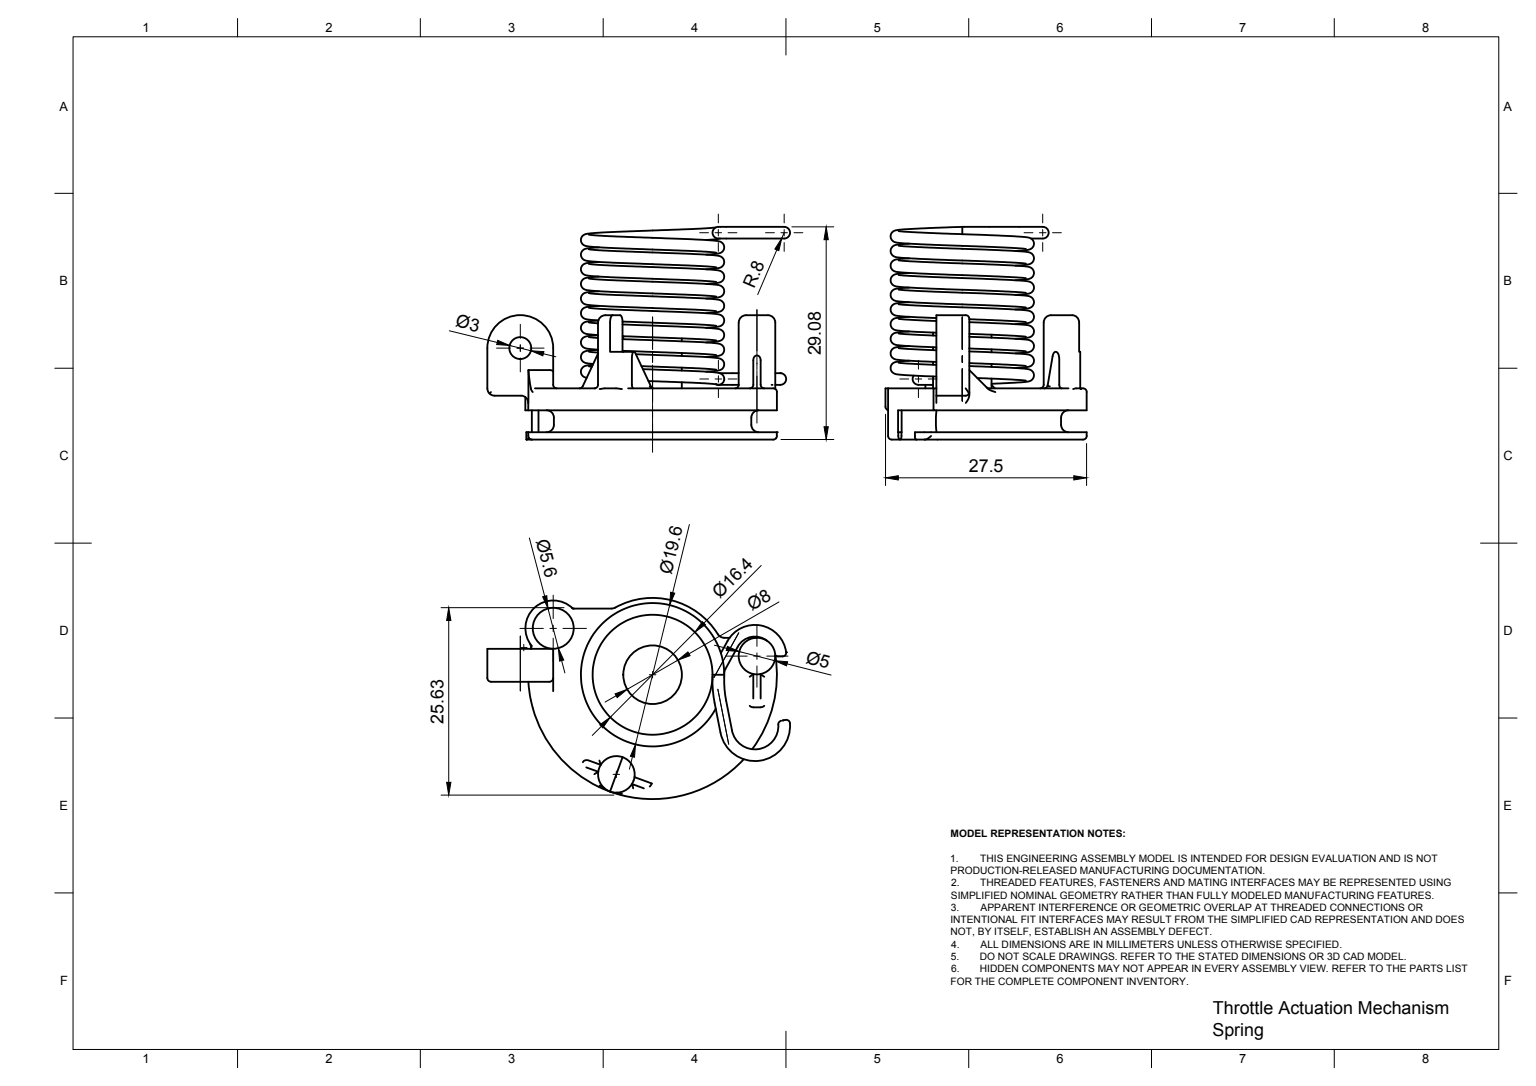
ISO-10303-21;
HEADER;
/* Generated by software containing ST-Developer
 * from STEP Tools, Inc. (www.steptools.com) 
 */

FILE_DESCRIPTION(
/* description */ ('STEP AP214'),
/* implementation_level */ '2;1');

FILE_NAME(
/* name */ 'Throttle Actuation Mechanism Spring.step',
/* time_stamp */ '2026-10-07T12:18:07-07:00',
/* author */ (''),
/* organization */ (''),
/* preprocessor_version */ 'ST-DEVELOPER v20.2',
/* originating_system */ 'Autodesk Translation Framework v15.15.0.0',
/* authorisation */ '');

FILE_SCHEMA (('AUTOMOTIVE_DESIGN { 1 0 10303 214 3 1 1 }'));
ENDSEC;

DATA;
#10=MECHANICAL_DESIGN_GEOMETRIC_PRESENTATION_REPRESENTATION('',(#126),#62974);
#71=(
BOUNDED_CURVE()
B_SPLINE_CURVE(2,(#37611,#37612,#37613,#37614,#37615,#37616,#37617,#37618,
#37619,#37620,#37621,#37622,#37623,#37624,#37625,#37626,#37627,#37628,#37629,
#37630,#37631,#37632,#37633,#37634,#37635,#37636,#37637,#37638,#37639,#37640,
#37641,#37642,#37643,#37644,#37645,#37646,#37647,#37648,#37649,#37650,#37651,
#37652,#37653,#37654,#37655,#37656,#37657,#37658,#37659,#37660,#37661,#37662,
#37663,#37664,#37665,#37666,#37667,#37668,#37669,#37670,#37671,#37672,#37673,
#37674,#37675,#37676,#37677,#37678,#37679,#37680,#37681,#37682,#37683,#37684,
#37685,#37686,#37687,#37688,#37689,#37690,#37691,#37692,#37693,#37694,#37695,
#37696,#37697,#37698,#37699,#37700,#37701,#37702,#37703,#37704,#37705,#37706,
#37707,#37708,#37709,#37710,#37711,#37712,#37713,#37714,#37715,#37716,#37717,
#37718,#37719,#37720,#37721,#37722,#37723,#37724,#37725,#37726,#37727,#37728,
#37729,#37730,#37731),.UNSPECIFIED.,.F.,.F.)
B_SPLINE_CURVE_WITH_KNOTS((3,2,2,2,2,2,2,2,2,2,2,2,2,2,2,2,2,2,2,2,2,2,
2,2,2,2,2,2,2,2,2,2,2,2,2,2,2,2,2,2,2,2,2,2,2,2,2,2,2,2,2,2,2,2,2,2,2,2,
2,2,3),(0.,0.0166666666666666,0.0333333333333333,0.05,0.0666666666666667,
0.0833333333333333,0.1,0.116666666666667,0.133333333333333,0.15,0.166666666666667,
0.183333333333334,0.2,0.216666666666667,0.233333333333334,0.25,0.266666666666667,
0.283333333333334,0.3,0.316666666666666,0.333333333333334,0.35,0.366666666666666,
0.383333333333334,0.4,0.416666666666667,0.433333333333334,0.45,0.466666666666667,
0.483333333333333,0.5,0.516666666666667,0.533333333333333,0.55,0.566666666666667,
0.583333333333333,0.6,0.616666666666667,0.633333333333333,0.65,0.666666666666667,
0.683333333333333,0.7,0.716666666666667,0.733333333333333,0.75,0.766666666666667,
0.783333333333333,0.8,0.816666666666667,0.833333333333333,0.85,0.866666666666667,
0.883333333333333,0.9,0.916666666666667,0.933333333333333,0.95,0.966666666666667,
0.983333333333333,1.),.UNSPECIFIED.)
CURVE()
GEOMETRIC_REPRESENTATION_ITEM()
RATIONAL_B_SPLINE_CURVE((1.,0.866025403784439,1.,0.866025403784439,1.,0.866025403784439,
1.,0.866025403784439,1.,0.866025403784439,1.,0.866025403784439,1.,0.866025403784439,
1.,0.866025403784439,1.,0.866025403784439,1.,0.866025403784439,1.,0.866025403784439,
1.,0.866025403784439,1.,0.866025403784439,1.,0.866025403784439,1.,0.866025403784439,
1.,0.866025403784439,1.,0.866025403784439,1.,0.866025403784439,1.,0.866025403784439,
1.,0.866025403784439,1.,0.866025403784439,1.,0.866025403784439,1.,0.866025403784439,
1.,0.866025403784439,1.,0.866025403784439,1.,0.866025403784439,1.,0.866025403784439,
1.,0.866025403784439,1.,0.866025403784439,1.,0.866025403784439,1.,0.866025403784439,
1.,0.866025403784439,1.,0.866025403784439,1.,0.866025403784439,1.,0.866025403784439,
1.,0.866025403784439,1.,0.866025403784439,1.,0.866025403784439,1.,0.866025403784439,
1.,0.866025403784439,1.,0.866025403784439,1.,0.866025403784439,1.,0.866025403784439,
1.,0.866025403784439,1.,0.866025403784439,1.,0.866025403784439,1.,0.866025403784439,
1.,0.866025403784439,1.,0.866025403784439,1.,0.866025403784439,1.,0.866025403784439,
1.,0.866025403784439,1.,0.866025403784439,1.,0.866025403784439,1.,0.866025403784439,
1.,0.866025403784439,1.,0.866025403784439,1.,0.866025403784439,1.,0.866025403784439,
1.,0.866025403784439,1.))
REPRESENTATION_ITEM('')
);
#72=(
BOUNDED_CURVE()
B_SPLINE_CURVE(2,(#37732,#37733,#37734,#37735,#37736,#37737,#37738,#37739,
#37740,#37741,#37742,#37743,#37744,#37745,#37746,#37747,#37748,#37749,#37750,
#37751,#37752,#37753,#37754,#37755,#37756,#37757,#37758,#37759,#37760,#37761,
#37762,#37763,#37764,#37765,#37766,#37767,#37768,#37769,#37770,#37771,#37772,
#37773,#37774,#37775,#37776,#37777,#37778,#37779,#37780,#37781,#37782,#37783,
#37784,#37785,#37786,#37787,#37788,#37789,#37790,#37791,#37792,#37793,#37794,
#37795,#37796,#37797,#37798,#37799,#37800,#37801,#37802,#37803,#37804,#37805,
#37806,#37807,#37808,#37809,#37810,#37811,#37812,#37813,#37814,#37815,#37816,
#37817,#37818,#37819,#37820,#37821,#37822,#37823,#37824,#37825,#37826,#37827,
#37828,#37829,#37830,#37831,#37832,#37833,#37834,#37835,#37836,#37837,#37838,
#37839,#37840,#37841,#37842,#37843,#37844,#37845,#37846,#37847,#37848,#37849,
#37850,#37851,#37852),.UNSPECIFIED.,.F.,.F.)
B_SPLINE_CURVE_WITH_KNOTS((3,2,2,2,2,2,2,2,2,2,2,2,2,2,2,2,2,2,2,2,2,2,
2,2,2,2,2,2,2,2,2,2,2,2,2,2,2,2,2,2,2,2,2,2,2,2,2,2,2,2,2,2,2,2,2,2,2,2,
2,2,3),(0.,0.0166666666666666,0.0333333333333333,0.05,0.0666666666666667,
0.0833333333333333,0.1,0.116666666666667,0.133333333333333,0.15,0.166666666666667,
0.183333333333334,0.2,0.216666666666667,0.233333333333334,0.25,0.266666666666667,
0.283333333333334,0.3,0.316666666666666,0.333333333333334,0.35,0.366666666666666,
0.383333333333334,0.4,0.416666666666667,0.433333333333334,0.45,0.466666666666667,
0.483333333333333,0.5,0.516666666666667,0.533333333333333,0.55,0.566666666666667,
0.583333333333333,0.6,0.616666666666667,0.633333333333333,0.65,0.666666666666667,
0.683333333333333,0.7,0.716666666666667,0.733333333333333,0.75,0.766666666666667,
0.783333333333333,0.8,0.816666666666667,0.833333333333333,0.85,0.866666666666667,
0.883333333333333,0.9,0.916666666666667,0.933333333333333,0.95,0.966666666666667,
0.983333333333333,1.),.UNSPECIFIED.)
CURVE()
GEOMETRIC_REPRESENTATION_ITEM()
RATIONAL_B_SPLINE_CURVE((1.,0.866025403784439,1.,0.866025403784439,1.,0.866025403784439,
1.,0.866025403784439,1.,0.866025403784439,1.,0.866025403784439,1.,0.866025403784439,
1.,0.866025403784439,1.,0.866025403784439,1.,0.866025403784439,1.,0.866025403784439,
1.,0.866025403784439,1.,0.866025403784439,1.,0.866025403784439,1.,0.866025403784439,
1.,0.866025403784439,1.,0.866025403784439,1.,0.866025403784439,1.,0.866025403784439,
1.,0.866025403784439,1.,0.866025403784439,1.,0.866025403784439,1.,0.866025403784439,
1.,0.866025403784439,1.,0.866025403784439,1.,0.866025403784439,1.,0.866025403784439,
1.,0.866025403784439,1.,0.866025403784439,1.,0.866025403784439,1.,0.866025403784439,
1.,0.866025403784439,1.,0.866025403784439,1.,0.866025403784439,1.,0.866025403784439,
1.,0.866025403784439,1.,0.866025403784439,1.,0.866025403784439,1.,0.866025403784439,
1.,0.866025403784439,1.,0.866025403784439,1.,0.866025403784439,1.,0.866025403784439,
1.,0.866025403784439,1.,0.866025403784439,1.,0.866025403784439,1.,0.866025403784439,
1.,0.866025403784439,1.,0.866025403784439,1.,0.866025403784439,1.,0.866025403784439,
1.,0.866025403784439,1.,0.866025403784439,1.,0.866025403784439,1.,0.866025403784439,
1.,0.866025403784439,1.,0.866025403784439,1.,0.866025403784439,1.,0.866025403784439,
1.,0.866025403784439,1.))
REPRESENTATION_ITEM('')
);
#102=SHAPE_REPRESENTATION_RELATIONSHIP('SRR','None',#63025,#114);
#114=ADVANCED_BREP_SHAPE_REPRESENTATION('',(#138),#62966);
#126=STYLED_ITEM('',(#63090),#138);
#138=MANIFOLD_SOLID_BREP('Body1',#15196);
#149=(
BOUNDED_SURFACE()
B_SPLINE_SURFACE(3,2,((#36764,#36765,#36766,#36767,#36768,#36769,#36770,
#36771,#36772,#36773,#36774,#36775,#36776,#36777,#36778,#36779,#36780,#36781,
#36782,#36783,#36784,#36785,#36786,#36787,#36788,#36789,#36790,#36791,#36792,
#36793,#36794,#36795,#36796,#36797,#36798,#36799,#36800,#36801,#36802,#36803,
#36804,#36805,#36806,#36807,#36808,#36809,#36810,#36811,#36812,#36813,#36814,
#36815,#36816,#36817,#36818,#36819,#36820,#36821,#36822,#36823,#36824,#36825,
#36826,#36827,#36828,#36829,#36830,#36831,#36832,#36833,#36834,#36835,#36836,
#36837,#36838,#36839,#36840,#36841,#36842,#36843,#36844,#36845,#36846,#36847,
#36848,#36849,#36850,#36851,#36852,#36853,#36854,#36855,#36856,#36857,#36858,
#36859,#36860,#36861,#36862,#36863,#36864,#36865,#36866,#36867,#36868,#36869,
#36870,#36871,#36872,#36873,#36874,#36875,#36876,#36877,#36878,#36879,#36880,
#36881,#36882,#36883,#36884),(#36885,#36886,#36887,#36888,#36889,#36890,
#36891,#36892,#36893,#36894,#36895,#36896,#36897,#36898,#36899,#36900,#36901,
#36902,#36903,#36904,#36905,#36906,#36907,#36908,#36909,#36910,#36911,#36912,
#36913,#36914,#36915,#36916,#36917,#36918,#36919,#36920,#36921,#36922,#36923,
#36924,#36925,#36926,#36927,#36928,#36929,#36930,#36931,#36932,#36933,#36934,
#36935,#36936,#36937,#36938,#36939,#36940,#36941,#36942,#36943,#36944,#36945,
#36946,#36947,#36948,#36949,#36950,#36951,#36952,#36953,#36954,#36955,#36956,
#36957,#36958,#36959,#36960,#36961,#36962,#36963,#36964,#36965,#36966,#36967,
#36968,#36969,#36970,#36971,#36972,#36973,#36974,#36975,#36976,#36977,#36978,
#36979,#36980,#36981,#36982,#36983,#36984,#36985,#36986,#36987,#36988,#36989,
#36990,#36991,#36992,#36993,#36994,#36995,#36996,#36997,#36998,#36999,#37000,
#37001,#37002,#37003,#37004,#37005),(#37006,#37007,#37008,#37009,#37010,
#37011,#37012,#37013,#37014,#37015,#37016,#37017,#37018,#37019,#37020,#37021,
#37022,#37023,#37024,#37025,#37026,#37027,#37028,#37029,#37030,#37031,#37032,
#37033,#37034,#37035,#37036,#37037,#37038,#37039,#37040,#37041,#37042,#37043,
#37044,#37045,#37046,#37047,#37048,#37049,#37050,#37051,#37052,#37053,#37054,
#37055,#37056,#37057,#37058,#37059,#37060,#37061,#37062,#37063,#37064,#37065,
#37066,#37067,#37068,#37069,#37070,#37071,#37072,#37073,#37074,#37075,#37076,
#37077,#37078,#37079,#37080,#37081,#37082,#37083,#37084,#37085,#37086,#37087,
#37088,#37089,#37090,#37091,#37092,#37093,#37094,#37095,#37096,#37097,#37098,
#37099,#37100,#37101,#37102,#37103,#37104,#37105,#37106,#37107,#37108,#37109,
#37110,#37111,#37112,#37113,#37114,#37115,#37116,#37117,#37118,#37119,#37120,
#37121,#37122,#37123,#37124,#37125,#37126),(#37127,#37128,#37129,#37130,
#37131,#37132,#37133,#37134,#37135,#37136,#37137,#37138,#37139,#37140,#37141,
#37142,#37143,#37144,#37145,#37146,#37147,#37148,#37149,#37150,#37151,#37152,
#37153,#37154,#37155,#37156,#37157,#37158,#37159,#37160,#37161,#37162,#37163,
#37164,#37165,#37166,#37167,#37168,#37169,#37170,#37171,#37172,#37173,#37174,
#37175,#37176,#37177,#37178,#37179,#37180,#37181,#37182,#37183,#37184,#37185,
#37186,#37187,#37188,#37189,#37190,#37191,#37192,#37193,#37194,#37195,#37196,
#37197,#37198,#37199,#37200,#37201,#37202,#37203,#37204,#37205,#37206,#37207,
#37208,#37209,#37210,#37211,#37212,#37213,#37214,#37215,#37216,#37217,#37218,
#37219,#37220,#37221,#37222,#37223,#37224,#37225,#37226,#37227,#37228,#37229,
#37230,#37231,#37232,#37233,#37234,#37235,#37236,#37237,#37238,#37239,#37240,
#37241,#37242,#37243,#37244,#37245,#37246,#37247),(#37248,#37249,#37250,
#37251,#37252,#37253,#37254,#37255,#37256,#37257,#37258,#37259,#37260,#37261,
#37262,#37263,#37264,#37265,#37266,#37267,#37268,#37269,#37270,#37271,#37272,
#37273,#37274,#37275,#37276,#37277,#37278,#37279,#37280,#37281,#37282,#37283,
#37284,#37285,#37286,#37287,#37288,#37289,#37290,#37291,#37292,#37293,#37294,
#37295,#37296,#37297,#37298,#37299,#37300,#37301,#37302,#37303,#37304,#37305,
#37306,#37307,#37308,#37309,#37310,#37311,#37312,#37313,#37314,#37315,#37316,
#37317,#37318,#37319,#37320,#37321,#37322,#37323,#37324,#37325,#37326,#37327,
#37328,#37329,#37330,#37331,#37332,#37333,#37334,#37335,#37336,#37337,#37338,
#37339,#37340,#37341,#37342,#37343,#37344,#37345,#37346,#37347,#37348,#37349,
#37350,#37351,#37352,#37353,#37354,#37355,#37356,#37357,#37358,#37359,#37360,
#37361,#37362,#37363,#37364,#37365,#37366,#37367,#37368),(#37369,#37370,
#37371,#37372,#37373,#37374,#37375,#37376,#37377,#37378,#37379,#37380,#37381,
#37382,#37383,#37384,#37385,#37386,#37387,#37388,#37389,#37390,#37391,#37392,
#37393,#37394,#37395,#37396,#37397,#37398,#37399,#37400,#37401,#37402,#37403,
#37404,#37405,#37406,#37407,#37408,#37409,#37410,#37411,#37412,#37413,#37414,
#37415,#37416,#37417,#37418,#37419,#37420,#37421,#37422,#37423,#37424,#37425,
#37426,#37427,#37428,#37429,#37430,#37431,#37432,#37433,#37434,#37435,#37436,
#37437,#37438,#37439,#37440,#37441,#37442,#37443,#37444,#37445,#37446,#37447,
#37448,#37449,#37450,#37451,#37452,#37453,#37454,#37455,#37456,#37457,#37458,
#37459,#37460,#37461,#37462,#37463,#37464,#37465,#37466,#37467,#37468,#37469,
#37470,#37471,#37472,#37473,#37474,#37475,#37476,#37477,#37478,#37479,#37480,
#37481,#37482,#37483,#37484,#37485,#37486,#37487,#37488,#37489),(#37490,
#37491,#37492,#37493,#37494,#37495,#37496,#37497,#37498,#37499,#37500,#37501,
#37502,#37503,#37504,#37505,#37506,#37507,#37508,#37509,#37510,#37511,#37512,
#37513,#37514,#37515,#37516,#37517,#37518,#37519,#37520,#37521,#37522,#37523,
#37524,#37525,#37526,#37527,#37528,#37529,#37530,#37531,#37532,#37533,#37534,
#37535,#37536,#37537,#37538,#37539,#37540,#37541,#37542,#37543,#37544,#37545,
#37546,#37547,#37548,#37549,#37550,#37551,#37552,#37553,#37554,#37555,#37556,
#37557,#37558,#37559,#37560,#37561,#37562,#37563,#37564,#37565,#37566,#37567,
#37568,#37569,#37570,#37571,#37572,#37573,#37574,#37575,#37576,#37577,#37578,
#37579,#37580,#37581,#37582,#37583,#37584,#37585,#37586,#37587,#37588,#37589,
#37590,#37591,#37592,#37593,#37594,#37595,#37596,#37597,#37598,#37599,#37600,
#37601,#37602,#37603,#37604,#37605,#37606,#37607,#37608,#37609,#37610)),
 .UNSPECIFIED.,.T.,.F.,.F.)
B_SPLINE_SURFACE_WITH_KNOTS((4,3,4),(3,2,2,2,2,2,2,2,2,2,2,2,2,2,2,2,2,
2,2,2,2,2,2,2,2,2,2,2,2,2,2,2,2,2,2,2,2,2,2,2,2,2,2,2,2,2,2,2,2,2,2,2,2,
2,2,2,2,2,2,2,3),(0.,0.5,1.),(0.,0.0166666666666666,0.0333333333333333,
0.05,0.0666666666666667,0.0833333333333333,0.1,0.116666666666667,0.133333333333333,
0.15,0.166666666666667,0.183333333333334,0.2,0.216666666666667,0.233333333333334,
0.25,0.266666666666667,0.283333333333334,0.3,0.316666666666666,0.333333333333334,
0.35,0.366666666666666,0.383333333333334,0.4,0.416666666666667,0.433333333333334,
0.45,0.466666666666667,0.483333333333333,0.5,0.516666666666667,0.533333333333333,
0.55,0.566666666666667,0.583333333333333,0.6,0.616666666666667,0.633333333333333,
0.65,0.666666666666667,0.683333333333333,0.7,0.716666666666667,0.733333333333333,
0.75,0.766666666666667,0.783333333333333,0.8,0.816666666666667,0.833333333333333,
0.85,0.866666666666667,0.883333333333333,0.9,0.916666666666667,0.933333333333333,
0.95,0.966666666666667,0.983333333333333,1.),.UNSPECIFIED.)
GEOMETRIC_REPRESENTATION_ITEM()
RATIONAL_B_SPLINE_SURFACE(((1.,0.866025403784439,1.,0.866025403784439,1.,
0.866025403784439,1.,0.866025403784439,1.,0.866025403784439,1.,0.866025403784439,
1.,0.866025403784439,1.,0.866025403784439,1.,0.866025403784439,1.,0.866025403784439,
1.,0.866025403784439,1.,0.866025403784439,1.,0.866025403784439,1.,0.866025403784439,
1.,0.866025403784439,1.,0.866025403784439,1.,0.866025403784439,1.,0.866025403784439,
1.,0.866025403784439,1.,0.866025403784439,1.,0.866025403784439,1.,0.866025403784439,
1.,0.866025403784439,1.,0.866025403784439,1.,0.866025403784439,1.,0.866025403784439,
1.,0.866025403784439,1.,0.866025403784439,1.,0.866025403784439,1.,0.866025403784439,
1.,0.866025403784439,1.,0.866025403784439,1.,0.866025403784439,1.,0.866025403784439,
1.,0.866025403784439,1.,0.866025403784439,1.,0.866025403784439,1.,0.866025403784439,
1.,0.866025403784439,1.,0.866025403784439,1.,0.866025403784439,1.,0.866025403784439,
1.,0.866025403784439,1.,0.866025403784439,1.,0.866025403784439,1.,0.866025403784439,
1.,0.866025403784439,1.,0.866025403784439,1.,0.866025403784439,1.,0.866025403784439,
1.,0.866025403784439,1.,0.866025403784439,1.,0.866025403784439,1.,0.866025403784439,
1.,0.866025403784439,1.,0.866025403784439,1.,0.866025403784439,1.,0.866025403784439,
1.,0.866025403784439,1.,0.866025403784439,1.),(0.333333333333334,0.288675134594813,
0.333333333333334,0.288675134594813,0.333333333333334,0.288675134594813,
0.333333333333334,0.288675134594813,0.333333333333334,0.288675134594813,
0.333333333333334,0.288675134594813,0.333333333333334,0.288675134594813,
0.333333333333334,0.288675134594813,0.333333333333334,0.288675134594813,
0.333333333333334,0.288675134594813,0.333333333333334,0.288675134594813,
0.333333333333334,0.288675134594813,0.333333333333334,0.288675134594813,
0.333333333333334,0.288675134594813,0.333333333333334,0.288675134594813,
0.333333333333334,0.288675134594813,0.333333333333334,0.288675134594813,
0.333333333333334,0.288675134594813,0.333333333333334,0.288675134594813,
0.333333333333334,0.288675134594813,0.333333333333334,0.288675134594813,
0.333333333333334,0.288675134594813,0.333333333333334,0.288675134594813,
0.333333333333334,0.288675134594813,0.333333333333334,0.288675134594813,
0.333333333333334,0.288675134594813,0.333333333333334,0.288675134594813,
0.333333333333334,0.288675134594813,0.333333333333334,0.288675134594813,
0.333333333333334,0.288675134594813,0.333333333333334,0.288675134594813,
0.333333333333334,0.288675134594813,0.333333333333334,0.288675134594813,
0.333333333333334,0.288675134594813,0.333333333333334,0.288675134594813,
0.333333333333334,0.288675134594813,0.333333333333334,0.288675134594813,
0.333333333333334,0.288675134594813,0.333333333333334,0.288675134594813,
0.333333333333334,0.288675134594813,0.333333333333334,0.288675134594813,
0.333333333333334,0.288675134594813,0.333333333333334,0.288675134594813,
0.333333333333334,0.288675134594813,0.333333333333334,0.288675134594813,
0.333333333333334,0.288675134594813,0.333333333333334,0.288675134594813,
0.333333333333334,0.288675134594813,0.333333333333334,0.288675134594813,
0.333333333333334,0.288675134594813,0.333333333333334,0.288675134594813,
0.333333333333334,0.288675134594813,0.333333333333334,0.288675134594813,
0.333333333333334,0.288675134594813,0.333333333333334,0.288675134594813,
0.333333333333334,0.288675134594813,0.333333333333334,0.288675134594813,
0.333333333333334,0.288675134594813,0.333333333333334,0.288675134594813,
0.333333333333334,0.288675134594813,0.333333333333334),(0.333333333333334,
0.288675134594813,0.333333333333334,0.288675134594813,0.333333333333334,
0.288675134594813,0.333333333333334,0.288675134594813,0.333333333333334,
0.288675134594813,0.333333333333334,0.288675134594813,0.333333333333334,
0.288675134594813,0.333333333333334,0.288675134594813,0.333333333333334,
0.288675134594813,0.333333333333334,0.288675134594813,0.333333333333334,
0.288675134594813,0.333333333333334,0.288675134594813,0.333333333333334,
0.288675134594813,0.333333333333334,0.288675134594813,0.333333333333334,
0.288675134594813,0.333333333333334,0.288675134594813,0.333333333333334,
0.288675134594813,0.333333333333334,0.288675134594813,0.333333333333334,
0.288675134594813,0.333333333333334,0.288675134594813,0.333333333333334,
0.288675134594813,0.333333333333334,0.288675134594813,0.333333333333334,
0.288675134594813,0.333333333333334,0.288675134594813,0.333333333333334,
0.288675134594813,0.333333333333334,0.288675134594813,0.333333333333334,
0.288675134594813,0.333333333333334,0.288675134594813,0.333333333333334,
0.288675134594813,0.333333333333334,0.288675134594813,0.333333333333334,
0.288675134594813,0.333333333333334,0.288675134594813,0.333333333333334,
0.288675134594813,0.333333333333334,0.288675134594813,0.333333333333334,
0.288675134594813,0.333333333333334,0.288675134594813,0.333333333333334,
0.288675134594813,0.333333333333334,0.288675134594813,0.333333333333334,
0.288675134594813,0.333333333333334,0.288675134594813,0.333333333333334,
0.288675134594813,0.333333333333334,0.288675134594813,0.333333333333334,
0.288675134594813,0.333333333333334,0.288675134594813,0.333333333333334,
0.288675134594813,0.333333333333334,0.288675134594813,0.333333333333334,
0.288675134594813,0.333333333333334,0.288675134594813,0.333333333333334,
0.288675134594813,0.333333333333334,0.288675134594813,0.333333333333334,
0.288675134594813,0.333333333333334,0.288675134594813,0.333333333333334,
0.288675134594813,0.333333333333334,0.288675134594813,0.333333333333334,
0.288675134594813,0.333333333333334,0.288675134594813,0.333333333333334,
0.288675134594813,0.333333333333334,0.288675134594813,0.333333333333334,
0.288675134594813,0.333333333333334,0.288675134594813,0.333333333333334),
(1.,0.866025403784439,1.,0.866025403784439,1.,0.866025403784439,1.,0.866025403784439,
1.,0.866025403784439,1.,0.866025403784439,1.,0.866025403784439,1.,0.866025403784439,
1.,0.866025403784439,1.,0.866025403784439,1.,0.866025403784439,1.,0.866025403784439,
1.,0.866025403784439,1.,0.866025403784439,1.,0.866025403784439,1.,0.866025403784439,
1.,0.866025403784439,1.,0.866025403784439,1.,0.866025403784439,1.,0.866025403784439,
1.,0.866025403784439,1.,0.866025403784439,1.,0.866025403784439,1.,0.866025403784439,
1.,0.866025403784439,1.,0.866025403784439,1.,0.866025403784439,1.,0.866025403784439,
1.,0.866025403784439,1.,0.866025403784439,1.,0.866025403784439,1.,0.866025403784439,
1.,0.866025403784439,1.,0.866025403784439,1.,0.866025403784439,1.,0.866025403784439,
1.,0.866025403784439,1.,0.866025403784439,1.,0.866025403784439,1.,0.866025403784439,
1.,0.866025403784439,1.,0.866025403784439,1.,0.866025403784439,1.,0.866025403784439,
1.,0.866025403784439,1.,0.866025403784439,1.,0.866025403784439,1.,0.866025403784439,
1.,0.866025403784439,1.,0.866025403784439,1.,0.866025403784439,1.,0.866025403784439,
1.,0.866025403784439,1.,0.866025403784439,1.,0.866025403784439,1.,0.866025403784439,
1.,0.866025403784439,1.,0.866025403784439,1.,0.866025403784439,1.,0.866025403784439,
1.),(0.333333333333334,0.288675134594813,0.333333333333334,0.288675134594813,
0.333333333333334,0.288675134594813,0.333333333333334,0.288675134594813,
0.333333333333334,0.288675134594813,0.333333333333334,0.288675134594813,
0.333333333333334,0.288675134594813,0.333333333333334,0.288675134594813,
0.333333333333334,0.288675134594813,0.333333333333334,0.288675134594813,
0.333333333333334,0.288675134594813,0.333333333333334,0.288675134594813,
0.333333333333334,0.288675134594813,0.333333333333334,0.288675134594813,
0.333333333333334,0.288675134594813,0.333333333333334,0.288675134594813,
0.333333333333334,0.288675134594813,0.333333333333334,0.288675134594813,
0.333333333333334,0.288675134594813,0.333333333333334,0.288675134594813,
0.333333333333334,0.288675134594813,0.333333333333334,0.288675134594813,
0.333333333333334,0.288675134594813,0.333333333333334,0.288675134594813,
0.333333333333334,0.288675134594813,0.333333333333334,0.288675134594813,
0.333333333333334,0.288675134594813,0.333333333333334,0.288675134594813,
0.333333333333334,0.288675134594813,0.333333333333334,0.288675134594813,
0.333333333333334,0.288675134594813,0.333333333333334,0.288675134594813,
0.333333333333334,0.288675134594813,0.333333333333334,0.288675134594813,
0.333333333333334,0.288675134594813,0.333333333333334,0.288675134594813,
0.333333333333334,0.288675134594813,0.333333333333334,0.288675134594813,
0.333333333333334,0.288675134594813,0.333333333333334,0.288675134594813,
0.333333333333334,0.288675134594813,0.333333333333334,0.288675134594813,
0.333333333333334,0.288675134594813,0.333333333333334,0.288675134594813,
0.333333333333334,0.288675134594813,0.333333333333334,0.288675134594813,
0.333333333333334,0.288675134594813,0.333333333333334,0.288675134594813,
0.333333333333334,0.288675134594813,0.333333333333334,0.288675134594813,
0.333333333333334,0.288675134594813,0.333333333333334,0.288675134594813,
0.333333333333334,0.288675134594813,0.333333333333334,0.288675134594813,
0.333333333333334,0.288675134594813,0.333333333333334,0.288675134594813,
0.333333333333334,0.288675134594813,0.333333333333334,0.288675134594813,
0.333333333333334,0.288675134594813,0.333333333333334,0.288675134594813,
0.333333333333334),(0.333333333333334,0.288675134594813,0.333333333333334,
0.288675134594813,0.333333333333334,0.288675134594813,0.333333333333334,
0.288675134594813,0.333333333333334,0.288675134594813,0.333333333333334,
0.288675134594813,0.333333333333334,0.288675134594813,0.333333333333334,
0.288675134594813,0.333333333333334,0.288675134594813,0.333333333333334,
0.288675134594813,0.333333333333334,0.288675134594813,0.333333333333334,
0.288675134594813,0.333333333333334,0.288675134594813,0.333333333333334,
0.288675134594813,0.333333333333334,0.288675134594813,0.333333333333334,
0.288675134594813,0.333333333333334,0.288675134594813,0.333333333333334,
0.288675134594813,0.333333333333334,0.288675134594813,0.333333333333334,
0.288675134594813,0.333333333333334,0.288675134594813,0.333333333333334,
0.288675134594813,0.333333333333334,0.288675134594813,0.333333333333334,
0.288675134594813,0.333333333333334,0.288675134594813,0.333333333333334,
0.288675134594813,0.333333333333334,0.288675134594813,0.333333333333334,
0.288675134594813,0.333333333333334,0.288675134594813,0.333333333333334,
0.288675134594813,0.333333333333334,0.288675134594813,0.333333333333334,
0.288675134594813,0.333333333333334,0.288675134594813,0.333333333333334,
0.288675134594813,0.333333333333334,0.288675134594813,0.333333333333334,
0.288675134594813,0.333333333333334,0.288675134594813,0.333333333333334,
0.288675134594813,0.333333333333334,0.288675134594813,0.333333333333334,
0.288675134594813,0.333333333333334,0.288675134594813,0.333333333333334,
0.288675134594813,0.333333333333334,0.288675134594813,0.333333333333334,
0.288675134594813,0.333333333333334,0.288675134594813,0.333333333333334,
0.288675134594813,0.333333333333334,0.288675134594813,0.333333333333334,
0.288675134594813,0.333333333333334,0.288675134594813,0.333333333333334,
0.288675134594813,0.333333333333334,0.288675134594813,0.333333333333334,
0.288675134594813,0.333333333333334,0.288675134594813,0.333333333333334,
0.288675134594813,0.333333333333334,0.288675134594813,0.333333333333334,
0.288675134594813,0.333333333333334,0.288675134594813,0.333333333333334,
0.288675134594813,0.333333333333334,0.288675134594813,0.333333333333334,
0.288675134594813,0.333333333333334),(1.,0.866025403784439,1.,0.866025403784439,
1.,0.866025403784439,1.,0.866025403784439,1.,0.866025403784439,1.,0.866025403784439,
1.,0.866025403784439,1.,0.866025403784439,1.,0.866025403784439,1.,0.866025403784439,
1.,0.866025403784439,1.,0.866025403784439,1.,0.866025403784439,1.,0.866025403784439,
1.,0.866025403784439,1.,0.866025403784439,1.,0.866025403784439,1.,0.866025403784439,
1.,0.866025403784439,1.,0.866025403784439,1.,0.866025403784439,1.,0.866025403784439,
1.,0.866025403784439,1.,0.866025403784439,1.,0.866025403784439,1.,0.866025403784439,
1.,0.866025403784439,1.,0.866025403784439,1.,0.866025403784439,1.,0.866025403784439,
1.,0.866025403784439,1.,0.866025403784439,1.,0.866025403784439,1.,0.866025403784439,
1.,0.866025403784439,1.,0.866025403784439,1.,0.866025403784439,1.,0.866025403784439,
1.,0.866025403784439,1.,0.866025403784439,1.,0.866025403784439,1.,0.866025403784439,
1.,0.866025403784439,1.,0.866025403784439,1.,0.866025403784439,1.,0.866025403784439,
1.,0.866025403784439,1.,0.866025403784439,1.,0.866025403784439,1.,0.866025403784439,
1.,0.866025403784439,1.,0.866025403784439,1.,0.866025403784439,1.,0.866025403784439,
1.,0.866025403784439,1.,0.866025403784439,1.,0.866025403784439,1.,0.866025403784439,
1.,0.866025403784439,1.,0.866025403784439,1.)))
REPRESENTATION_ITEM('')
SURFACE()
);
#150=(
BOUNDED_SURFACE()
B_SPLINE_SURFACE(3,2,((#37853,#37854,#37855),(#37856,#37857,#37858),(#37859,
#37860,#37861),(#37862,#37863,#37864),(#37865,#37866,#37867),(#37868,#37869,
#37870),(#37871,#37872,#37873),(#37874,#37875,#37876),(#37877,#37878,#37879),
(#37880,#37881,#37882),(#37883,#37884,#37885),(#37886,#37887,#37888),(#37889,
#37890,#37891),(#37892,#37893,#37894),(#37895,#37896,#37897),(#37898,#37899,
#37900),(#37901,#37902,#37903),(#37904,#37905,#37906),(#37907,#37908,#37909),
(#37910,#37911,#37912),(#37913,#37914,#37915),(#37916,#37917,#37918),(#37919,
#37920,#37921),(#37922,#37923,#37924),(#37925,#37926,#37927),(#37928,#37929,
#37930),(#37931,#37932,#37933),(#37934,#37935,#37936),(#37937,#37938,#37939),
(#37940,#37941,#37942),(#37943,#37944,#37945),(#37946,#37947,#37948),(#37949,
#37950,#37951),(#37952,#37953,#37954),(#37955,#37956,#37957),(#37958,#37959,
#37960),(#37961,#37962,#37963),(#37964,#37965,#37966),(#37967,#37968,#37969),
(#37970,#37971,#37972),(#37973,#37974,#37975),(#37976,#37977,#37978),(#37979,
#37980,#37981),(#37982,#37983,#37984),(#37985,#37986,#37987),(#37988,#37989,
#37990),(#37991,#37992,#37993),(#37994,#37995,#37996),(#37997,#37998,#37999),
(#38000,#38001,#38002),(#38003,#38004,#38005),(#38006,#38007,#38008),(#38009,
#38010,#38011),(#38012,#38013,#38014),(#38015,#38016,#38017),(#38018,#38019,
#38020),(#38021,#38022,#38023),(#38024,#38025,#38026),(#38027,#38028,#38029),
(#38030,#38031,#38032),(#38033,#38034,#38035),(#38036,#38037,#38038),(#38039,
#38040,#38041),(#38042,#38043,#38044),(#38045,#38046,#38047),(#38048,#38049,
#38050),(#38051,#38052,#38053),(#38054,#38055,#38056),(#38057,#38058,#38059),
(#38060,#38061,#38062),(#38063,#38064,#38065),(#38066,#38067,#38068),(#38069,
#38070,#38071),(#38072,#38073,#38074),(#38075,#38076,#38077),(#38078,#38079,
#38080),(#38081,#38082,#38083),(#38084,#38085,#38086),(#38087,#38088,#38089),
(#38090,#38091,#38092),(#38093,#38094,#38095),(#38096,#38097,#38098),(#38099,
#38100,#38101),(#38102,#38103,#38104),(#38105,#38106,#38107),(#38108,#38109,
#38110),(#38111,#38112,#38113),(#38114,#38115,#38116),(#38117,#38118,#38119),
(#38120,#38121,#38122),(#38123,#38124,#38125),(#38126,#38127,#38128),(#38129,
#38130,#38131),(#38132,#38133,#38134),(#38135,#38136,#38137),(#38138,#38139,
#38140),(#38141,#38142,#38143),(#38144,#38145,#38146),(#38147,#38148,#38149),
(#38150,#38151,#38152),(#38153,#38154,#38155),(#38156,#38157,#38158),(#38159,
#38160,#38161),(#38162,#38163,#38164),(#38165,#38166,#38167),(#38168,#38169,
#38170),(#38171,#38172,#38173),(#38174,#38175,#38176),(#38177,#38178,#38179),
(#38180,#38181,#38182),(#38183,#38184,#38185),(#38186,#38187,#38188),(#38189,
#38190,#38191),(#38192,#38193,#38194),(#38195,#38196,#38197),(#38198,#38199,
#38200),(#38201,#38202,#38203),(#38204,#38205,#38206),(#38207,#38208,#38209),
(#38210,#38211,#38212),(#38213,#38214,#38215),(#38216,#38217,#38218),(#38219,
#38220,#38221),(#38222,#38223,#38224),(#38225,#38226,#38227),(#38228,#38229,
#38230),(#38231,#38232,#38233),(#38234,#38235,#38236),(#38237,#38238,#38239),
(#38240,#38241,#38242),(#38243,#38244,#38245),(#38246,#38247,#38248),(#38249,
#38250,#38251),(#38252,#38253,#38254),(#38255,#38256,#38257),(#38258,#38259,
#38260),(#38261,#38262,#38263),(#38264,#38265,#38266),(#38267,#38268,#38269),
(#38270,#38271,#38272),(#38273,#38274,#38275),(#38276,#38277,#38278),(#38279,
#38280,#38281),(#38282,#38283,#38284),(#38285,#38286,#38287),(#38288,#38289,
#38290),(#38291,#38292,#38293),(#38294,#38295,#38296)),.UNSPECIFIED.,.T.,
 .F.,.F.)
B_SPLINE_SURFACE_WITH_KNOTS((4,2,2,2,2,2,2,2,2,2,2,2,2,2,2,2,2,2,2,2,2,
2,2,2,2,2,2,2,2,2,2,2,2,2,2,2,2,2,2,2,2,2,2,2,2,2,2,2,2,2,2,2,2,2,2,2,2,
2,2,2,2,2,2,2,2,2,2,2,2,2,2,2,2,4),(3,3),(0.,5.88439546912971E-5,8.82659320369456E-5,
0.00010297692070977,0.000117687909382594,0.000176531864073891,0.000191242852746715,
0.00020595384141954,0.000235375818765188,0.000294219773456485,0.000301575267792897,
0.00030893076212931,0.000323641750802134,0.000353063728147782,0.000382485705493431,
0.000397196694166255,0.000404552188502667,0.000411907682839079,0.000470751637530376,
0.000500173614876025,0.000514884603548849,0.000529595592221674,0.00058843954691297,
0.000603150535585795,0.000617861524258619,0.000647283501604268,0.000706127456295565,
0.000713482950631977,0.000720838444968389,0.000735549433641213,0.000764971410986862,
0.00079439338833251,0.000809104377005334,0.000823815365678159,0.000882659320369456,
0.00089737030904228,0.000912081297715104,0.000941503275060753,0.000970925252406401,
0.000985636241079226,0.00100034722975205,0.00105919118444335,0.00107390217311617,
0.001088613161789,0.00111803513913464,0.00117687909382594,0.00120630107117159,
0.00123572304851724,0.00126514502586289,0.00127985601453571,0.00129456700320854,
0.00135341095789983,0.00136812194657266,0.00138283293524548,0.00141225491259113,
0.00147109886728243,0.00147845436161884,0.00148580985595525,0.00150052084462807,
0.00152994282197372,0.00155936479931937,0.0015740757879922,0.00158878677666502,
0.00164763073135632,0.00167705270870197,0.00168440820303838,0.00169176369737479,
0.00170647468604761,0.00176531864073891,0.00178002962941174,0.00179474061808456,
0.00182416259543021,0.00185358457277586,0.00188300655012151),(0.,1.),
 .UNSPECIFIED.)
GEOMETRIC_REPRESENTATION_ITEM()
RATIONAL_B_SPLINE_SURFACE(((1.,0.715726527571974,1.),(1.,0.712824837312312,
1.),(1.,0.709939183288703,1.),(1.,0.70563780485041,1.),(1.,0.704208324053071,
1.),(1.,0.702070408823295,1.),(1.,0.701358182508267,1.),(1.,0.699938470033913,
1.),(1.,0.699235558344621,1.),(1.,0.695754807328025,1.),(1.,0.693077556893273,
1.),(1.,0.689858407232006,1.),(1.,0.689220997236269,1.),(1.,0.687959045727463,
1.),(1.,0.687333603220981,1.),(1.,0.685482641655898,1.),(1.,0.684295233247551,
1.),(1.,0.680865948622576,1.),(1.,0.678755828779441,1.),(1.,0.676577048170574,
1.),(1.,0.676337696500587,1.),(1.,0.675864499150325,1.),(1.,0.675630328898002,
1.),(1.,0.674939074618547,1.),(1.,0.674493188941281,1.),(1.,0.673199210425328,
1.),(1.,0.672394697221168,1.),(1.,0.670898516819421,1.),(1.,0.67020685543305,
1.),(1.,0.669254011840167,1.),(1.,0.668950530912342,1.),(1.,0.668516758864078,
1.),(1.,0.668375744076451,1.),(1.,0.668100931680429,1.),(1.,0.66796703830326,
1.),(1.,0.666801110120948,1.),(1.,0.666028636022973,1.),(1.,0.665248431462833,
1.),(1.,0.665051947055941,1.),(1.,0.664854970332435,1.),(1.,0.664805603591522,
1.),(1.,0.664740760515236,1.),(1.,0.664725098690157,1.),(1.,0.664729031892036,
1.),(1.,0.664992831063146,1.),(1.,0.665649916349412,1.),(1.,0.665797857858843,
1.),(1.,0.666127492088933,1.),(1.,0.666309421952839,1.),(1.,0.666899952411735,
1.),(1.,0.667354870043226,1.),(1.,0.668899800350139,1.),(1.,0.670168108270442,
1.),(1.,0.671877972859038,1.),(1.,0.672071972172369,1.),(1.,0.672465766634245,
1.),(1.,0.672665825106501,1.),(1.,0.673275414881356,1.),(1.,0.673694356676243,
1.),(1.,0.674988511758639,1.),(1.,0.675900966431535,1.),(1.,0.677825804601594,
1.),(1.,0.678838181026788,1.),(1.,0.680434320387322,1.),(1.,0.680979480786494,
1.),(1.,0.682095794766937,1.),(1.,0.682662909252039,1.),(1.,0.68554058312361,
1.),(1.,0.687978699058213,1.),(1.,0.69120098153353,1.),(1.,0.691854240148126,
1.),(1.,0.693178775224038,1.),(1.,0.693851046877455,1.),(1.,0.695888940711959,
1.),(1.,0.697266250733029,1.),(1.,0.700058726696578,1.),(1.,0.701473890706926,
1.),(1.,0.703625959383263,1.),(1.,0.704345718616287,1.),(1.,0.705783355102051,
1.),(1.,0.706502269097388,1.),(1.,0.71009740810345,1.),(1.,0.712975541569779,
1.),(1.,0.716575141001572,1.),(1.,0.717295144791949,1.),(1.,0.718735249984781,
1.),(1.,0.719451276741359,1.),(1.,0.721578968626909,1.),(1.,0.722973916817993,
1.),(1.,0.727088200171688,1.),(1.,0.729737986565996,1.),(1.,0.733557197223877,
1.),(1.,0.734784504108155,1.),(1.,0.737143649706032,1.),(1.,0.738276364056428,
1.),(1.,0.740446615586834,1.),(1.,0.741484163457107,1.),(1.,0.742965865508942,
1.),(1.,0.743447540320556,1.),(1.,0.744384190268116,1.),(1.,0.744835768417984,
1.),(1.,0.747010115951137,1.),(1.,0.748485471872314,1.),(1.,0.749993321046985,
1.),(1.,0.750277933331016,1.),(1.,0.750812495848506,1.),(1.,0.751062871482513,
1.),(1.,0.751757652067472,1.),(1.,0.752142025968554,1.),(1.,0.753064753379183,
1.),(1.,0.753374703098945,1.),(1.,0.753370274811438,1.),(1.,0.753364836618584,
1.),(1.,0.753343954153974,1.),(1.,0.753328486568168,1.),(1.,0.753267330936153,
1.),(1.,0.753206862795746,1.),(1.,0.752967583346212,1.),(1.,0.752731013298035,
1.),(1.,0.752107006678872,1.),(1.,0.751719566002465,1.),(1.,0.751024658994972,
1.),(1.,0.75077403600156,1.),(1.,0.750234324747068,1.),(1.,0.749944553237197,
1.),(1.,0.748414981448763,1.),(1.,0.746926622748835,1.),(1.,0.744319366838701,
1.),(1.,0.743387383255421,1.),(1.,0.742142765249864,1.),(1.,0.741889533171004,
1.),(1.,0.74137762258562,1.),(1.,0.74111874517533,1.),(1.,0.740333498527515,
1.),(1.,0.739798515633772,1.),(1.,0.737067782822572,1.),(1.,0.73470619863159,
1.),(1.,0.731541347327889,1.),(1.,0.73089763158831,1.),(1.,0.729588498808487,
1.),(1.,0.728926359265131,1.),(1.,0.726927210402846,1.),(1.,0.725573615722195,
1.),(1.,0.722827030199711,1.),(1.,0.721434033464342,1.),(1.,0.718609414473237,
1.),(1.,0.717177372701805,1.),(1.,0.715726527571974,1.)))
REPRESENTATION_ITEM('')
SURFACE()
);
#151=(
BOUNDED_SURFACE()
B_SPLINE_SURFACE(3,2,((#38515,#38516,#38517),(#38518,#38519,#38520),(#38521,
#38522,#38523),(#38524,#38525,#38526),(#38527,#38528,#38529),(#38530,#38531,
#38532),(#38533,#38534,#38535),(#38536,#38537,#38538),(#38539,#38540,#38541),
(#38542,#38543,#38544),(#38545,#38546,#38547),(#38548,#38549,#38550),(#38551,
#38552,#38553),(#38554,#38555,#38556),(#38557,#38558,#38559),(#38560,#38561,
#38562),(#38563,#38564,#38565),(#38566,#38567,#38568),(#38569,#38570,#38571),
(#38572,#38573,#38574),(#38575,#38576,#38577),(#38578,#38579,#38580),(#38581,
#38582,#38583),(#38584,#38585,#38586),(#38587,#38588,#38589),(#38590,#38591,
#38592),(#38593,#38594,#38595),(#38596,#38597,#38598),(#38599,#38600,#38601),
(#38602,#38603,#38604),(#38605,#38606,#38607),(#38608,#38609,#38610),(#38611,
#38612,#38613),(#38614,#38615,#38616),(#38617,#38618,#38619),(#38620,#38621,
#38622),(#38623,#38624,#38625),(#38626,#38627,#38628),(#38629,#38630,#38631),
(#38632,#38633,#38634),(#38635,#38636,#38637),(#38638,#38639,#38640),(#38641,
#38642,#38643),(#38644,#38645,#38646),(#38647,#38648,#38649),(#38650,#38651,
#38652),(#38653,#38654,#38655),(#38656,#38657,#38658),(#38659,#38660,#38661),
(#38662,#38663,#38664),(#38665,#38666,#38667),(#38668,#38669,#38670),(#38671,
#38672,#38673),(#38674,#38675,#38676),(#38677,#38678,#38679),(#38680,#38681,
#38682),(#38683,#38684,#38685),(#38686,#38687,#38688),(#38689,#38690,#38691),
(#38692,#38693,#38694),(#38695,#38696,#38697),(#38698,#38699,#38700),(#38701,
#38702,#38703),(#38704,#38705,#38706),(#38707,#38708,#38709),(#38710,#38711,
#38712),(#38713,#38714,#38715),(#38716,#38717,#38718),(#38719,#38720,#38721),
(#38722,#38723,#38724),(#38725,#38726,#38727),(#38728,#38729,#38730),(#38731,
#38732,#38733),(#38734,#38735,#38736),(#38737,#38738,#38739),(#38740,#38741,
#38742),(#38743,#38744,#38745),(#38746,#38747,#38748),(#38749,#38750,#38751),
(#38752,#38753,#38754),(#38755,#38756,#38757),(#38758,#38759,#38760),(#38761,
#38762,#38763),(#38764,#38765,#38766),(#38767,#38768,#38769),(#38770,#38771,
#38772),(#38773,#38774,#38775),(#38776,#38777,#38778),(#38779,#38780,#38781),
(#38782,#38783,#38784),(#38785,#38786,#38787),(#38788,#38789,#38790),(#38791,
#38792,#38793),(#38794,#38795,#38796),(#38797,#38798,#38799),(#38800,#38801,
#38802),(#38803,#38804,#38805),(#38806,#38807,#38808),(#38809,#38810,#38811),
(#38812,#38813,#38814),(#38815,#38816,#38817),(#38818,#38819,#38820),(#38821,
#38822,#38823),(#38824,#38825,#38826),(#38827,#38828,#38829),(#38830,#38831,
#38832),(#38833,#38834,#38835),(#38836,#38837,#38838),(#38839,#38840,#38841),
(#38842,#38843,#38844),(#38845,#38846,#38847),(#38848,#38849,#38850),(#38851,
#38852,#38853),(#38854,#38855,#38856),(#38857,#38858,#38859),(#38860,#38861,
#38862),(#38863,#38864,#38865),(#38866,#38867,#38868),(#38869,#38870,#38871),
(#38872,#38873,#38874),(#38875,#38876,#38877),(#38878,#38879,#38880),(#38881,
#38882,#38883),(#38884,#38885,#38886),(#38887,#38888,#38889),(#38890,#38891,
#38892),(#38893,#38894,#38895),(#38896,#38897,#38898),(#38899,#38900,#38901),
(#38902,#38903,#38904),(#38905,#38906,#38907),(#38908,#38909,#38910),(#38911,
#38912,#38913),(#38914,#38915,#38916),(#38917,#38918,#38919),(#38920,#38921,
#38922),(#38923,#38924,#38925),(#38926,#38927,#38928),(#38929,#38930,#38931),
(#38932,#38933,#38934),(#38935,#38936,#38937),(#38938,#38939,#38940),(#38941,
#38942,#38943),(#38944,#38945,#38946),(#38947,#38948,#38949),(#38950,#38951,
#38952),(#38953,#38954,#38955),(#38956,#38957,#38958)),.UNSPECIFIED.,.T.,
 .F.,.F.)
B_SPLINE_SURFACE_WITH_KNOTS((4,2,2,2,2,2,2,2,2,2,2,2,2,2,2,2,2,2,2,2,2,
2,2,2,2,2,2,2,2,2,2,2,2,2,2,2,2,2,2,2,2,2,2,2,2,2,2,2,2,2,2,2,2,2,2,2,2,
2,2,2,2,2,2,2,2,2,2,2,2,2,2,2,2,4),(3,3),(0.,2.94572120696205E-5,5.89144241392409E-5,
8.83716362088614E-5,0.000103100242243672,0.000117828848278482,0.000176743272417723,
0.000206200484487343,0.000235657696556964,0.000294572120696205,0.000309300726731015,
0.000324029332765825,0.000353486544835446,0.000382943756905066,0.000397672362939876,
0.000405036665957281,0.000412400968974686,0.000471315393113927,0.000500772605183548,
0.000515501211218358,0.000530229817253168,0.000589144241392409,0.00060387284742722,
0.00061860145346203,0.00064805866553165,0.000706973089670891,0.000721701695705701,
0.000736430301740512,0.000765887513810132,0.000795344725879752,0.000810073331914563,
0.000824801937949373,0.000883716362088614,0.000898444968123424,0.000913173574158234,
0.000942630786227855,0.000972087998297475,0.000986816604332285,0.0010015452103671,
0.00106045963450634,0.00107518824054115,0.00108255254355855,0.00108991684657596,
0.00111937405864558,0.00117828848278482,0.00119301708881963,0.00120774569485444,
0.00123720290692406,0.00126666011899368,0.00128138872502849,0.0012961173310633,
0.00135503175520254,0.00136976036123735,0.00137712466425476,0.00138448896727216,
0.00141394617934178,0.00147286060348102,0.00148758920951583,0.00150231781555064,
0.00153177502762026,0.00156123223968988,0.00157596084572469,0.00159068945175951,
0.00164960387589875,0.00167906108796837,0.00168642539098577,0.00169378969400318,
0.00170851830003799,0.00176743272417723,0.00178216133021204,0.00179688993624685,
0.00182634714831647,0.00185580436038609,0.00188526157245571),(0.,1.),
 .UNSPECIFIED.)
GEOMETRIC_REPRESENTATION_ITEM()
RATIONAL_B_SPLINE_SURFACE(((1.,0.706768250621048,1.),(1.,0.708426298986424,
1.),(1.,0.71008008713948,1.),(1.,0.713376962618569,1.),(1.,0.715020497077106,
1.),(1.,0.718297519423347,1.),(1.,0.719931010200883,1.),(1.,0.722372962983203,
1.),(1.,0.723186044045656,1.),(1.,0.724807250742798,1.),(1.,0.725609732738587,
1.),(1.,0.729581079301821,1.),(1.,0.732629067598119,1.),(1.,0.736998113914005,
1.),(1.,0.738421550016217,1.),(1.,0.741190319959484,1.),(1.,0.742514778054944,
1.),(1.,0.74631005642732,1.),(1.,0.748604628218609,1.),(1.,0.751158032017892,
1.),(1.,0.751653549012408,1.),(1.,0.752608572928937,1.),(1.,0.75306560396881,
1.),(1.,0.754375982622539,1.),(1.,0.755168745312861,1.),(1.,0.756593080986396,
1.),(1.,0.757224656832598,1.),(1.,0.758048217054286,1.),(1.,0.758302072136257,
1.),(1.,0.758651166057736,1.),(1.,0.758762248731274,1.),(1.,0.758973701473796,
1.),(1.,0.759074180129559,1.),(1.,0.75992529243238,1.),(1.,0.760313664756985,
1.),(1.,0.760358379138884,1.),(1.,0.760283061324181,1.),(1.,0.760031210406024,
1.),(1.,0.759923663695399,1.),(1.,0.759664049141739,1.),(1.,0.759511979981949,
1.),(1.,0.758642742016197,1.),(1.,0.757601675913755,1.),(1.,0.755877310483683,
1.),(1.,0.755511111609718,1.),(1.,0.754735567621713,1.),(1.,0.75432615177884,
1.),(1.,0.753047436476538,1.),(1.,0.752123540268788,1.),(1.,0.749147228369339,
1.),(1.,0.746892043597223,1.),(1.,0.743737116871849,1.),(1.,0.743092518946092,
1.),(1.,0.741782460083778,1.),(1.,0.74111613029348,1.),(1.,0.739084256899976,
1.),(1.,0.737685905862985,1.),(1.,0.734804890076589,1.),(1.,0.733322221436288,
1.),(1.,0.731035362741923,1.),(1.,0.730261837049612,1.),(1.,0.728696721731266,
1.),(1.,0.727910041758493,1.),(1.,0.723956994901979,1.),(1.,0.72073248846334,
1.),(1.,0.716630623834303,1.),(1.,0.715806638742097,1.),(1.,0.71415140110213,
1.),(1.,0.713318880580274,1.),(1.,0.710818889674067,1.),(1.,0.709159874596443,
1.),(1.,0.705856827432451,1.),(1.,0.704212795668421,1.),(1.,0.701757740368045,
1.),(1.,0.70094258809021,1.),(1.,0.699329967906212,1.),(1.,0.698530836824196,
1.),(1.,0.694570217898487,1.),(1.,0.691513076412309,1.),(1.,0.68782527710447,
1.),(1.,0.687094446903374,1.),(1.,0.686008340574591,1.),(1.,0.685647981698853,
1.),(1.,0.684934623703741,1.),(1.,0.684581117243663,1.),(1.,0.682829208835022,
1.),(1.,0.681477582738208,1.),(1.,0.677566315979365,1.),(1.,0.675148976138824,
1.),(1.,0.672364992202017,1.),(1.,0.671822976516116,1.),(1.,0.670773369616535,
1.),(1.,0.670264872579329,1.),(1.,0.668787238113039,1.),(1.,0.667865848198686,
1.),(1.,0.666147791049292,1.),(1.,0.665351122681227,1.),(1.,0.664250505737303,
1.),(1.,0.663899342689736,1.),(1.,0.663229258567818,1.),(1.,0.662912812691936,
1.),(1.,0.661423454802151,1.),(1.,0.660523869740149,1.),(1.,0.659755087773086,
1.),(1.,0.659619291059147,1.),(1.,0.659442901571928,1.),(1.,0.659388657238171,
1.),(1.,0.659289365428024,1.),(1.,0.659244263596543,1.),(1.,0.659042755870835,
1.),(1.,0.658958196453633,1.),(1.,0.658926561787994,1.),(1.,0.65919923542524,
1.),(1.,0.659916945733705,1.),(1.,0.660080071316468,1.),(1.,0.66044206006233,
1.),(1.,0.660640827665059,1.),(1.,0.66128959367181,1.),(1.,0.661791926833545,
1.),(1.,0.662935104672839,1.),(1.,0.663575947273059,1.),(1.,0.664643501128785,
1.),(1.,0.665017098787334,1.),(1.,0.665800623734546,1.),(1.,0.666211239135607,
1.),(1.,0.668333553785471,1.),(1.,0.670266144225975,1.),(1.,0.673518819932723,
1.),(1.,0.674662432543349,1.),(1.,0.676169720992961,1.),(1.,0.676475354929264,
1.),(1.,0.677091212222312,1.),(1.,0.677401785378898,1.),(1.,0.67834139879166,
1.),(1.,0.678978329515477,1.),(1.,0.68221536599383,1.),(1.,0.684971199140434,
1.),(1.,0.68863449272668,1.),(1.,0.689378165047444,1.),(1.,0.690888190776147,
1.),(1.,0.691650293315998,1.),(1.,0.693949128739525,1.),(1.,0.695502049311963,
1.),(1.,0.698649001495033,1.),(1.,0.700243032118734,1.),(1.,0.703473401016461,
1.),(1.,0.705110202255672,1.),(1.,0.706768250621048,1.)))
REPRESENTATION_ITEM('')
SURFACE()
);
#152=(
BOUNDED_SURFACE()
B_SPLINE_SURFACE(3,2,((#39384,#39385,#39386),(#39387,#39388,#39389),(#39390,
#39391,#39392),(#39393,#39394,#39395),(#39396,#39397,#39398),(#39399,#39400,
#39401),(#39402,#39403,#39404),(#39405,#39406,#39407),(#39408,#39409,#39410),
(#39411,#39412,#39413),(#39414,#39415,#39416),(#39417,#39418,#39419),(#39420,
#39421,#39422),(#39423,#39424,#39425),(#39426,#39427,#39428),(#39429,#39430,
#39431),(#39432,#39433,#39434),(#39435,#39436,#39437),(#39438,#39439,#39440),
(#39441,#39442,#39443),(#39444,#39445,#39446),(#39447,#39448,#39449),(#39450,
#39451,#39452),(#39453,#39454,#39455),(#39456,#39457,#39458),(#39459,#39460,
#39461),(#39462,#39463,#39464),(#39465,#39466,#39467),(#39468,#39469,#39470),
(#39471,#39472,#39473),(#39474,#39475,#39476),(#39477,#39478,#39479),(#39480,
#39481,#39482),(#39483,#39484,#39485),(#39486,#39487,#39488),(#39489,#39490,
#39491),(#39492,#39493,#39494),(#39495,#39496,#39497),(#39498,#39499,#39500),
(#39501,#39502,#39503),(#39504,#39505,#39506),(#39507,#39508,#39509),(#39510,
#39511,#39512),(#39513,#39514,#39515),(#39516,#39517,#39518),(#39519,#39520,
#39521),(#39522,#39523,#39524),(#39525,#39526,#39527),(#39528,#39529,#39530),
(#39531,#39532,#39533),(#39534,#39535,#39536),(#39537,#39538,#39539),(#39540,
#39541,#39542),(#39543,#39544,#39545),(#39546,#39547,#39548),(#39549,#39550,
#39551),(#39552,#39553,#39554),(#39555,#39556,#39557),(#39558,#39559,#39560),
(#39561,#39562,#39563),(#39564,#39565,#39566),(#39567,#39568,#39569),(#39570,
#39571,#39572),(#39573,#39574,#39575),(#39576,#39577,#39578),(#39579,#39580,
#39581),(#39582,#39583,#39584),(#39585,#39586,#39587),(#39588,#39589,#39590),
(#39591,#39592,#39593),(#39594,#39595,#39596),(#39597,#39598,#39599),(#39600,
#39601,#39602),(#39603,#39604,#39605),(#39606,#39607,#39608),(#39609,#39610,
#39611),(#39612,#39613,#39614),(#39615,#39616,#39617),(#39618,#39619,#39620),
(#39621,#39622,#39623),(#39624,#39625,#39626),(#39627,#39628,#39629),(#39630,
#39631,#39632),(#39633,#39634,#39635),(#39636,#39637,#39638),(#39639,#39640,
#39641),(#39642,#39643,#39644),(#39645,#39646,#39647),(#39648,#39649,#39650),
(#39651,#39652,#39653),(#39654,#39655,#39656),(#39657,#39658,#39659),(#39660,
#39661,#39662),(#39663,#39664,#39665),(#39666,#39667,#39668),(#39669,#39670,
#39671),(#39672,#39673,#39674),(#39675,#39676,#39677),(#39678,#39679,#39680),
(#39681,#39682,#39683),(#39684,#39685,#39686),(#39687,#39688,#39689),(#39690,
#39691,#39692),(#39693,#39694,#39695),(#39696,#39697,#39698),(#39699,#39700,
#39701),(#39702,#39703,#39704),(#39705,#39706,#39707),(#39708,#39709,#39710),
(#39711,#39712,#39713),(#39714,#39715,#39716),(#39717,#39718,#39719),(#39720,
#39721,#39722),(#39723,#39724,#39725),(#39726,#39727,#39728),(#39729,#39730,
#39731),(#39732,#39733,#39734),(#39735,#39736,#39737),(#39738,#39739,#39740),
(#39741,#39742,#39743),(#39744,#39745,#39746),(#39747,#39748,#39749),(#39750,
#39751,#39752),(#39753,#39754,#39755),(#39756,#39757,#39758),(#39759,#39760,
#39761),(#39762,#39763,#39764),(#39765,#39766,#39767),(#39768,#39769,#39770),
(#39771,#39772,#39773),(#39774,#39775,#39776),(#39777,#39778,#39779),(#39780,
#39781,#39782),(#39783,#39784,#39785),(#39786,#39787,#39788),(#39789,#39790,
#39791),(#39792,#39793,#39794),(#39795,#39796,#39797),(#39798,#39799,#39800),
(#39801,#39802,#39803),(#39804,#39805,#39806),(#39807,#39808,#39809),(#39810,
#39811,#39812),(#39813,#39814,#39815),(#39816,#39817,#39818),(#39819,#39820,
#39821),(#39822,#39823,#39824),(#39825,#39826,#39827)),.UNSPECIFIED.,.T.,
 .F.,.F.)
B_SPLINE_SURFACE_WITH_KNOTS((4,2,2,2,2,2,2,2,2,2,2,2,2,2,2,2,2,2,2,2,2,
2,2,2,2,2,2,2,2,2,2,2,2,2,2,2,2,2,2,2,2,2,2,2,2,2,2,2,2,2,2,2,2,2,2,2,2,
2,2,2,2,2,2,2,2,2,2,2,2,2,2,2,2,4),(3,3),(0.,2.94572120696205E-5,5.89144241392409E-5,
8.83716362088614E-5,0.000103100242243672,0.000117828848278482,0.000176743272417723,
0.000206200484487343,0.000235657696556964,0.000294572120696205,0.000309300726731015,
0.000324029332765825,0.000353486544835446,0.000382943756905066,0.000397672362939876,
0.000405036665957281,0.000412400968974686,0.000471315393113927,0.000500772605183548,
0.000515501211218358,0.000530229817253168,0.000589144241392409,0.00060387284742722,
0.00061860145346203,0.00064805866553165,0.000706973089670891,0.000721701695705701,
0.000736430301740512,0.000765887513810132,0.000795344725879752,0.000810073331914563,
0.000824801937949373,0.000883716362088614,0.000898444968123424,0.000913173574158234,
0.000942630786227855,0.000972087998297475,0.000986816604332285,0.0010015452103671,
0.00106045963450634,0.00107518824054115,0.00108255254355855,0.00108991684657596,
0.00111937405864558,0.00117828848278482,0.00119301708881963,0.00120774569485444,
0.00123720290692406,0.00126666011899368,0.00128138872502849,0.0012961173310633,
0.00135503175520254,0.00136976036123735,0.00137712466425476,0.00138448896727216,
0.00141394617934178,0.00147286060348102,0.00148758920951583,0.00150231781555064,
0.00153177502762026,0.00156123223968988,0.00157596084572469,0.00159068945175951,
0.00164960387589875,0.00167906108796837,0.00168642539098577,0.00169378969400318,
0.00170851830003799,0.00176743272417723,0.00178216133021204,0.00179688993624685,
0.00182634714831647,0.00185580436038609,0.00188526157245571),(0.,1.),
 .UNSPECIFIED.)
GEOMETRIC_REPRESENTATION_ITEM()
RATIONAL_B_SPLINE_SURFACE(((1.,0.706768250621048,1.),(1.,0.708426298986424,
1.),(1.,0.71008008713948,1.),(1.,0.713376962618569,1.),(1.,0.715020497077106,
1.),(1.,0.718297519423347,1.),(1.,0.719931010200883,1.),(1.,0.722372962983203,
1.),(1.,0.723186044045656,1.),(1.,0.724807250742798,1.),(1.,0.725609732738587,
1.),(1.,0.729581079301821,1.),(1.,0.732629067598119,1.),(1.,0.736998113914005,
1.),(1.,0.738421550016217,1.),(1.,0.741190319959484,1.),(1.,0.742514778054944,
1.),(1.,0.74631005642732,1.),(1.,0.748604628218609,1.),(1.,0.751158032017892,
1.),(1.,0.751653549012408,1.),(1.,0.752608572928937,1.),(1.,0.75306560396881,
1.),(1.,0.754375982622539,1.),(1.,0.755168745312861,1.),(1.,0.756593080986396,
1.),(1.,0.757224656832598,1.),(1.,0.758048217054286,1.),(1.,0.758302072136257,
1.),(1.,0.758651166057736,1.),(1.,0.758762248731274,1.),(1.,0.758973701473796,
1.),(1.,0.759074180129559,1.),(1.,0.75992529243238,1.),(1.,0.760313664756985,
1.),(1.,0.760358379138884,1.),(1.,0.760283061324181,1.),(1.,0.760031210406024,
1.),(1.,0.759923663695399,1.),(1.,0.759664049141739,1.),(1.,0.759511979981949,
1.),(1.,0.758642742016197,1.),(1.,0.757601675913755,1.),(1.,0.755877310483683,
1.),(1.,0.755511111609718,1.),(1.,0.754735567621713,1.),(1.,0.75432615177884,
1.),(1.,0.753047436476538,1.),(1.,0.752123540268788,1.),(1.,0.749147228369339,
1.),(1.,0.746892043597223,1.),(1.,0.743737116871849,1.),(1.,0.743092518946092,
1.),(1.,0.741782460083778,1.),(1.,0.74111613029348,1.),(1.,0.739084256899976,
1.),(1.,0.737685905862985,1.),(1.,0.734804890076589,1.),(1.,0.733322221436288,
1.),(1.,0.731035362741923,1.),(1.,0.730261837049612,1.),(1.,0.728696721731266,
1.),(1.,0.727910041758493,1.),(1.,0.723956994901979,1.),(1.,0.72073248846334,
1.),(1.,0.716630623834303,1.),(1.,0.715806638742097,1.),(1.,0.71415140110213,
1.),(1.,0.713318880580274,1.),(1.,0.710818889674067,1.),(1.,0.709159874596443,
1.),(1.,0.705856827432451,1.),(1.,0.704212795668421,1.),(1.,0.701757740368045,
1.),(1.,0.70094258809021,1.),(1.,0.699329967906212,1.),(1.,0.698530836824196,
1.),(1.,0.694570217898487,1.),(1.,0.691513076412309,1.),(1.,0.68782527710447,
1.),(1.,0.687094446903374,1.),(1.,0.686008340574591,1.),(1.,0.685647981698853,
1.),(1.,0.684934623703741,1.),(1.,0.684581117243663,1.),(1.,0.682829208835022,
1.),(1.,0.681477582738208,1.),(1.,0.677566315979365,1.),(1.,0.675148976138824,
1.),(1.,0.672364992202017,1.),(1.,0.671822976516116,1.),(1.,0.670773369616535,
1.),(1.,0.670264872579329,1.),(1.,0.668787238113039,1.),(1.,0.667865848198686,
1.),(1.,0.666147791049292,1.),(1.,0.665351122681227,1.),(1.,0.664250505737303,
1.),(1.,0.663899342689736,1.),(1.,0.663229258567818,1.),(1.,0.662912812691936,
1.),(1.,0.661423454802151,1.),(1.,0.660523869740149,1.),(1.,0.659755087773086,
1.),(1.,0.659619291059147,1.),(1.,0.659442901571928,1.),(1.,0.659388657238171,
1.),(1.,0.659289365428024,1.),(1.,0.659244263596543,1.),(1.,0.659042755870835,
1.),(1.,0.658958196453633,1.),(1.,0.658926561787994,1.),(1.,0.65919923542524,
1.),(1.,0.659916945733705,1.),(1.,0.660080071316468,1.),(1.,0.66044206006233,
1.),(1.,0.660640827665059,1.),(1.,0.66128959367181,1.),(1.,0.661791926833545,
1.),(1.,0.662935104672839,1.),(1.,0.663575947273059,1.),(1.,0.664643501128785,
1.),(1.,0.665017098787334,1.),(1.,0.665800623734546,1.),(1.,0.666211239135607,
1.),(1.,0.668333553785471,1.),(1.,0.670266144225975,1.),(1.,0.673518819932723,
1.),(1.,0.674662432543349,1.),(1.,0.676169720992961,1.),(1.,0.676475354929264,
1.),(1.,0.677091212222312,1.),(1.,0.677401785378898,1.),(1.,0.67834139879166,
1.),(1.,0.678978329515477,1.),(1.,0.68221536599383,1.),(1.,0.684971199140434,
1.),(1.,0.68863449272668,1.),(1.,0.689378165047444,1.),(1.,0.690888190776147,
1.),(1.,0.691650293315998,1.),(1.,0.693949128739525,1.),(1.,0.695502049311963,
1.),(1.,0.698649001495033,1.),(1.,0.700243032118734,1.),(1.,0.703473401016461,
1.),(1.,0.705110202255672,1.),(1.,0.706768250621048,1.)))
REPRESENTATION_ITEM('')
SURFACE()
);
#153=(
BOUNDED_SURFACE()
B_SPLINE_SURFACE(3,2,((#40039,#40040,#40041),(#40042,#40043,#40044),(#40045,
#40046,#40047),(#40048,#40049,#40050),(#40051,#40052,#40053),(#40054,#40055,
#40056),(#40057,#40058,#40059),(#40060,#40061,#40062),(#40063,#40064,#40065),
(#40066,#40067,#40068),(#40069,#40070,#40071),(#40072,#40073,#40074),(#40075,
#40076,#40077),(#40078,#40079,#40080),(#40081,#40082,#40083),(#40084,#40085,
#40086),(#40087,#40088,#40089),(#40090,#40091,#40092),(#40093,#40094,#40095),
(#40096,#40097,#40098),(#40099,#40100,#40101),(#40102,#40103,#40104),(#40105,
#40106,#40107),(#40108,#40109,#40110),(#40111,#40112,#40113),(#40114,#40115,
#40116),(#40117,#40118,#40119),(#40120,#40121,#40122),(#40123,#40124,#40125),
(#40126,#40127,#40128),(#40129,#40130,#40131),(#40132,#40133,#40134),(#40135,
#40136,#40137),(#40138,#40139,#40140),(#40141,#40142,#40143),(#40144,#40145,
#40146),(#40147,#40148,#40149),(#40150,#40151,#40152),(#40153,#40154,#40155),
(#40156,#40157,#40158),(#40159,#40160,#40161),(#40162,#40163,#40164),(#40165,
#40166,#40167),(#40168,#40169,#40170),(#40171,#40172,#40173),(#40174,#40175,
#40176),(#40177,#40178,#40179),(#40180,#40181,#40182),(#40183,#40184,#40185),
(#40186,#40187,#40188),(#40189,#40190,#40191),(#40192,#40193,#40194),(#40195,
#40196,#40197),(#40198,#40199,#40200),(#40201,#40202,#40203),(#40204,#40205,
#40206),(#40207,#40208,#40209),(#40210,#40211,#40212),(#40213,#40214,#40215),
(#40216,#40217,#40218),(#40219,#40220,#40221),(#40222,#40223,#40224),(#40225,
#40226,#40227),(#40228,#40229,#40230),(#40231,#40232,#40233),(#40234,#40235,
#40236),(#40237,#40238,#40239),(#40240,#40241,#40242),(#40243,#40244,#40245),
(#40246,#40247,#40248),(#40249,#40250,#40251),(#40252,#40253,#40254),(#40255,
#40256,#40257),(#40258,#40259,#40260),(#40261,#40262,#40263),(#40264,#40265,
#40266),(#40267,#40268,#40269),(#40270,#40271,#40272),(#40273,#40274,#40275),
(#40276,#40277,#40278),(#40279,#40280,#40281),(#40282,#40283,#40284),(#40285,
#40286,#40287),(#40288,#40289,#40290),(#40291,#40292,#40293),(#40294,#40295,
#40296),(#40297,#40298,#40299),(#40300,#40301,#40302),(#40303,#40304,#40305),
(#40306,#40307,#40308),(#40309,#40310,#40311),(#40312,#40313,#40314),(#40315,
#40316,#40317),(#40318,#40319,#40320),(#40321,#40322,#40323),(#40324,#40325,
#40326),(#40327,#40328,#40329),(#40330,#40331,#40332),(#40333,#40334,#40335),
(#40336,#40337,#40338),(#40339,#40340,#40341),(#40342,#40343,#40344),(#40345,
#40346,#40347),(#40348,#40349,#40350),(#40351,#40352,#40353),(#40354,#40355,
#40356),(#40357,#40358,#40359),(#40360,#40361,#40362),(#40363,#40364,#40365),
(#40366,#40367,#40368),(#40369,#40370,#40371),(#40372,#40373,#40374),(#40375,
#40376,#40377),(#40378,#40379,#40380),(#40381,#40382,#40383),(#40384,#40385,
#40386),(#40387,#40388,#40389),(#40390,#40391,#40392),(#40393,#40394,#40395),
(#40396,#40397,#40398),(#40399,#40400,#40401),(#40402,#40403,#40404),(#40405,
#40406,#40407),(#40408,#40409,#40410),(#40411,#40412,#40413),(#40414,#40415,
#40416),(#40417,#40418,#40419),(#40420,#40421,#40422),(#40423,#40424,#40425),
(#40426,#40427,#40428),(#40429,#40430,#40431),(#40432,#40433,#40434),(#40435,
#40436,#40437),(#40438,#40439,#40440),(#40441,#40442,#40443),(#40444,#40445,
#40446),(#40447,#40448,#40449),(#40450,#40451,#40452),(#40453,#40454,#40455),
(#40456,#40457,#40458),(#40459,#40460,#40461),(#40462,#40463,#40464),(#40465,
#40466,#40467),(#40468,#40469,#40470),(#40471,#40472,#40473),(#40474,#40475,
#40476),(#40477,#40478,#40479),(#40480,#40481,#40482)),.UNSPECIFIED.,.T.,
 .F.,.F.)
B_SPLINE_SURFACE_WITH_KNOTS((4,2,2,2,2,2,2,2,2,2,2,2,2,2,2,2,2,2,2,2,2,
2,2,2,2,2,2,2,2,2,2,2,2,2,2,2,2,2,2,2,2,2,2,2,2,2,2,2,2,2,2,2,2,2,2,2,2,
2,2,2,2,2,2,2,2,2,2,2,2,2,2,2,2,4),(3,3),(0.,5.88439546912971E-5,8.82659320369456E-5,
0.00010297692070977,0.000117687909382594,0.000176531864073891,0.000191242852746715,
0.00020595384141954,0.000235375818765188,0.000294219773456485,0.000301575267792897,
0.00030893076212931,0.000323641750802134,0.000353063728147782,0.000382485705493431,
0.000397196694166255,0.000404552188502667,0.000411907682839079,0.000470751637530376,
0.000500173614876025,0.000514884603548849,0.000529595592221674,0.00058843954691297,
0.000603150535585795,0.000617861524258619,0.000647283501604268,0.000706127456295565,
0.000713482950631977,0.000720838444968389,0.000735549433641213,0.000764971410986862,
0.00079439338833251,0.000809104377005334,0.000823815365678159,0.000882659320369456,
0.00089737030904228,0.000912081297715104,0.000941503275060753,0.000970925252406401,
0.000985636241079226,0.00100034722975205,0.00105919118444335,0.00107390217311617,
0.001088613161789,0.00111803513913464,0.00117687909382594,0.00120630107117159,
0.00123572304851724,0.00126514502586289,0.00127985601453571,0.00129456700320854,
0.00135341095789983,0.00136812194657266,0.00138283293524548,0.00141225491259113,
0.00147109886728243,0.00147845436161884,0.00148580985595525,0.00150052084462807,
0.00152994282197372,0.00155936479931937,0.0015740757879922,0.00158878677666502,
0.00164763073135632,0.00167705270870197,0.00168440820303838,0.00169176369737479,
0.00170647468604761,0.00176531864073891,0.00178002962941174,0.00179474061808456,
0.00182416259543021,0.00185358457277586,0.00188300655012151),(0.,1.),
 .UNSPECIFIED.)
GEOMETRIC_REPRESENTATION_ITEM()
RATIONAL_B_SPLINE_SURFACE(((1.,0.715726527571974,1.),(1.,0.712824837312312,
1.),(1.,0.709939183288703,1.),(1.,0.70563780485041,1.),(1.,0.704208324053071,
1.),(1.,0.702070408823295,1.),(1.,0.701358182508267,1.),(1.,0.699938470033913,
1.),(1.,0.699235558344621,1.),(1.,0.695754807328025,1.),(1.,0.693077556893273,
1.),(1.,0.689858407232006,1.),(1.,0.689220997236269,1.),(1.,0.687959045727463,
1.),(1.,0.687333603220981,1.),(1.,0.685482641655898,1.),(1.,0.684295233247551,
1.),(1.,0.680865948622576,1.),(1.,0.678755828779441,1.),(1.,0.676577048170574,
1.),(1.,0.676337696500587,1.),(1.,0.675864499150325,1.),(1.,0.675630328898002,
1.),(1.,0.674939074618547,1.),(1.,0.674493188941281,1.),(1.,0.673199210425328,
1.),(1.,0.672394697221168,1.),(1.,0.670898516819421,1.),(1.,0.67020685543305,
1.),(1.,0.669254011840167,1.),(1.,0.668950530912342,1.),(1.,0.668516758864078,
1.),(1.,0.668375744076451,1.),(1.,0.668100931680429,1.),(1.,0.66796703830326,
1.),(1.,0.666801110120948,1.),(1.,0.666028636022973,1.),(1.,0.665248431462833,
1.),(1.,0.665051947055941,1.),(1.,0.664854970332435,1.),(1.,0.664805603591522,
1.),(1.,0.664740760515236,1.),(1.,0.664725098690157,1.),(1.,0.664729031892036,
1.),(1.,0.664992831063146,1.),(1.,0.665649916349412,1.),(1.,0.665797857858843,
1.),(1.,0.666127492088933,1.),(1.,0.666309421952839,1.),(1.,0.666899952411735,
1.),(1.,0.667354870043226,1.),(1.,0.668899800350139,1.),(1.,0.670168108270442,
1.),(1.,0.671877972859038,1.),(1.,0.672071972172369,1.),(1.,0.672465766634245,
1.),(1.,0.672665825106501,1.),(1.,0.673275414881356,1.),(1.,0.673694356676243,
1.),(1.,0.674988511758639,1.),(1.,0.675900966431535,1.),(1.,0.677825804601594,
1.),(1.,0.678838181026788,1.),(1.,0.680434320387322,1.),(1.,0.680979480786494,
1.),(1.,0.682095794766937,1.),(1.,0.682662909252039,1.),(1.,0.68554058312361,
1.),(1.,0.687978699058213,1.),(1.,0.69120098153353,1.),(1.,0.691854240148126,
1.),(1.,0.693178775224038,1.),(1.,0.693851046877455,1.),(1.,0.695888940711959,
1.),(1.,0.697266250733029,1.),(1.,0.700058726696578,1.),(1.,0.701473890706926,
1.),(1.,0.703625959383263,1.),(1.,0.704345718616287,1.),(1.,0.705783355102051,
1.),(1.,0.706502269097388,1.),(1.,0.71009740810345,1.),(1.,0.712975541569779,
1.),(1.,0.716575141001572,1.),(1.,0.717295144791949,1.),(1.,0.718735249984781,
1.),(1.,0.719451276741359,1.),(1.,0.721578968626909,1.),(1.,0.722973916817993,
1.),(1.,0.727088200171688,1.),(1.,0.729737986565996,1.),(1.,0.733557197223877,
1.),(1.,0.734784504108155,1.),(1.,0.737143649706032,1.),(1.,0.738276364056428,
1.),(1.,0.740446615586834,1.),(1.,0.741484163457107,1.),(1.,0.742965865508942,
1.),(1.,0.743447540320556,1.),(1.,0.744384190268116,1.),(1.,0.744835768417984,
1.),(1.,0.747010115951137,1.),(1.,0.748485471872314,1.),(1.,0.749993321046985,
1.),(1.,0.750277933331016,1.),(1.,0.750812495848506,1.),(1.,0.751062871482513,
1.),(1.,0.751757652067472,1.),(1.,0.752142025968554,1.),(1.,0.753064753379183,
1.),(1.,0.753374703098945,1.),(1.,0.753370274811438,1.),(1.,0.753364836618584,
1.),(1.,0.753343954153974,1.),(1.,0.753328486568168,1.),(1.,0.753267330936153,
1.),(1.,0.753206862795746,1.),(1.,0.752967583346212,1.),(1.,0.752731013298035,
1.),(1.,0.752107006678872,1.),(1.,0.751719566002465,1.),(1.,0.751024658994972,
1.),(1.,0.75077403600156,1.),(1.,0.750234324747068,1.),(1.,0.749944553237197,
1.),(1.,0.748414981448763,1.),(1.,0.746926622748835,1.),(1.,0.744319366838701,
1.),(1.,0.743387383255421,1.),(1.,0.742142765249864,1.),(1.,0.741889533171004,
1.),(1.,0.74137762258562,1.),(1.,0.74111874517533,1.),(1.,0.740333498527515,
1.),(1.,0.739798515633772,1.),(1.,0.737067782822572,1.),(1.,0.73470619863159,
1.),(1.,0.731541347327889,1.),(1.,0.73089763158831,1.),(1.,0.729588498808487,
1.),(1.,0.728926359265131,1.),(1.,0.726927210402846,1.),(1.,0.725573615722195,
1.),(1.,0.722827030199711,1.),(1.,0.721434033464342,1.),(1.,0.718609414473237,
1.),(1.,0.717177372701805,1.),(1.,0.715726527571974,1.)))
REPRESENTATION_ITEM('')
SURFACE()
);
#154=(
BOUNDED_SURFACE()
B_SPLINE_SURFACE(3,2,((#40484,#40485,#40486,#40487,#40488,#40489,#40490,
#40491,#40492,#40493,#40494,#40495,#40496,#40497,#40498,#40499,#40500,#40501,
#40502,#40503,#40504,#40505,#40506,#40507,#40508,#40509,#40510,#40511,#40512,
#40513,#40514,#40515,#40516,#40517,#40518,#40519,#40520,#40521,#40522,#40523,
#40524,#40525,#40526,#40527,#40528,#40529,#40530,#40531,#40532,#40533,#40534,
#40535,#40536,#40537,#40538,#40539,#40540,#40541,#40542,#40543,#40544,#40545,
#40546,#40547,#40548,#40549,#40550,#40551,#40552,#40553,#40554,#40555,#40556,
#40557,#40558,#40559,#40560,#40561,#40562,#40563,#40564,#40565,#40566,#40567,
#40568,#40569,#40570,#40571,#40572,#40573,#40574,#40575,#40576,#40577,#40578,
#40579,#40580,#40581,#40582,#40583,#40584,#40585,#40586,#40587,#40588,#40589,
#40590,#40591,#40592,#40593,#40594,#40595,#40596,#40597,#40598,#40599,#40600,
#40601,#40602,#40603,#40604),(#40605,#40606,#40607,#40608,#40609,#40610,
#40611,#40612,#40613,#40614,#40615,#40616,#40617,#40618,#40619,#40620,#40621,
#40622,#40623,#40624,#40625,#40626,#40627,#40628,#40629,#40630,#40631,#40632,
#40633,#40634,#40635,#40636,#40637,#40638,#40639,#40640,#40641,#40642,#40643,
#40644,#40645,#40646,#40647,#40648,#40649,#40650,#40651,#40652,#40653,#40654,
#40655,#40656,#40657,#40658,#40659,#40660,#40661,#40662,#40663,#40664,#40665,
#40666,#40667,#40668,#40669,#40670,#40671,#40672,#40673,#40674,#40675,#40676,
#40677,#40678,#40679,#40680,#40681,#40682,#40683,#40684,#40685,#40686,#40687,
#40688,#40689,#40690,#40691,#40692,#40693,#40694,#40695,#40696,#40697,#40698,
#40699,#40700,#40701,#40702,#40703,#40704,#40705,#40706,#40707,#40708,#40709,
#40710,#40711,#40712,#40713,#40714,#40715,#40716,#40717,#40718,#40719,#40720,
#40721,#40722,#40723,#40724,#40725),(#40726,#40727,#40728,#40729,#40730,
#40731,#40732,#40733,#40734,#40735,#40736,#40737,#40738,#40739,#40740,#40741,
#40742,#40743,#40744,#40745,#40746,#40747,#40748,#40749,#40750,#40751,#40752,
#40753,#40754,#40755,#40756,#40757,#40758,#40759,#40760,#40761,#40762,#40763,
#40764,#40765,#40766,#40767,#40768,#40769,#40770,#40771,#40772,#40773,#40774,
#40775,#40776,#40777,#40778,#40779,#40780,#40781,#40782,#40783,#40784,#40785,
#40786,#40787,#40788,#40789,#40790,#40791,#40792,#40793,#40794,#40795,#40796,
#40797,#40798,#40799,#40800,#40801,#40802,#40803,#40804,#40805,#40806,#40807,
#40808,#40809,#40810,#40811,#40812,#40813,#40814,#40815,#40816,#40817,#40818,
#40819,#40820,#40821,#40822,#40823,#40824,#40825,#40826,#40827,#40828,#40829,
#40830,#40831,#40832,#40833,#40834,#40835,#40836,#40837,#40838,#40839,#40840,
#40841,#40842,#40843,#40844,#40845,#40846),(#40847,#40848,#40849,#40850,
#40851,#40852,#40853,#40854,#40855,#40856,#40857,#40858,#40859,#40860,#40861,
#40862,#40863,#40864,#40865,#40866,#40867,#40868,#40869,#40870,#40871,#40872,
#40873,#40874,#40875,#40876,#40877,#40878,#40879,#40880,#40881,#40882,#40883,
#40884,#40885,#40886,#40887,#40888,#40889,#40890,#40891,#40892,#40893,#40894,
#40895,#40896,#40897,#40898,#40899,#40900,#40901,#40902,#40903,#40904,#40905,
#40906,#40907,#40908,#40909,#40910,#40911,#40912,#40913,#40914,#40915,#40916,
#40917,#40918,#40919,#40920,#40921,#40922,#40923,#40924,#40925,#40926,#40927,
#40928,#40929,#40930,#40931,#40932,#40933,#40934,#40935,#40936,#40937,#40938,
#40939,#40940,#40941,#40942,#40943,#40944,#40945,#40946,#40947,#40948,#40949,
#40950,#40951,#40952,#40953,#40954,#40955,#40956,#40957,#40958,#40959,#40960,
#40961,#40962,#40963,#40964,#40965,#40966,#40967),(#40968,#40969,#40970,
#40971,#40972,#40973,#40974,#40975,#40976,#40977,#40978,#40979,#40980,#40981,
#40982,#40983,#40984,#40985,#40986,#40987,#40988,#40989,#40990,#40991,#40992,
#40993,#40994,#40995,#40996,#40997,#40998,#40999,#41000,#41001,#41002,#41003,
#41004,#41005,#41006,#41007,#41008,#41009,#41010,#41011,#41012,#41013,#41014,
#41015,#41016,#41017,#41018,#41019,#41020,#41021,#41022,#41023,#41024,#41025,
#41026,#41027,#41028,#41029,#41030,#41031,#41032,#41033,#41034,#41035,#41036,
#41037,#41038,#41039,#41040,#41041,#41042,#41043,#41044,#41045,#41046,#41047,
#41048,#41049,#41050,#41051,#41052,#41053,#41054,#41055,#41056,#41057,#41058,
#41059,#41060,#41061,#41062,#41063,#41064,#41065,#41066,#41067,#41068,#41069,
#41070,#41071,#41072,#41073,#41074,#41075,#41076,#41077,#41078,#41079,#41080,
#41081,#41082,#41083,#41084,#41085,#41086,#41087,#41088),(#41089,#41090,
#41091,#41092,#41093,#41094,#41095,#41096,#41097,#41098,#41099,#41100,#41101,
#41102,#41103,#41104,#41105,#41106,#41107,#41108,#41109,#41110,#41111,#41112,
#41113,#41114,#41115,#41116,#41117,#41118,#41119,#41120,#41121,#41122,#41123,
#41124,#41125,#41126,#41127,#41128,#41129,#41130,#41131,#41132,#41133,#41134,
#41135,#41136,#41137,#41138,#41139,#41140,#41141,#41142,#41143,#41144,#41145,
#41146,#41147,#41148,#41149,#41150,#41151,#41152,#41153,#41154,#41155,#41156,
#41157,#41158,#41159,#41160,#41161,#41162,#41163,#41164,#41165,#41166,#41167,
#41168,#41169,#41170,#41171,#41172,#41173,#41174,#41175,#41176,#41177,#41178,
#41179,#41180,#41181,#41182,#41183,#41184,#41185,#41186,#41187,#41188,#41189,
#41190,#41191,#41192,#41193,#41194,#41195,#41196,#41197,#41198,#41199,#41200,
#41201,#41202,#41203,#41204,#41205,#41206,#41207,#41208,#41209),(#41210,
#41211,#41212,#41213,#41214,#41215,#41216,#41217,#41218,#41219,#41220,#41221,
#41222,#41223,#41224,#41225,#41226,#41227,#41228,#41229,#41230,#41231,#41232,
#41233,#41234,#41235,#41236,#41237,#41238,#41239,#41240,#41241,#41242,#41243,
#41244,#41245,#41246,#41247,#41248,#41249,#41250,#41251,#41252,#41253,#41254,
#41255,#41256,#41257,#41258,#41259,#41260,#41261,#41262,#41263,#41264,#41265,
#41266,#41267,#41268,#41269,#41270,#41271,#41272,#41273,#41274,#41275,#41276,
#41277,#41278,#41279,#41280,#41281,#41282,#41283,#41284,#41285,#41286,#41287,
#41288,#41289,#41290,#41291,#41292,#41293,#41294,#41295,#41296,#41297,#41298,
#41299,#41300,#41301,#41302,#41303,#41304,#41305,#41306,#41307,#41308,#41309,
#41310,#41311,#41312,#41313,#41314,#41315,#41316,#41317,#41318,#41319,#41320,
#41321,#41322,#41323,#41324,#41325,#41326,#41327,#41328,#41329,#41330)),
 .UNSPECIFIED.,.T.,.F.,.F.)
B_SPLINE_SURFACE_WITH_KNOTS((4,3,4),(3,2,2,2,2,2,2,2,2,2,2,2,2,2,2,2,2,
2,2,2,2,2,2,2,2,2,2,2,2,2,2,2,2,2,2,2,2,2,2,2,2,2,2,2,2,2,2,2,2,2,2,2,2,
2,2,2,2,2,2,2,3),(0.,0.5,1.),(0.,0.0166666666666666,0.0333333333333333,
0.05,0.0666666666666667,0.0833333333333333,0.1,0.116666666666667,0.133333333333333,
0.15,0.166666666666667,0.183333333333334,0.2,0.216666666666667,0.233333333333334,
0.25,0.266666666666667,0.283333333333334,0.3,0.316666666666666,0.333333333333334,
0.35,0.366666666666666,0.383333333333334,0.4,0.416666666666667,0.433333333333334,
0.45,0.466666666666667,0.483333333333333,0.5,0.516666666666667,0.533333333333333,
0.55,0.566666666666667,0.583333333333333,0.6,0.616666666666667,0.633333333333333,
0.65,0.666666666666667,0.683333333333333,0.7,0.716666666666667,0.733333333333333,
0.75,0.766666666666667,0.783333333333333,0.8,0.816666666666667,0.833333333333333,
0.85,0.866666666666667,0.883333333333333,0.9,0.916666666666667,0.933333333333333,
0.95,0.966666666666667,0.983333333333333,1.),.UNSPECIFIED.)
GEOMETRIC_REPRESENTATION_ITEM()
RATIONAL_B_SPLINE_SURFACE(((1.,0.866025403784439,1.,0.866025403784439,1.,
0.866025403784439,1.,0.866025403784439,1.,0.866025403784439,1.,0.866025403784439,
1.,0.866025403784439,1.,0.866025403784439,1.,0.866025403784439,1.,0.866025403784439,
1.,0.866025403784439,1.,0.866025403784439,1.,0.866025403784439,1.,0.866025403784439,
1.,0.866025403784439,1.,0.866025403784439,1.,0.866025403784439,1.,0.866025403784439,
1.,0.866025403784439,1.,0.866025403784439,1.,0.866025403784439,1.,0.866025403784439,
1.,0.866025403784439,1.,0.866025403784439,1.,0.866025403784439,1.,0.866025403784439,
1.,0.866025403784439,1.,0.866025403784439,1.,0.866025403784439,1.,0.866025403784439,
1.,0.866025403784439,1.,0.866025403784439,1.,0.866025403784439,1.,0.866025403784439,
1.,0.866025403784439,1.,0.866025403784439,1.,0.866025403784439,1.,0.866025403784439,
1.,0.866025403784439,1.,0.866025403784439,1.,0.866025403784439,1.,0.866025403784439,
1.,0.866025403784439,1.,0.866025403784439,1.,0.866025403784439,1.,0.866025403784439,
1.,0.866025403784439,1.,0.866025403784439,1.,0.866025403784439,1.,0.866025403784439,
1.,0.866025403784439,1.,0.866025403784439,1.,0.866025403784439,1.,0.866025403784439,
1.,0.866025403784439,1.,0.866025403784439,1.,0.866025403784439,1.,0.866025403784439,
1.,0.866025403784439,1.,0.866025403784439,1.),(0.333333333333334,0.288675134594813,
0.333333333333334,0.288675134594813,0.333333333333334,0.288675134594813,
0.333333333333334,0.288675134594813,0.333333333333334,0.288675134594813,
0.333333333333334,0.288675134594813,0.333333333333334,0.288675134594813,
0.333333333333334,0.288675134594813,0.333333333333334,0.288675134594813,
0.333333333333334,0.288675134594813,0.333333333333334,0.288675134594813,
0.333333333333334,0.288675134594813,0.333333333333334,0.288675134594813,
0.333333333333334,0.288675134594813,0.333333333333334,0.288675134594813,
0.333333333333334,0.288675134594813,0.333333333333334,0.288675134594813,
0.333333333333334,0.288675134594813,0.333333333333334,0.288675134594813,
0.333333333333334,0.288675134594813,0.333333333333334,0.288675134594813,
0.333333333333334,0.288675134594813,0.333333333333334,0.288675134594813,
0.333333333333334,0.288675134594813,0.333333333333334,0.288675134594813,
0.333333333333334,0.288675134594813,0.333333333333334,0.288675134594813,
0.333333333333334,0.288675134594813,0.333333333333334,0.288675134594813,
0.333333333333334,0.288675134594813,0.333333333333334,0.288675134594813,
0.333333333333334,0.288675134594813,0.333333333333334,0.288675134594813,
0.333333333333334,0.288675134594813,0.333333333333334,0.288675134594813,
0.333333333333334,0.288675134594813,0.333333333333334,0.288675134594813,
0.333333333333334,0.288675134594813,0.333333333333334,0.288675134594813,
0.333333333333334,0.288675134594813,0.333333333333334,0.288675134594813,
0.333333333333334,0.288675134594813,0.333333333333334,0.288675134594813,
0.333333333333334,0.288675134594813,0.333333333333334,0.288675134594813,
0.333333333333334,0.288675134594813,0.333333333333334,0.288675134594813,
0.333333333333334,0.288675134594813,0.333333333333334,0.288675134594813,
0.333333333333334,0.288675134594813,0.333333333333334,0.288675134594813,
0.333333333333334,0.288675134594813,0.333333333333334,0.288675134594813,
0.333333333333334,0.288675134594813,0.333333333333334,0.288675134594813,
0.333333333333334,0.288675134594813,0.333333333333334,0.288675134594813,
0.333333333333334,0.288675134594813,0.333333333333334,0.288675134594813,
0.333333333333334,0.288675134594813,0.333333333333334),(0.333333333333334,
0.288675134594813,0.333333333333334,0.288675134594813,0.333333333333334,
0.288675134594813,0.333333333333334,0.288675134594813,0.333333333333334,
0.288675134594813,0.333333333333334,0.288675134594813,0.333333333333334,
0.288675134594813,0.333333333333334,0.288675134594813,0.333333333333334,
0.288675134594813,0.333333333333334,0.288675134594813,0.333333333333334,
0.288675134594813,0.333333333333334,0.288675134594813,0.333333333333334,
0.288675134594813,0.333333333333334,0.288675134594813,0.333333333333334,
0.288675134594813,0.333333333333334,0.288675134594813,0.333333333333334,
0.288675134594813,0.333333333333334,0.288675134594813,0.333333333333334,
0.288675134594813,0.333333333333334,0.288675134594813,0.333333333333334,
0.288675134594813,0.333333333333334,0.288675134594813,0.333333333333334,
0.288675134594813,0.333333333333334,0.288675134594813,0.333333333333334,
0.288675134594813,0.333333333333334,0.288675134594813,0.333333333333334,
0.288675134594813,0.333333333333334,0.288675134594813,0.333333333333334,
0.288675134594813,0.333333333333334,0.288675134594813,0.333333333333334,
0.288675134594813,0.333333333333334,0.288675134594813,0.333333333333334,
0.288675134594813,0.333333333333334,0.288675134594813,0.333333333333334,
0.288675134594813,0.333333333333334,0.288675134594813,0.333333333333334,
0.288675134594813,0.333333333333334,0.288675134594813,0.333333333333334,
0.288675134594813,0.333333333333334,0.288675134594813,0.333333333333334,
0.288675134594813,0.333333333333334,0.288675134594813,0.333333333333334,
0.288675134594813,0.333333333333334,0.288675134594813,0.333333333333334,
0.288675134594813,0.333333333333334,0.288675134594813,0.333333333333334,
0.288675134594813,0.333333333333334,0.288675134594813,0.333333333333334,
0.288675134594813,0.333333333333334,0.288675134594813,0.333333333333334,
0.288675134594813,0.333333333333334,0.288675134594813,0.333333333333334,
0.288675134594813,0.333333333333334,0.288675134594813,0.333333333333334,
0.288675134594813,0.333333333333334,0.288675134594813,0.333333333333334,
0.288675134594813,0.333333333333334,0.288675134594813,0.333333333333334,
0.288675134594813,0.333333333333334,0.288675134594813,0.333333333333334),
(1.,0.866025403784439,1.,0.866025403784439,1.,0.866025403784439,1.,0.866025403784439,
1.,0.866025403784439,1.,0.866025403784439,1.,0.866025403784439,1.,0.866025403784439,
1.,0.866025403784439,1.,0.866025403784439,1.,0.866025403784439,1.,0.866025403784439,
1.,0.866025403784439,1.,0.866025403784439,1.,0.866025403784439,1.,0.866025403784439,
1.,0.866025403784439,1.,0.866025403784439,1.,0.866025403784439,1.,0.866025403784439,
1.,0.866025403784439,1.,0.866025403784439,1.,0.866025403784439,1.,0.866025403784439,
1.,0.866025403784439,1.,0.866025403784439,1.,0.866025403784439,1.,0.866025403784439,
1.,0.866025403784439,1.,0.866025403784439,1.,0.866025403784439,1.,0.866025403784439,
1.,0.866025403784439,1.,0.866025403784439,1.,0.866025403784439,1.,0.866025403784439,
1.,0.866025403784439,1.,0.866025403784439,1.,0.866025403784439,1.,0.866025403784439,
1.,0.866025403784439,1.,0.866025403784439,1.,0.866025403784439,1.,0.866025403784439,
1.,0.866025403784439,1.,0.866025403784439,1.,0.866025403784439,1.,0.866025403784439,
1.,0.866025403784439,1.,0.866025403784439,1.,0.866025403784439,1.,0.866025403784439,
1.,0.866025403784439,1.,0.866025403784439,1.,0.866025403784439,1.,0.866025403784439,
1.,0.866025403784439,1.,0.866025403784439,1.,0.866025403784439,1.,0.866025403784439,
1.),(0.333333333333334,0.288675134594813,0.333333333333334,0.288675134594813,
0.333333333333334,0.288675134594813,0.333333333333334,0.288675134594813,
0.333333333333334,0.288675134594813,0.333333333333334,0.288675134594813,
0.333333333333334,0.288675134594813,0.333333333333334,0.288675134594813,
0.333333333333334,0.288675134594813,0.333333333333334,0.288675134594813,
0.333333333333334,0.288675134594813,0.333333333333334,0.288675134594813,
0.333333333333334,0.288675134594813,0.333333333333334,0.288675134594813,
0.333333333333334,0.288675134594813,0.333333333333334,0.288675134594813,
0.333333333333334,0.288675134594813,0.333333333333334,0.288675134594813,
0.333333333333334,0.288675134594813,0.333333333333334,0.288675134594813,
0.333333333333334,0.288675134594813,0.333333333333334,0.288675134594813,
0.333333333333334,0.288675134594813,0.333333333333334,0.288675134594813,
0.333333333333334,0.288675134594813,0.333333333333334,0.288675134594813,
0.333333333333334,0.288675134594813,0.333333333333334,0.288675134594813,
0.333333333333334,0.288675134594813,0.333333333333334,0.288675134594813,
0.333333333333334,0.288675134594813,0.333333333333334,0.288675134594813,
0.333333333333334,0.288675134594813,0.333333333333334,0.288675134594813,
0.333333333333334,0.288675134594813,0.333333333333334,0.288675134594813,
0.333333333333334,0.288675134594813,0.333333333333334,0.288675134594813,
0.333333333333334,0.288675134594813,0.333333333333334,0.288675134594813,
0.333333333333334,0.288675134594813,0.333333333333334,0.288675134594813,
0.333333333333334,0.288675134594813,0.333333333333334,0.288675134594813,
0.333333333333334,0.288675134594813,0.333333333333334,0.288675134594813,
0.333333333333334,0.288675134594813,0.333333333333334,0.288675134594813,
0.333333333333334,0.288675134594813,0.333333333333334,0.288675134594813,
0.333333333333334,0.288675134594813,0.333333333333334,0.288675134594813,
0.333333333333334,0.288675134594813,0.333333333333334,0.288675134594813,
0.333333333333334,0.288675134594813,0.333333333333334,0.288675134594813,
0.333333333333334,0.288675134594813,0.333333333333334,0.288675134594813,
0.333333333333334,0.288675134594813,0.333333333333334,0.288675134594813,
0.333333333333334),(0.333333333333334,0.288675134594813,0.333333333333334,
0.288675134594813,0.333333333333334,0.288675134594813,0.333333333333334,
0.288675134594813,0.333333333333334,0.288675134594813,0.333333333333334,
0.288675134594813,0.333333333333334,0.288675134594813,0.333333333333334,
0.288675134594813,0.333333333333334,0.288675134594813,0.333333333333334,
0.288675134594813,0.333333333333334,0.288675134594813,0.333333333333334,
0.288675134594813,0.333333333333334,0.288675134594813,0.333333333333334,
0.288675134594813,0.333333333333334,0.288675134594813,0.333333333333334,
0.288675134594813,0.333333333333334,0.288675134594813,0.333333333333334,
0.288675134594813,0.333333333333334,0.288675134594813,0.333333333333334,
0.288675134594813,0.333333333333334,0.288675134594813,0.333333333333334,
0.288675134594813,0.333333333333334,0.288675134594813,0.333333333333334,
0.288675134594813,0.333333333333334,0.288675134594813,0.333333333333334,
0.288675134594813,0.333333333333334,0.288675134594813,0.333333333333334,
0.288675134594813,0.333333333333334,0.288675134594813,0.333333333333334,
0.288675134594813,0.333333333333334,0.288675134594813,0.333333333333334,
0.288675134594813,0.333333333333334,0.288675134594813,0.333333333333334,
0.288675134594813,0.333333333333334,0.288675134594813,0.333333333333334,
0.288675134594813,0.333333333333334,0.288675134594813,0.333333333333334,
0.288675134594813,0.333333333333334,0.288675134594813,0.333333333333334,
0.288675134594813,0.333333333333334,0.288675134594813,0.333333333333334,
0.288675134594813,0.333333333333334,0.288675134594813,0.333333333333334,
0.288675134594813,0.333333333333334,0.288675134594813,0.333333333333334,
0.288675134594813,0.333333333333334,0.288675134594813,0.333333333333334,
0.288675134594813,0.333333333333334,0.288675134594813,0.333333333333334,
0.288675134594813,0.333333333333334,0.288675134594813,0.333333333333334,
0.288675134594813,0.333333333333334,0.288675134594813,0.333333333333334,
0.288675134594813,0.333333333333334,0.288675134594813,0.333333333333334,
0.288675134594813,0.333333333333334,0.288675134594813,0.333333333333334,
0.288675134594813,0.333333333333334,0.288675134594813,0.333333333333334,
0.288675134594813,0.333333333333334),(1.,0.866025403784439,1.,0.866025403784439,
1.,0.866025403784439,1.,0.866025403784439,1.,0.866025403784439,1.,0.866025403784439,
1.,0.866025403784439,1.,0.866025403784439,1.,0.866025403784439,1.,0.866025403784439,
1.,0.866025403784439,1.,0.866025403784439,1.,0.866025403784439,1.,0.866025403784439,
1.,0.866025403784439,1.,0.866025403784439,1.,0.866025403784439,1.,0.866025403784439,
1.,0.866025403784439,1.,0.866025403784439,1.,0.866025403784439,1.,0.866025403784439,
1.,0.866025403784439,1.,0.866025403784439,1.,0.866025403784439,1.,0.866025403784439,
1.,0.866025403784439,1.,0.866025403784439,1.,0.866025403784439,1.,0.866025403784439,
1.,0.866025403784439,1.,0.866025403784439,1.,0.866025403784439,1.,0.866025403784439,
1.,0.866025403784439,1.,0.866025403784439,1.,0.866025403784439,1.,0.866025403784439,
1.,0.866025403784439,1.,0.866025403784439,1.,0.866025403784439,1.,0.866025403784439,
1.,0.866025403784439,1.,0.866025403784439,1.,0.866025403784439,1.,0.866025403784439,
1.,0.866025403784439,1.,0.866025403784439,1.,0.866025403784439,1.,0.866025403784439,
1.,0.866025403784439,1.,0.866025403784439,1.,0.866025403784439,1.,0.866025403784439,
1.,0.866025403784439,1.,0.866025403784439,1.,0.866025403784439,1.,0.866025403784439,
1.,0.866025403784439,1.,0.866025403784439,1.)))
REPRESENTATION_ITEM('')
SURFACE()
);
#155=(
BOUNDED_SURFACE()
B_SPLINE_SURFACE(3,2,((#41507,#41508,#41509),(#41510,#41511,#41512),(#41513,
#41514,#41515),(#41516,#41517,#41518),(#41519,#41520,#41521),(#41522,#41523,
#41524),(#41525,#41526,#41527),(#41528,#41529,#41530),(#41531,#41532,#41533),
(#41534,#41535,#41536),(#41537,#41538,#41539),(#41540,#41541,#41542),(#41543,
#41544,#41545),(#41546,#41547,#41548),(#41549,#41550,#41551),(#41552,#41553,
#41554),(#41555,#41556,#41557),(#41558,#41559,#41560),(#41561,#41562,#41563),
(#41564,#41565,#41566),(#41567,#41568,#41569),(#41570,#41571,#41572),(#41573,
#41574,#41575),(#41576,#41577,#41578),(#41579,#41580,#41581),(#41582,#41583,
#41584),(#41585,#41586,#41587),(#41588,#41589,#41590),(#41591,#41592,#41593),
(#41594,#41595,#41596),(#41597,#41598,#41599),(#41600,#41601,#41602),(#41603,
#41604,#41605),(#41606,#41607,#41608),(#41609,#41610,#41611),(#41612,#41613,
#41614),(#41615,#41616,#41617),(#41618,#41619,#41620),(#41621,#41622,#41623),
(#41624,#41625,#41626),(#41627,#41628,#41629),(#41630,#41631,#41632)),
 .UNSPECIFIED.,.F.,.F.,.F.)
B_SPLINE_SURFACE_WITH_KNOTS((4,2,2,2,2,2,2,2,2,2,2,2,2,2,2,2,2,2,2,2,4),
(3,3),(-0.000180428912156006,0.164606365078715,0.329212730157431,0.493819095236146,
0.658425460314861,0.823031825393576,0.987638190472292,1.15224455555101,
1.31685092062972,1.48145728570844,1.64606365078715,1.81067001586587,1.97527638094458,
2.05757956348394,2.1398827460233,2.22218592856266,2.30448911110201,2.38679229364137,
2.46909547618073,2.55139865872009,2.63370184125944),(-0.000180428912158174,
1.),.UNSPECIFIED.)
GEOMETRIC_REPRESENTATION_ITEM()
RATIONAL_B_SPLINE_SURFACE(((1.00002747362388,0.923865794144028,1.),(1.00002747283797,
0.923867972041735,1.),(1.00002778507159,0.923002718203409,1.),(1.00002903107801,
0.919549816980654,1.),(1.00002996427325,0.916963770134614,1.),(1.00003244208062,
0.910097333539332,1.),(1.00003398669916,0.905816926024921,1.),(1.00003767113923,
0.895606699673117,1.),(1.00003981097144,0.889676851216917,1.),(1.00004466281745,
0.876231539283259,1.),(1.00004737484772,0.868716030175813,1.),(1.0000533408798,
0.852183114223139,1.),(1.00005659490622,0.843165639185358,1.),(1.00006360694908,
0.823734044835397,1.),(1.00006736500184,0.813319824861043,1.),(1.00007533847186,
0.791223948081428,1.),(1.00007955394243,0.779542143552474,1.),(1.00008838568606,
0.755067840834176,1.),(1.00009300203695,0.742275126983019,1.),(1.00010256714128,
0.715768553807505,1.),(1.00010751600729,0.702054382506394,1.),(1.00011766312963,
0.673934935852508,1.),(1.00012286154571,0.659529217785071,1.),(1.00013340615476,
0.630308266094241,1.),(1.00013875256542,0.615492429246126,1.),(1.0001467886769,
0.593222962028068,1.),(1.00014946992156,0.585792765217129,1.),(1.00015481886695,
0.570969904149657,1.),(1.0001574865782,0.563577210768261,1.),(1.00016278762071,
0.548887096965589,1.),(1.00016542096244,0.541589647514159,1.),(1.00017062993481,
0.527154676129277,1.),(1.00017320557466,0.520017128655486,1.),(1.00017827307841,
0.505974191505765,1.),(1.00018076494827,0.499068785290728,1.),(1.00018563594977,
0.485570390172216,1.),(1.00018801508117,0.4789774019006,1.),(1.00019262873255,
0.466192168865366,1.),(1.00019486324215,0.459999952835799,1.),(1.00019915310735,
0.448111987809573,1.),(1.00020120841379,0.442416375004484,1.),(1.00020315589889,
0.437019553957336,1.)))
REPRESENTATION_ITEM('')
SURFACE()
);
#156=(
BOUNDED_SURFACE()
B_SPLINE_SURFACE(3,2,((#41656,#41657,#41658),(#41659,#41660,#41661),(#41662,
#41663,#41664),(#41665,#41666,#41667),(#41668,#41669,#41670),(#41671,#41672,
#41673),(#41674,#41675,#41676),(#41677,#41678,#41679),(#41680,#41681,#41682),
(#41683,#41684,#41685),(#41686,#41687,#41688),(#41689,#41690,#41691),(#41692,
#41693,#41694),(#41695,#41696,#41697),(#41698,#41699,#41700),(#41701,#41702,
#41703),(#41704,#41705,#41706),(#41707,#41708,#41709),(#41710,#41711,#41712),
(#41713,#41714,#41715),(#41716,#41717,#41718),(#41719,#41720,#41721),(#41722,
#41723,#41724),(#41725,#41726,#41727),(#41728,#41729,#41730),(#41731,#41732,
#41733),(#41734,#41735,#41736),(#41737,#41738,#41739),(#41740,#41741,#41742),
(#41743,#41744,#41745),(#41746,#41747,#41748),(#41749,#41750,#41751),(#41752,
#41753,#41754),(#41755,#41756,#41757),(#41758,#41759,#41760),(#41761,#41762,
#41763),(#41764,#41765,#41766),(#41767,#41768,#41769),(#41770,#41771,#41772),
(#41773,#41774,#41775),(#41776,#41777,#41778),(#41779,#41780,#41781),(#41782,
#41783,#41784),(#41785,#41786,#41787),(#41788,#41789,#41790),(#41791,#41792,
#41793),(#41794,#41795,#41796),(#41797,#41798,#41799)),.UNSPECIFIED.,.F.,
 .F.,.F.)
B_SPLINE_SURFACE_WITH_KNOTS((4,2,2,2,2,2,2,2,2,2,2,2,2,2,2,2,2,2,2,2,2,
2,2,4),(3,3),(0.00405715139965717,0.0042139480393906,0.00432957425184741,
0.00435848080496162,0.00438738735807582,0.00444520046430423,0.00456082667676104,
0.00458973322987524,0.00461863978298944,0.00467645288921785,0.00479207910167466,
0.00484989220790306,0.00490770531413147,0.00502333152658828,0.00513895773904509,
0.00516786429215929,0.0051967708452735,0.0052545839515019,0.00537021016395871,
0.00548583637641552,0.00560146258887234,0.00565927569510074,0.00571708880132915,
0.00594834122624277),(0.,1.00004117042728),.UNSPECIFIED.)
GEOMETRIC_REPRESENTATION_ITEM()
RATIONAL_B_SPLINE_SURFACE(((1.,0.921979058456473,1.000006424311),(1.,0.924596675875849,
1.00000620877414),(1.,0.926417326016543,1.00000605886026),(1.,0.92821880541024,
1.0000059105249),(1.,0.928558002582939,1.00000588259512),(1.,0.928433280614718,
1.00000589286483),(1.,0.928380610460445,1.00000589720174),(1.,0.928221595227939,
1.00000591029519),(1.,0.92811523092253,1.00000591905332),(1.,0.927717554191574,
1.00000595179836),(1.,0.927347749203701,1.00000598224842),(1.,0.925936429317906,
1.0000060984577),(1.,0.924594290701714,1.00000620897054),(1.,0.922434222240346,
1.00000638683242),(1.,0.921976988327732,1.00000642448146),(1.,0.921020155283146,
1.00000650326791),(1.,0.920520634377084,1.00000654439888),(1.,0.918960875377281,
1.00000667283077),(1.,0.917839524509904,1.00000676516376),(1.,0.914244283327225,
1.00000706119899),(1.,0.911540219248417,1.00000728385394),(1.,0.90705432648433,
1.00000765322618),(1.,0.905483610646325,1.00000778256027),(1.,0.902242131132709,
1.00000804946646),(1.,0.900567342069336,1.00000818737002),(1.,0.895389495139947,
1.00000861371837),(1.,0.891733580942485,1.00000891474946),(1.,0.884041048555298,
1.00000954815915),(1.,0.880004227665733,1.00000988055444),(1.,0.874725766434696,
1.00001031518745),(1.,0.87365841541306,1.00001040307404),(1.,0.871500398344183,
1.00001058076701),(1.,0.870409954167221,1.00001067055512),(1.,0.867119949574412,
1.0000109414569),(1.,0.864896413773187,1.00001112454474),(1.,0.858136741898467,
1.0000116811419),(1.,0.853511773742965,1.00001206196573),(1.,0.844026400946148,
1.00001284299943),(1.,0.839165945656301,1.00001324321348),(1.,0.829204144361192,
1.00001406347671),(1.,0.824102781547739,1.00001448352728),(1.,0.816261555954164,
1.0000151291805),(1.,0.813616239468941,1.00001534699812),(1.,0.80826050162453,
1.00001578799415),(1.,0.805555387411647,1.00001601073556),(1.,0.791956355880912,
1.00001713049144),(1.,0.780780298581849,1.00001805073755),(1.,0.769254523194895,
1.00001899977974)))
REPRESENTATION_ITEM('')
SURFACE()
);
#157=(
BOUNDED_SURFACE()
B_SPLINE_SURFACE(3,2,((#42035,#42036,#42037),(#42038,#42039,#42040),(#42041,
#42042,#42043),(#42044,#42045,#42046),(#42047,#42048,#42049),(#42050,#42051,
#42052),(#42053,#42054,#42055),(#42056,#42057,#42058),(#42059,#42060,#42061),
(#42062,#42063,#42064),(#42065,#42066,#42067),(#42068,#42069,#42070),(#42071,
#42072,#42073),(#42074,#42075,#42076),(#42077,#42078,#42079),(#42080,#42081,
#42082),(#42083,#42084,#42085),(#42086,#42087,#42088),(#42089,#42090,#42091),
(#42092,#42093,#42094),(#42095,#42096,#42097),(#42098,#42099,#42100),(#42101,
#42102,#42103),(#42104,#42105,#42106),(#42107,#42108,#42109),(#42110,#42111,
#42112),(#42113,#42114,#42115),(#42116,#42117,#42118),(#42119,#42120,#42121),
(#42122,#42123,#42124),(#42125,#42126,#42127),(#42128,#42129,#42130),(#42131,
#42132,#42133),(#42134,#42135,#42136),(#42137,#42138,#42139),(#42140,#42141,
#42142),(#42143,#42144,#42145),(#42146,#42147,#42148),(#42149,#42150,#42151),
(#42152,#42153,#42154),(#42155,#42156,#42157),(#42158,#42159,#42160),(#42161,
#42162,#42163),(#42164,#42165,#42166),(#42167,#42168,#42169),(#42170,#42171,
#42172),(#42173,#42174,#42175),(#42176,#42177,#42178),(#42179,#42180,#42181),
(#42182,#42183,#42184),(#42185,#42186,#42187),(#42188,#42189,#42190),(#42191,
#42192,#42193),(#42194,#42195,#42196),(#42197,#42198,#42199),(#42200,#42201,
#42202),(#42203,#42204,#42205),(#42206,#42207,#42208),(#42209,#42210,#42211),
(#42212,#42213,#42214),(#42215,#42216,#42217),(#42218,#42219,#42220),(#42221,
#42222,#42223),(#42224,#42225,#42226),(#42227,#42228,#42229),(#42230,#42231,
#42232)),.UNSPECIFIED.,.F.,.F.,.F.)
B_SPLINE_SURFACE_WITH_KNOTS((4,2,2,2,2,2,2,2,2,2,2,2,2,2,2,2,2,2,2,2,2,
2,2,2,2,2,2,2,2,2,2,2,4),(3,3),(4.7123634827097,4.84407407244766,4.97575916451063,
5.10744425657361,5.23912934863658,5.37081444069955,5.50249953276252,5.63418462482549,
5.76586971688847,5.89755480895144,6.02923990101441,6.16092499307738,6.29261008514036,
6.42429517720333,6.5559802692663,6.68766536132927,6.81935045339224,6.95103554545522,
7.08272063751819,7.21440572958116,7.34609082164413,7.4777759137071,7.60946100577008,
7.74114609783305,7.87283118989602,8.00451628195899,8.13620137402197,8.26788646608494,
8.39957155814791,8.53125665021088,8.66294174227385,8.79462683433682,8.9263119263998),
(-2.54976749745779E-5,1.0000200211984),.UNSPECIFIED.)
GEOMETRIC_REPRESENTATION_ITEM()
RATIONAL_B_SPLINE_SURFACE(((1.00001493677863,0.707089416884705,1.00001172854274),
(1.00001458276126,0.714031705927214,1.00001145056393),(1.0000142339983,
0.72087095578393,1.00001117671096),(1.00001355192398,0.734246449476047,
1.00001064113779),(1.00001321861735,0.740782600388391,1.00001037942132),
(1.00001257176904,0.753467310976227,1.00000987150805),(1.00001225822607,
0.759615896089341,1.00000962531024),(1.00001165474721,0.771450130927326,
1.0000091514512),(1.0000113648101,0.777135804508549,1.00000892378901),(1.00001081189245,
0.787978532648321,1.00000848963125),(1.00001054891083,0.793135608462434,
1.00000828313484),(1.00001005279086,0.802864532786016,1.00000789357533),
(1.00000981965159,0.80743639954397,1.00000771051149),(1.00000938566623,
0.815946862742293,1.00000736974084),(1.00000918481937,0.819885474363816,
1.00000721203341),(1.00000881745384,0.827089521022162,1.00000692357347),
(1.00000865093455,0.8303549682861,1.00000679282047),(1.00000835386198,0.836180568468688,
1.00000655955542),(1.00000822330822,0.838740730840915,1.000006457043),(1.00000799942127,
0.843131159125162,1.00000628124421),(1.00000790608774,0.844961431902458,
1.00000620795757),(1.00000775752295,0.847874791033107,1.00000609130266),
(1.00000770229146,0.848957881819088,1.00000604793422),(1.00000763044669,
0.850366759396511,1.00000599152082),(1.00000761383331,0.850692548296484,
1.00000597847579),(1.00000761937903,0.850583796497954,1.00000598283036),
(1.00000764153815,0.850149255637501,1.00000600022997),(1.00000772442274,
0.848523886858095,1.00000606531197),(1.00000778514834,0.847333056502543,
1.00000611299446),(1.00000794459767,0.844206251360263,1.00000623819604),
(1.00000804332165,0.842270271800573,1.00000631571532),(1.00000827783294,
0.837671499782725,1.00000649985648),(1.00000841362062,0.8350087000993,1.00000660647865),
(1.00000872095034,0.828981956938996,1.00000684779773),(1.00000889249289,
0.825618003623282,1.00000698249505),(1.00000926963831,0.818222172985636,
1.00000727863429),(1.00000947524183,0.814190283024086,1.00000744007671),
(1.00000991841571,0.805499632828679,1.0000077880623),(1.00001015598685,
0.800840856978932,1.00000797460609),(1.00001066058466,0.79094568201105,
1.00000837082251),(1.00001092761227,0.785709264204444,1.00000858049589),
(1.00001148817145,0.774716685456562,1.00000902065386),(1.00001178170412,
0.768960502851546,1.00000925113933),(1.00001239185506,0.756995428492058,
1.00000973023737),(1.00001270847456,0.750786512573754,1.00000997885091),
(1.00001336088375,0.737992752755806,1.00001049113065),(1.00001369667475,
0.73140788332834,1.00001075479788),(1.00001438298174,0.717949387037515,
1.00001129369459),(1.00001473349899,0.711075735492579,1.00001156892506),
(1.00001544425076,0.697137876382458,1.00001212701611),(1.0000158044863,
0.690073648827045,1.0000124098775),(1.00001652907635,0.675864420871923,
1.00001297883454),(1.00001689343131,0.668719411333768,1.00001326493055),
(1.0000176200554,0.654470295700902,1.00001383548474),(1.00001798232397,
0.647366200462238,1.00001411994249),(1.00001869797199,0.633332325987409,
1.00001468187813),(1.00001905134922,0.626402590046828,1.0000149593543),
(1.00001974186121,0.612861633591743,1.00001550155282),(1.00002007899133,
0.606250503907858,1.00001576627155),(1.00002072921578,0.593499586974255,
1.00001627683581),(1.00002104230228,0.587359953302464,1.00001652267519),
(1.00002163640176,0.57570964848589,1.00001698916942),(1.00002191740319,
0.570199203714092,1.00001720981521),(1.00002243935165,0.55996378210997,
1.00001761965557),(1.00002268029487,0.555238879860998,1.00001780884716),
(1.00002289743305,0.550980794913776,1.00001797934674)))
REPRESENTATION_ITEM('')
SURFACE()
);
#158=(
BOUNDED_SURFACE()
B_SPLINE_SURFACE(3,2,((#42415,#42416,#42417),(#42418,#42419,#42420),(#42421,
#42422,#42423),(#42424,#42425,#42426),(#42427,#42428,#42429),(#42430,#42431,
#42432),(#42433,#42434,#42435),(#42436,#42437,#42438),(#42439,#42440,#42441),
(#42442,#42443,#42444),(#42445,#42446,#42447),(#42448,#42449,#42450),(#42451,
#42452,#42453),(#42454,#42455,#42456),(#42457,#42458,#42459),(#42460,#42461,
#42462),(#42463,#42464,#42465),(#42466,#42467,#42468),(#42469,#42470,#42471),
(#42472,#42473,#42474),(#42475,#42476,#42477),(#42478,#42479,#42480),(#42481,
#42482,#42483),(#42484,#42485,#42486),(#42487,#42488,#42489),(#42490,#42491,
#42492),(#42493,#42494,#42495),(#42496,#42497,#42498),(#42499,#42500,#42501),
(#42502,#42503,#42504),(#42505,#42506,#42507),(#42508,#42509,#42510),(#42511,
#42512,#42513),(#42514,#42515,#42516)),.UNSPECIFIED.,.F.,.F.,.F.)
B_SPLINE_SURFACE_WITH_KNOTS((4,2,2,2,2,2,2,2,2,2,2,2,2,2,2,2,4),(3,3),(1.55194677087336,
1.74947440896781,1.94700204706227,2.14452968515673,2.34205732325119,2.53958496134565,
2.73711259944011,2.93464023753456,3.13216787562902,3.32969551372348,3.52722315181794,
3.7247507899124,3.92227842800686,4.11980606610132,4.31733370419577,4.51486134229023,
4.71238898038469),(-2.42766963556483E-5,1.),.UNSPECIFIED.)
GEOMETRIC_REPRESENTATION_ITEM()
RATIONAL_B_SPLINE_SURFACE(((1.00001436631327,0.704113091369118,1.),(1.00001385873323,
0.714567150498244,1.),(1.00001336171142,0.724803753602056,1.),(1.0000124041668,
0.744525230800647,1.),(1.00001194367891,0.754009385402698,1.),(1.00001107227999,
0.771956615694544,1.),(1.00001066136108,0.780419853575295,1.),(1.00000989969439,
0.796107051746786,1.),(1.00000954894,0.803331148053762,1.),(1.00000891601262,
0.816366846433687,1.),(1.00000863383454,0.822178553085928,1.),(1.0000081444562,
0.832257732352426,1.),(1.00000793725231,0.836525279419831,1.),(1.00000760233045,
0.843423290914308,1.),(1.00000747461017,0.846053802860064,1.),(1.00000730136028,
0.849622037199957,1.),(1.00000725582954,0.850559783059377,1.),(1.0000072479093,
0.850722907291969,1.),(1.00000728551976,0.849948286719655,1.),(1.00000744309521,
0.846702881275639,1.),(1.00000756306123,0.844232075124759,1.),(1.00000788280972,
0.837646572592139,1.),(1.00000808259438,0.833531831096325,1.),(1.0000085576446,
0.823747752192612,1.),(1.00000883291365,0.818078343045833,1.),(1.00000945271828,
0.805312919420194,1.),(1.00000979725879,0.798216803347918,1.),(1.00001054739183,
0.782767151031959,1.),(1.00001095299081,0.774413481699587,1.),(1.00001181486088,
0.756662506520888,1.),(1.00001227113974,0.747265040418406,1.),(1.00001322161599,
0.727689142842311,1.),(1.00001371577882,0.717511422999973,1.),(1.00001422130471,
0.707099670706811,1.)))
REPRESENTATION_ITEM('')
SURFACE()
);
#159=(
BOUNDED_SURFACE()
B_SPLINE_SURFACE(3,2,((#42564,#42565,#42566),(#42567,#42568,#42569),(#42570,
#42571,#42572),(#42573,#42574,#42575),(#42576,#42577,#42578),(#42579,#42580,
#42581),(#42582,#42583,#42584),(#42585,#42586,#42587),(#42588,#42589,#42590),
(#42591,#42592,#42593),(#42594,#42595,#42596),(#42597,#42598,#42599),(#42600,
#42601,#42602),(#42603,#42604,#42605),(#42606,#42607,#42608),(#42609,#42610,
#42611),(#42612,#42613,#42614),(#42615,#42616,#42617),(#42618,#42619,#42620),
(#42621,#42622,#42623),(#42624,#42625,#42626),(#42627,#42628,#42629),(#42630,
#42631,#42632),(#42633,#42634,#42635),(#42636,#42637,#42638),(#42639,#42640,
#42641)),.UNSPECIFIED.,.F.,.F.,.F.)
B_SPLINE_SURFACE_WITH_KNOTS((4,2,2,2,2,2,2,2,2,2,2,2,4),(3,3),(-8.02309607639273E-18,
0.000231201308553261,0.00046240261710653,0.000578003271383164,0.000635803598521482,
0.000693603925659799,0.000924805234213068,0.00115600654276634,0.00138720785131961,
0.00150280850559624,0.00156060883273456,0.00161840915987287,0.00184961046842614),
(0.,1.),.UNSPECIFIED.)
GEOMETRIC_REPRESENTATION_ITEM()
RATIONAL_B_SPLINE_SURFACE(((1.,0.707106781186546,1.),(1.,0.720929919393816,
1.),(1.,0.734604162805705,1.),(1.,0.761404742811728,1.),(1.,0.774530928339215,
1.),(1.,0.793676981797689,1.),(1.,0.799968971951391,1.),(1.,0.809258992556117,
1.),(1.,0.812331025452392,1.),(1.,0.818423859772064,1.),(1.,0.821445484452913,
1.),(1.,0.836344837847268,1.),(1.,0.847660204338874,1.),(1.,0.869100951414214,
1.),(1.,0.879226501171938,1.),(1.,0.898300415096302,1.),(1.,0.907248884122996,
1.),(1.,0.919790865749779,1.),(1.,0.923824653174569,1.),(1.,0.929654417556856,
1.),(1.,0.931560846523734,1.),(1.,0.935299871240406,1.),(1.,0.937133447719843,
1.),(1.,0.946081718428858,1.),(1.,0.952565822325163,1.),(1.,0.95841150296378,
1.)))
REPRESENTATION_ITEM('')
SURFACE()
);
#160=(
BOUNDED_SURFACE()
B_SPLINE_SURFACE(3,2,((#42685,#42686,#42687),(#42688,#42689,#42690),(#42691,
#42692,#42693),(#42694,#42695,#42696),(#42697,#42698,#42699),(#42700,#42701,
#42702),(#42703,#42704,#42705),(#42706,#42707,#42708),(#42709,#42710,#42711),
(#42712,#42713,#42714),(#42715,#42716,#42717),(#42718,#42719,#42720),(#42721,
#42722,#42723),(#42724,#42725,#42726),(#42727,#42728,#42729),(#42730,#42731,
#42732),(#42733,#42734,#42735),(#42736,#42737,#42738),(#42739,#42740,#42741),
(#42742,#42743,#42744),(#42745,#42746,#42747),(#42748,#42749,#42750),(#42751,
#42752,#42753),(#42754,#42755,#42756),(#42757,#42758,#42759),(#42760,#42761,
#42762)),.UNSPECIFIED.,.F.,.F.,.F.)
B_SPLINE_SURFACE_WITH_KNOTS((4,2,2,2,2,2,2,2,2,2,2,2,4),(3,3),(2.4611389315421E-17,
0.000231201308553273,0.000462402617106521,0.000578003271383145,0.000635803598521457,
0.000693603925659769,0.000924805234213017,0.00115600654276626,0.00138720785131951,
0.00150280850559614,0.00156060883273445,0.00161840915987276,0.00184961046842601),
(0.,1.),.UNSPECIFIED.)
GEOMETRIC_REPRESENTATION_ITEM()
RATIONAL_B_SPLINE_SURFACE(((1.,0.707106781186553,1.),(1.,0.720929919393856,
1.),(1.,0.734604162805657,1.),(1.,0.76140474281178,1.),(1.,0.774530928339167,
1.),(1.,0.79367698179771,1.),(1.,0.799968971951349,1.),(1.,0.809258992556132,
1.),(1.,0.812331025452404,1.),(1.,0.818423859772045,1.),(1.,0.821445484452912,
1.),(1.,0.836344837847255,1.),(1.,0.847660204338855,1.),(1.,0.869100951414219,
1.),(1.,0.879226501171922,1.),(1.,0.898300415096301,1.),(1.,0.907248884123008,
1.),(1.,0.919790865749757,1.),(1.,0.923824653174548,1.),(1.,0.929654417556854,
1.),(1.,0.931560846523727,1.),(1.,0.935299871240392,1.),(1.,0.937133447719837,
1.),(1.,0.946081718428836,1.),(1.,0.952565822325914,1.),(1.,0.958411502963771,
1.)))
REPRESENTATION_ITEM('')
SURFACE()
);
#161=(
BOUNDED_SURFACE()
B_SPLINE_SURFACE(3,2,((#42989,#42990,#42991),(#42992,#42993,#42994),(#42995,
#42996,#42997),(#42998,#42999,#43000),(#43001,#43002,#43003),(#43004,#43005,
#43006),(#43007,#43008,#43009),(#43010,#43011,#43012),(#43013,#43014,#43015),
(#43016,#43017,#43018),(#43019,#43020,#43021),(#43022,#43023,#43024),(#43025,
#43026,#43027),(#43028,#43029,#43030),(#43031,#43032,#43033),(#43034,#43035,
#43036),(#43037,#43038,#43039),(#43040,#43041,#43042),(#43043,#43044,#43045),
(#43046,#43047,#43048),(#43049,#43050,#43051),(#43052,#43053,#43054),(#43055,
#43056,#43057),(#43058,#43059,#43060),(#43061,#43062,#43063),(#43064,#43065,
#43066),(#43067,#43068,#43069),(#43070,#43071,#43072),(#43073,#43074,#43075),
(#43076,#43077,#43078),(#43079,#43080,#43081),(#43082,#43083,#43084),(#43085,
#43086,#43087),(#43088,#43089,#43090),(#43091,#43092,#43093),(#43094,#43095,
#43096),(#43097,#43098,#43099),(#43100,#43101,#43102),(#43103,#43104,#43105),
(#43106,#43107,#43108),(#43109,#43110,#43111),(#43112,#43113,#43114)),
 .UNSPECIFIED.,.F.,.F.,.F.)
B_SPLINE_SURFACE_WITH_KNOTS((4,2,2,2,2,2,2,2,2,2,2,2,2,2,2,2,2,2,2,2,4),
(3,3),(-1.14925430283463E-17,0.000184433511101772,0.000368867022203556,
0.000553300533305339,0.000645517288856231,0.000691625666631677,0.000737734044407122,
0.000922167555508906,0.00110660106661069,0.00147546808881426,0.00156768484436515,
0.00161379322214059,0.00165990159991604,0.00184433511101782,0.00221320213322139,
0.00258206915542496,0.00276650266652674,0.00285871942207763,0.00290482779985308,
0.0029278819887408,0.00295093617762852),(0.,1.),.UNSPECIFIED.)
GEOMETRIC_REPRESENTATION_ITEM()
RATIONAL_B_SPLINE_SURFACE(((1.,0.707106781186548,1.),(1.,0.718133109232454,
1.),(1.,0.729066449118189,1.),(1.,0.750613820444198,1.),(1.,0.761227677789341,
1.),(1.,0.782035992265971,1.),(1.,0.792230829853422,1.),(1.,0.807152370816259,
1.),(1.,0.812064584782534,1.),(1.,0.819334468682991,1.),(1.,0.821740098050387,
1.),(1.,0.826498417096085,1.),(1.,0.828853542546963,1.),(1.,0.840509377458955,
1.),(1.,0.849450761297905,1.),(1.,0.866576104208724,1.),(1.,0.874760117668752,
1.),(1.,0.898186376934544,1.),(1.,0.912305286226077,1.),(1.,0.928084784593313,
1.),(1.,0.931147041015764,1.),(1.,0.935599437228533,1.),(1.,0.937060508010849,
1.),(1.,0.939926548778915,1.),(1.,0.941332681223158,1.),(1.,0.948230522590508,
1.),(1.,0.953324197247602,1.),(1.,0.967382764235203,1.),(1.,0.975129434277988,
1.),(1.,0.987528841798518,1.),(1.,0.992181040796599,1.),(1.,0.996857896678297,
1.),(1.,0.998032308863382,1.),(1.,0.999210733877751,1.),(1.,0.999506280906549,
1.),(1.,0.999802327869022,1.),(1.,0.999876460522184,1.),(1.,0.99995062376894,
1.),(1.,0.999969172009759,1.),(1.,0.999993884192384,1.),(1.,1.00000001991537,
1.),(1.,1.,1.)))
REPRESENTATION_ITEM('')
SURFACE()
);
#162=(
BOUNDED_SURFACE()
B_SPLINE_SURFACE(3,2,((#43231,#43232,#43233),(#43234,#43235,#43236),(#43237,
#43238,#43239),(#43240,#43241,#43242),(#43243,#43244,#43245),(#43246,#43247,
#43248),(#43249,#43250,#43251),(#43252,#43253,#43254),(#43255,#43256,#43257),
(#43258,#43259,#43260),(#43261,#43262,#43263),(#43264,#43265,#43266),(#43267,
#43268,#43269),(#43270,#43271,#43272),(#43273,#43274,#43275),(#43276,#43277,
#43278),(#43279,#43280,#43281),(#43282,#43283,#43284)),.UNSPECIFIED.,.F.,
 .F.,.F.)
B_SPLINE_SURFACE_WITH_KNOTS((4,2,2,2,2,2,2,2,4),(3,3),(-0.000256146907527732,
0.196349540849362,0.392699081698724,0.589048622548086,0.785398163397448,
0.98174770424681,1.17809724509617,1.37444678594553,1.57105247370244),(0.,
1.00025614690754),.UNSPECIFIED.)
GEOMETRIC_REPRESENTATION_ITEM()
RATIONAL_B_SPLINE_SURFACE(((0.999999999999999,0.923860025992052,1.00003900603776),
(1.,0.92386380976833,1.00003900409936),(1.,0.922631950619233,1.00003963517318),
(1.,0.917721587618823,1.00004215072178),(1.,0.914045686726666,1.00004403386307),
(1.,0.904303507747054,1.00004902472111),(1.,0.898237178126564,1.00005213246425),
(1.,0.883805658263611,1.00005952564262),(1.,0.875440377644158,1.00006381112414),
(1.,0.856541795567702,1.00007349275085),(1.,0.846008345896188,1.00007888897197),
(1.,0.822947010606607,1.00009070315141),(1.,0.810418887616988,1.00009712123133),
(1.,0.783590096545192,1.00011086545506),(1.,0.769289052220745,1.00011819179162),
(1.,0.739173873609776,1.00013361961136),(1.,0.723358473879048,1.00014172174282),
(1.,0.706967696454818,1.00015011863672)))
REPRESENTATION_ITEM('')
SURFACE()
);
#163=(
BOUNDED_SURFACE()
B_SPLINE_SURFACE(3,2,((#43297,#43298,#43299),(#43300,#43301,#43302),(#43303,
#43304,#43305),(#43306,#43307,#43308),(#43309,#43310,#43311),(#43312,#43313,
#43314),(#43315,#43316,#43317),(#43318,#43319,#43320),(#43321,#43322,#43323),
(#43324,#43325,#43326),(#43327,#43328,#43329),(#43330,#43331,#43332),(#43333,
#43334,#43335),(#43336,#43337,#43338),(#43339,#43340,#43341),(#43342,#43343,
#43344),(#43345,#43346,#43347),(#43348,#43349,#43350)),.UNSPECIFIED.,.F.,
 .F.,.F.)
B_SPLINE_SURFACE_WITH_KNOTS((4,2,2,2,2,2,2,2,4),(3,3),(1.57060699273548,
1.76832396488935,1.96585160298381,2.16337924107827,2.36090687917273,2.55843451726719,
2.75596215536165,2.9534897934561,3.15101743155056),(0.,1.00018933405942),
 .UNSPECIFIED.)
GEOMETRIC_REPRESENTATION_ITEM()
RATIONAL_B_SPLINE_SURFACE(((1.,0.707003978702482,1.00011094825221),(1.,
0.72348593060803,1.00010470706249),(1.,0.739385892154352,1.00009868625396),
(1.,0.769656517851604,1.00008722373307),(1.,0.784027936045077,1.00008178173518),
(1.,0.8109731743871,1.00007157843247),(1.,0.823547380016532,1.00006681698167),
(1.,0.84667338193124,1.00005805990203),(1.,0.857225420695959,1.00005406418136),
(1.,0.876131519789516,1.00004690504439),(1.,0.884485731030333,1.00004374157093),
(1.,0.898864213201865,1.00003829689813),(1.,0.904888575770995,1.00003601566409),
(1.,0.914515552682844,1.00003237023486),(1.,0.91811821889335,1.00003100602002),
(1.,0.922848120955148,1.0000292149569),(1.,0.923975956543124,1.00002878788152),
(1.,0.923856620627319,1.00002883307023)))
REPRESENTATION_ITEM('')
SURFACE()
);
#164=(
BOUNDED_SURFACE()
B_SPLINE_SURFACE(3,2,((#43550,#43551,#43552),(#43553,#43554,#43555),(#43556,
#43557,#43558),(#43559,#43560,#43561),(#43562,#43563,#43564),(#43565,#43566,
#43567),(#43568,#43569,#43570),(#43571,#43572,#43573),(#43574,#43575,#43576),
(#43577,#43578,#43579),(#43580,#43581,#43582),(#43583,#43584,#43585),(#43586,
#43587,#43588),(#43589,#43590,#43591),(#43592,#43593,#43594),(#43595,#43596,
#43597),(#43598,#43599,#43600),(#43601,#43602,#43603),(#43604,#43605,#43606),
(#43607,#43608,#43609),(#43610,#43611,#43612),(#43613,#43614,#43615),(#43616,
#43617,#43618),(#43619,#43620,#43621),(#43622,#43623,#43624),(#43625,#43626,
#43627),(#43628,#43629,#43630),(#43631,#43632,#43633),(#43634,#43635,#43636),
(#43637,#43638,#43639),(#43640,#43641,#43642),(#43643,#43644,#43645),(#43646,
#43647,#43648),(#43649,#43650,#43651),(#43652,#43653,#43654),(#43655,#43656,
#43657),(#43658,#43659,#43660),(#43661,#43662,#43663),(#43664,#43665,#43666),
(#43667,#43668,#43669),(#43670,#43671,#43672),(#43673,#43674,#43675),(#43676,
#43677,#43678),(#43679,#43680,#43681),(#43682,#43683,#43684),(#43685,#43686,
#43687),(#43688,#43689,#43690),(#43691,#43692,#43693),(#43694,#43695,#43696),
(#43697,#43698,#43699),(#43700,#43701,#43702),(#43703,#43704,#43705),(#43706,
#43707,#43708),(#43709,#43710,#43711),(#43712,#43713,#43714),(#43715,#43716,
#43717),(#43718,#43719,#43720),(#43721,#43722,#43723),(#43724,#43725,#43726),
(#43727,#43728,#43729)),.UNSPECIFIED.,.F.,.F.,.F.)
B_SPLINE_SURFACE_WITH_KNOTS((4,2,2,2,2,2,2,2,2,2,2,2,2,2,2,2,2,2,2,2,2,
2,2,2,2,2,2,2,2,4),(3,3),(0.00356026658290825,0.00370761548845134,0.00385496439399443,
0.00400231329953753,0.0040391505259233,0.00407598775230907,0.00414966220508062,
0.00429701111062371,0.0044443600161668,0.00451803446893835,0.00455487169532412,
0.00459170892170989,0.00473905782725299,0.00488640673279608,0.00492324395918185,
0.00496008118556762,0.00503375563833917,0.00510743009111072,0.00514426731749649,
0.00516268593068938,0.00518110454388226,0.00532845344942535,0.0054021279021969,
0.00543896512858267,0.00547580235496845,0.00562315126051154,0.00565998848689731,
0.00569682571328309,0.00577050016605463,0.00591784907159772),(0.,1.),
 .UNSPECIFIED.)
GEOMETRIC_REPRESENTATION_ITEM()
RATIONAL_B_SPLINE_SURFACE(((1.,0.707106781186547,1.),(1.,0.714899530141188,
1.),(1.,0.722851116139554,1.),(1.,0.738965796907419,1.),(1.,0.747128767269762,
1.),(1.,0.763573562645999,1.),(1.,0.771855539406454,1.),(1.,0.782231613637912,
1.),(1.,0.784308029863662,1.),(1.,0.788462064530618,1.),(1.,0.790542242277229,
1.),(1.,0.796763962116366,1.),(1.,0.800876179008829,1.),(1.,0.813095262016546,
1.),(1.,0.821084755433325,1.),(1.,0.836691228945864,1.),(1.,0.844308581612572,
1.),(1.,0.855403320496569,1.),(1.,0.859046240981785,1.),(1.,0.864419493162934,
1.),(1.,0.86619721499557,1.),(1.,0.869701088492385,1.),(1.,0.871429334319563,
1.),(1.,0.879949489101844,1.),(1.,0.886380304852135,1.),(1.,0.898373764602034,
1.),(1.,0.903938066040975,1.),(1.,0.910243055457683,1.),(1.,0.911466373703979,
1.),(1.,0.913826788251488,1.),(1.,0.914965304917439,1.),(1.,0.918252475084136,
1.),(1.,0.920272999106784,1.),(1.,0.92394925395352,1.),(1.,0.925605070562256,
1.),(1.,0.927791488596373,1.),(1.,0.928470669980879,1.),(1.,0.929411224851904,
1.),(1.,0.929711916737623,1.),(1.,0.930283108179015,1.),(1.,0.930554076458367,
1.),(1.,0.932861253750851,1.),(1.,0.933980898903266,1.),(1.,0.934229809753535,
1.),(1.,0.934073575444518,1.),(1.,0.933468573302636,1.),(1.,0.933204148039385,
1.),(1.,0.932559198561778,1.),(1.,0.932178256466784,1.),(1.,0.929991263320291,
1.),(1.,0.927343365860572,1.),(1.,0.923016139346013,1.),(1.,0.922097237767011,
1.),(1.,0.920176288887714,1.),(1.,0.919173225434103,1.),(1.,0.91604297106036,
1.),(1.,0.913794973536961,1.),(1.,0.906609692179916,1.),(1.,0.901232273200219,
1.),(1.,0.895342042385736,1.)))
REPRESENTATION_ITEM('')
SURFACE()
);
#165=(
BOUNDED_SURFACE()
B_SPLINE_SURFACE(3,2,((#43985,#43986,#43987),(#43988,#43989,#43990),(#43991,
#43992,#43993),(#43994,#43995,#43996),(#43997,#43998,#43999),(#44000,#44001,
#44002),(#44003,#44004,#44005),(#44006,#44007,#44008),(#44009,#44010,#44011),
(#44012,#44013,#44014),(#44015,#44016,#44017),(#44018,#44019,#44020),(#44021,
#44022,#44023),(#44024,#44025,#44026),(#44027,#44028,#44029),(#44030,#44031,
#44032),(#44033,#44034,#44035),(#44036,#44037,#44038),(#44039,#44040,#44041),
(#44042,#44043,#44044),(#44045,#44046,#44047),(#44048,#44049,#44050),(#44051,
#44052,#44053),(#44054,#44055,#44056),(#44057,#44058,#44059),(#44060,#44061,
#44062),(#44063,#44064,#44065),(#44066,#44067,#44068),(#44069,#44070,#44071),
(#44072,#44073,#44074),(#44075,#44076,#44077),(#44078,#44079,#44080),(#44081,
#44082,#44083),(#44084,#44085,#44086),(#44087,#44088,#44089),(#44090,#44091,
#44092),(#44093,#44094,#44095),(#44096,#44097,#44098),(#44099,#44100,#44101),
(#44102,#44103,#44104),(#44105,#44106,#44107),(#44108,#44109,#44110),(#44111,
#44112,#44113),(#44114,#44115,#44116),(#44117,#44118,#44119),(#44120,#44121,
#44122),(#44123,#44124,#44125),(#44126,#44127,#44128)),.UNSPECIFIED.,.F.,
 .F.,.F.)
B_SPLINE_SURFACE_WITH_KNOTS((4,2,2,2,2,2,2,2,2,2,2,2,2,2,2,2,2,2,2,2,2,
2,2,4),(3,3),(-2.69186893279756E-5,0.000147491368261441,0.000294982736522876,
0.00044247410478431,0.000479346946849669,0.000516219788915028,0.000589965473045745,
0.00073745684130718,0.000884948209568615,0.000958693893699332,0.000995566735764691,
0.00103243957783005,0.00117993094609148,0.00132742231435292,0.00147491368261435,
0.00154865936674507,0.00162240505087579,0.00176989641913722,0.00191738778739866,
0.00199113347152937,0.00202800631359473,0.00206487915566009,0.00221237052392153,
0.00235986189218296),(0.,1.00002691868933),.UNSPECIFIED.)
GEOMETRIC_REPRESENTATION_ITEM()
RATIONAL_B_SPLINE_SURFACE(((1.,0.706934185382307,1.00001577789523),(1.,
0.707289966495766,1.00001575874091),(1.,0.707645413657456,1.00001573960457),
(1.,0.708300892599077,1.0000157043153),(1.,0.708601012305713,1.00001568815764),
(1.,0.709200732421921,1.00001565587028),(1.,0.709500333423245,1.00001563974055),
(1.,0.709874355785092,1.00001561960417),(1.,0.709949135907864,1.0000156155782),
(1.,0.710098641866628,1.00001560752919),(1.,0.710173473062381,1.00001560350048),
(1.,0.710396928789648,1.0000155914702),(1.,0.710544516885821,1.00001558352445),
(1.,0.710983142239652,1.00001555991001),(1.,0.711270053741346,1.00001554446345),
(1.,0.711832583115565,1.00001551417834),(1.,0.712108201699971,1.00001549933976),
(1.,0.712512623814919,1.00001547756673),(1.,0.712645926822463,1.00001547039005),
(1.,0.712843524542374,1.0000154597519),(1.,0.71290899741735,1.00001545622701),
(1.,0.713039137297051,1.00001544922063),(1.,0.713103803366072,1.00001544573917),
(1.,0.713423270431812,1.0000154285399),(1.,0.713667991894455,1.00001541536474),
(1.,0.714135658414077,1.0000153901868),(1.,0.714358602875164,1.00001537818406),
(1.,0.714781991002754,1.00001535538995),(1.,0.714982437280183,1.00001534459845),
(1.,0.715265182582933,1.00001532937618),(1.,0.715356610594333,1.00001532445394),
(1.,0.715531426705098,1.0000153150423),(1.,0.715615029916155,1.00001531054132),
(1.,0.715854496794294,1.00001529764905),(1.,0.715999041792887,1.00001528986713),
(1.,0.716257713229434,1.00001527594093),(1.,0.71637184060172,1.00001526979661),
(1.,0.716519464132329,1.00001526184895),(1.,0.716564737889815,1.00001525941153),
(1.,0.716626593197021,1.0000152560814),(1.,0.716646227239996,1.00001525502436),
(1.,0.716683289956507,1.000015253029),(1.,0.71670072325815,1.00001525209044),
(1.,0.716782447076519,1.00001524769064),(1.,0.716830443772986,1.00001524510662),
(1.,0.716892320380967,1.00001524177535),(1.,0.716906185847933,1.00001524102887),
(1.,0.71690292040473,1.00001524120467)))
REPRESENTATION_ITEM('')
SURFACE()
);
#166=(
BOUNDED_SURFACE()
B_SPLINE_SURFACE(3,2,((#44129,#44130,#44131),(#44132,#44133,#44134),(#44135,
#44136,#44137),(#44138,#44139,#44140),(#44141,#44142,#44143),(#44144,#44145,
#44146),(#44147,#44148,#44149),(#44150,#44151,#44152),(#44153,#44154,#44155),
(#44156,#44157,#44158),(#44159,#44160,#44161),(#44162,#44163,#44164),(#44165,
#44166,#44167),(#44168,#44169,#44170),(#44171,#44172,#44173),(#44174,#44175,
#44176),(#44177,#44178,#44179),(#44180,#44181,#44182),(#44183,#44184,#44185),
(#44186,#44187,#44188),(#44189,#44190,#44191),(#44192,#44193,#44194),(#44195,
#44196,#44197),(#44198,#44199,#44200),(#44201,#44202,#44203),(#44204,#44205,
#44206),(#44207,#44208,#44209),(#44210,#44211,#44212)),.UNSPECIFIED.,.F.,
 .F.,.F.)
B_SPLINE_SURFACE_WITH_KNOTS((4,2,2,2,2,2,2,2,2,2,2,2,2,4),(3,3),(0.00102826841024056,
0.00108136671720793,0.00113446502417531,0.00124066163811006,0.00134685825204482,
0.00145305486597957,0.00166544809384908,0.00187784132171859,0.00209023454958809,
0.0023026277774576,0.00251502100532711,0.00262121761926186,0.00267431592622924,
0.00272741423319662),(-0.00283459110010449,1.),.UNSPECIFIED.)
GEOMETRIC_REPRESENTATION_ITEM()
RATIONAL_B_SPLINE_SURFACE(((1.00166517176203,0.706276548675112,1.),(1.00163220101093,
0.712092334787547,1.),(1.00159961546054,0.717840174463587,1.),(1.00153520684576,
0.729201357172828,1.),(1.00150334087126,0.734822269214763,1.),(1.0014092038008,
0.751427322137522,1.),(1.00134853122035,0.762129497213199,1.),(1.00123109470163,
0.782844393043764,1.),(1.00117433210629,0.79285687691495,1.),(1.00106457774187,
0.812216699997259,1.),(1.00101158686358,0.821563882080632,1.),(1.00085819617163,
0.848620816667832,1.),(1.00076335541889,0.865349993715338,1.),(1.00058884175311,
0.896132857911678,1.),(1.00050918219483,0.910184189386343,1.),(1.00036597350955,
0.9354450965539,1.),(1.00030277669818,0.94659252649063,1.),(1.00019375601416,
0.96582293401015,1.),(1.00014793806965,0.97390486591732,1.),(1.00007430095644,
0.986893884547261,1.),(1.0000464877762,0.991799914951515,1.),(1.00001862499585,
0.996714694431725,1.),(1.00001164514357,0.997945886521746,1.),(1.00000466137374,
0.999177769636466,1.),(1.00000291429973,0.999485940011998,1.),(1.00000058402726,
0.999896982096644,1.),(1.00000000076916,0.999999864326373,1.),(1.,1.,1.)))
REPRESENTATION_ITEM('')
SURFACE()
);
#167=(
BOUNDED_SURFACE()
B_SPLINE_SURFACE(3,2,((#44276,#44277,#44278),(#44279,#44280,#44281),(#44282,
#44283,#44284),(#44285,#44286,#44287),(#44288,#44289,#44290),(#44291,#44292,
#44293),(#44294,#44295,#44296),(#44297,#44298,#44299),(#44300,#44301,#44302),
(#44303,#44304,#44305),(#44306,#44307,#44308),(#44309,#44310,#44311),(#44312,
#44313,#44314),(#44315,#44316,#44317),(#44318,#44319,#44320),(#44321,#44322,
#44323),(#44324,#44325,#44326),(#44327,#44328,#44329),(#44330,#44331,#44332),
(#44333,#44334,#44335),(#44336,#44337,#44338),(#44339,#44340,#44341),(#44342,
#44343,#44344),(#44345,#44346,#44347),(#44348,#44349,#44350),(#44351,#44352,
#44353),(#44354,#44355,#44356),(#44357,#44358,#44359)),.UNSPECIFIED.,.F.,
 .F.,.F.)
B_SPLINE_SURFACE_WITH_KNOTS((4,2,2,2,2,2,2,2,2,2,2,2,2,4),(3,3),(0.00102826841024098,
0.00108136671720835,0.00113446502417572,0.00124066163811045,0.00134685825204519,
0.00145305486597993,0.00166544809384941,0.00187784132171888,0.00209023454958836,
0.00230262777745784,0.00251502100532731,0.00262121761926205,0.00267431592622942,
0.00272741423319679),(0.,1.00283459127414),.UNSPECIFIED.)
GEOMETRIC_REPRESENTATION_ITEM()
RATIONAL_B_SPLINE_SURFACE(((1.,0.706276548624223,1.00166517186456),(1.,
0.712092334737677,1.00163220111142),(1.,0.717840174414683,1.00159961555903),
(1.,0.729201357125934,1.00153520694028),(1.,0.734822269168861,1.00150334096382),
(1.,0.75142732209438,1.00140920388756),(1.,0.762129497171982,1.00134853130338),
(1.,0.78284439300614,1.00123109477743),(1.,0.792856876879042,1.00117433217859),
(1.,0.812216699964743,1.00106457780742),(1.,0.821563882049743,1.00101158692587),
(1.,0.848620816641558,1.00085819622447),(1.,0.865349993692116,1.00076335546589),
(1.,0.89613285789359,1.00058884178937),(1.,0.9101841893708,1.00050918222618),
(1.,0.935445096542706,1.00036597353209),(1.,0.946592526481339,1.00030277671682),
(1.,0.965822934004271,1.00019375602609),(1.,0.973904865912868,1.00014793807876),
(1.,0.98689388454492,1.00007430096101),(1.,0.991799914950075,1.00004648777906),
(1.,0.996714694431167,1.000018624997),(1.,0.99794588652139,1.00001164514429),
(1.,0.999177769636325,1.00000466137403),(1.,0.999485940011916,1.00000291429991),
(1.,0.999896982096622,1.0000005840273),(1.,0.999999864326377,1.00000000076916),
(1.,1.,1.)))
REPRESENTATION_ITEM('')
SURFACE()
);
#224=FACE_BOUND('',#4912,.T.);
#225=FACE_BOUND('',#5012,.T.);
#226=FACE_BOUND('',#5013,.T.);
#227=FACE_BOUND('',#5014,.T.);
#228=FACE_BOUND('',#5015,.T.);
#229=FACE_BOUND('',#5017,.T.);
#230=FACE_BOUND('',#5043,.T.);
#231=FACE_BOUND('',#5050,.T.);
#530=PLANE('',#15986);
#531=PLANE('',#15987);
#532=PLANE('',#15989);
#533=PLANE('',#15990);
#534=PLANE('',#15991);
#535=PLANE('',#15992);
#536=PLANE('',#15993);
#537=PLANE('',#15994);
#538=PLANE('',#15995);
#539=PLANE('',#16014);
#540=PLANE('',#16022);
#541=PLANE('',#16023);
#542=PLANE('',#16024);
#543=PLANE('',#16027);
#544=PLANE('',#16030);
#545=PLANE('',#16031);
#546=PLANE('',#16032);
#547=PLANE('',#16045);
#548=PLANE('',#16046);
#549=PLANE('',#16065);
#550=PLANE('',#16077);
#551=PLANE('',#16078);
#552=PLANE('',#16079);
#553=PLANE('',#16080);
#554=PLANE('',#16099);
#555=PLANE('',#16101);
#556=PLANE('',#16102);
#557=PLANE('',#16107);
#558=PLANE('',#16110);
#559=PLANE('',#16116);
#560=PLANE('',#16119);
#561=PLANE('',#16122);
#562=PLANE('',#16124);
#563=PLANE('',#16140);
#564=PLANE('',#16147);
#565=PLANE('',#16154);
#566=PLANE('',#16155);
#567=PLANE('',#16168);
#568=PLANE('',#16169);
#569=PLANE('',#16170);
#570=PLANE('',#16171);
#571=PLANE('',#16173);
#572=PLANE('',#16174);
#573=PLANE('',#16175);
#755=ELLIPSE('',#15926,24.0416305514422,16.9999999877997);
#756=ELLIPSE('',#15969,0.7071067812592,0.500000000027091);
#757=ELLIPSE('',#15970,0.70710678118732,0.500000000000854);
#758=ELLIPSE('',#16016,1.11803398875074,0.500000000000357);
#759=ELLIPSE('',#16018,1.41421601068422,1.0000094568796);
#760=ELLIPSE('',#16021,1.39479172867192,0.980946657426322);
#761=ELLIPSE('',#16038,0.707106781186665,0.500000000000195);
#762=ELLIPSE('',#16039,1.1180335450767,0.999997604635691);
#763=ELLIPSE('',#16043,1.11805148063465,0.999999766049803);
#764=ELLIPSE('',#16058,1.11803398875087,0.500000000000499);
#765=ELLIPSE('',#16082,1.11810288856955,0.500019557827469);
#766=ELLIPSE('',#16083,1.41330852530877,0.999058658412993);
#767=ELLIPSE('',#16084,1.41330395373969,0.999062064731566);
#768=ELLIPSE('',#16145,0.541196100146381,0.500000000000179);
#769=ELLIPSE('',#16150,0.707106781202788,0.50000000002241);
#798=B_SPLINE_CURVE_WITH_KNOTS('',3,(#35181,#35182,#35183,#35184,#35185,
#35186,#35187,#35188,#35189,#35190,#35191,#35192,#35193,#35194,#35195,#35196),
 .UNSPECIFIED.,.F.,.F.,(4,2,2,2,2,2,2,4),(0.559306717359078,0.626396965369611,
0.735567235927107,0.809225982698514,0.832702121898874,0.841751773808283,
0.84754287435266,0.849323156359136),.UNSPECIFIED.);
#799=B_SPLINE_CURVE_WITH_KNOTS('',3,(#35198,#35199,#35200,#35201,#35202,
#35203,#35204,#35205,#35206,#35207,#35208,#35209,#35210,#35211,#35212,#35213,
#35214,#35215,#35216,#35217,#35218,#35219,#35220,#35221,#35222,#35223,#35224,
#35225),.UNSPECIFIED.,.F.,.F.,(4,2,2,1,1,1,2,2,2,1,1,1,2,2,1,1,1,1,4),(0.0040855928878666,
0.00415787795859431,0.00417749059047448,0.00419710322235465,0.004236328486115,
0.00431477901363569,0.00439322954115639,0.00443245480491673,0.00445206743679691,
0.00447168006867708,0.00455013059619778,0.00462858112371847,0.00470703165123916,
0.00472664428311934,0.00474625691499952,0.00478548217875988,0.00486393270628059,
0.0049423832338013,0.00499039171021971),.UNSPECIFIED.);
#800=B_SPLINE_CURVE_WITH_KNOTS('',3,(#35227,#35228,#35229,#35230,#35231,
#35232,#35233,#35234,#35235,#35236,#35237,#35238,#35239,#35240,#35241,#35242,
#35243,#35244,#35245,#35246,#35247,#35248,#35249,#35250,#35251,#35252,#35253,
#35254,#35255,#35256,#35257,#35258,#35259,#35260,#35261,#35262,#35263,#35264),
 .UNSPECIFIED.,.F.,.F.,(4,2,1,1,2,2,1,1,1,2,2,2,1,1,2,1,2,2,1,1,2,2,1,1,
4),(0.00499039171021971,0.00502083376132202,0.00509928428884266,0.0051777348163633,
0.00525618534388394,0.0052757979757641,0.00529541060764426,0.00533463587140458,
0.00541308639892522,0.00549153692644585,0.00551114955832601,0.00553076219020616,
0.00556998745396648,0.00564843798148711,0.00572688850900774,0.00576611377276805,
0.00578572640464821,0.00580533903652836,0.005883789564049,0.00596224009156964,
0.00604069061909029,0.0060799158828506,0.00611914114661092,0.00619759167413156,
0.00623984937653201),.UNSPECIFIED.);
#801=B_SPLINE_CURVE_WITH_KNOTS('',3,(#35266,#35267,#35268,#35269,#35270,
#35271,#35272,#35273,#35274,#35275,#35276,#35277,#35278,#35279,#35280,#35281,
#35282,#35283,#35284,#35285,#35286,#35287,#35288,#35289,#35290,#35291,#35292,
#35293,#35294,#35295,#35296,#35297,#35298,#35299,#35300,#35301,#35302,#35303,
#35304,#35305,#35306,#35307),.UNSPECIFIED.,.F.,.F.,(4,2,2,2,1,1,1,2,2,1,
1,1,2,2,2,1,1,1,2,2,1,1,1,2,2,2,4),(0.00121901561520999,0.00125520844033018,
0.0012944337040905,0.00131404633597066,0.00133365896785082,0.00141210949537145,
0.00149056002289208,0.00156901055041272,0.00158862318229288,0.00160823581417303,
0.00164746107793335,0.00172591160545398,0.00180436213297462,0.00184358739673493,
0.00186320002861509,0.00188281266049525,0.00196126318801588,0.00203971371553651,
0.00211816424305713,0.00213777687493729,0.00215738950681745,0.00219661477057776,
0.00227506529809839,0.00235351582561902,0.00239274108937934,0.00243196635313965,
0.0024802465217231),.UNSPECIFIED.);
#802=B_SPLINE_CURVE_WITH_KNOTS('',3,(#35309,#35310,#35311,#35312,#35313,
#35314,#35315,#35316,#35317,#35318,#35319,#35320,#35321,#35322,#35323,#35324,
#35325,#35326,#35327,#35328,#35329,#35330,#35331,#35332,#35333,#35334,#35335,
#35336,#35337,#35338,#35339,#35340,#35341),.UNSPECIFIED.,.F.,.F.,(4,2,2,
2,1,1,1,2,2,1,1,1,2,2,2,1,1,2,1,2,4),(0.0024802465217231,0.0025104168806603,
0.00254964214442063,0.0025692547763008,0.00258886740818097,0.00266731793570164,
0.00274576846322231,0.00282421899074298,0.00284383162262314,0.00286344425450331,
0.00290266951826364,0.0029811200457843,0.00305957057330496,0.00309879583706529,
0.00311840846894545,0.00313802110082561,0.00321647162834627,0.00329492215586693,
0.00333414741962726,0.00335376005150743,0.00337185540595827),
 .UNSPECIFIED.);
#803=B_SPLINE_CURVE_WITH_KNOTS('',3,(#35342,#35343,#35344,#35345,#35346,
#35347,#35348,#35349,#35350,#35351,#35352,#35353,#35354,#35355,#35356,#35357,
#35358,#35359,#35360),.UNSPECIFIED.,.F.,.F.,(4,2,2,2,2,2,2,3,4),(0.849323156359136,
0.852552467217484,0.858257321208267,0.867642993968765,0.889066342099187,
0.954635992312572,1.05821450691892,1.11775317676601,1.12218737820187),
 .UNSPECIFIED.);
#804=B_SPLINE_CURVE_WITH_KNOTS('',3,(#35370,#35371,#35372,#35373,#35374,
#35375,#35376,#35377,#35378,#35379,#35380,#35381,#35382,#35383,#35384,#35385,
#35386,#35387,#35388,#35389,#35390,#35391,#35392,#35393,#35394,#35395,#35396,
#35397,#35398,#35399,#35400,#35401,#35402,#35403,#35404,#35405,#35406,#35407,
#35408,#35409,#35410,#35411,#35412),.UNSPECIFIED.,.F.,.F.,(4,1,1,2,2,1,
1,1,2,2,2,1,1,1,2,2,1,1,1,2,2,2,1,2,2,2,1,4),(0.00133762907826533,0.00141171783679417,
0.00149014660550492,0.00156857537421566,0.00158818256639335,0.00160778975857103,
0.00164700414292642,0.0017254329116372,0.00180386168034798,0.00184307606470337,
0.00186268325688106,0.00188229044905876,0.00196071921776951,0.00203914798648025,
0.002117576755191,0.00213718394736868,0.00215679113954637,0.00219600552390173,
0.00227443429261245,0.00235286306132317,0.00239207744567853,0.00243129183003388,
0.00250972059874461,0.00258814936745533,0.0026273637518107,0.00266657813616607,
0.00274500690487681,0.00274775444653194),.UNSPECIFIED.);
#805=B_SPLINE_CURVE_WITH_KNOTS('',3,(#35414,#35415,#35416,#35417,#35418,
#35419,#35420,#35421,#35422,#35423,#35424,#35425,#35426,#35427,#35428,#35429,
#35430,#35431,#35432,#35433,#35434,#35435,#35436,#35437,#35438,#35439,#35440,
#35441,#35442,#35443,#35444,#35445,#35446,#35447,#35448,#35449,#35450),
 .UNSPECIFIED.,.F.,.F.,(4,2,2,1,1,1,2,2,2,1,2,1,2,2,1,1,2,2,2,1,1,2,4),
(0.00274775444653194,0.00282343567358756,0.00284304286576525,0.00286265005794293,
0.00290186444229832,0.00298029321100909,0.00305872197971986,0.00309793636407524,
0.00313715074843063,0.00321557951714139,0.00329400828585215,0.00333322267020754,
0.00335282986238522,0.00337243705456291,0.00345086582327365,0.0035292945919844,
0.00360772336069514,0.00362733055287283,0.00364693774505051,0.00368615212940588,
0.00376458089811663,0.00384300966682737,0.00384768372848343),
 .UNSPECIFIED.);
#806=B_SPLINE_CURVE_WITH_KNOTS('',3,(#35452,#35453,#35454,#35455,#35456,
#35457,#35458,#35459,#35460,#35461,#35462,#35463,#35464,#35465,#35466,#35467,
#35468,#35469,#35470,#35471,#35472,#35473,#35474,#35475,#35476,#35477,#35478,
#35479,#35480,#35481,#35482,#35483,#35484,#35485,#35486,#35487,#35488,#35489,
#35490,#35491,#35492,#35493,#35494,#35495,#35496),.UNSPECIFIED.,.F.,.F.,
(4,2,2,1,1,2,2,1,1,1,2,2,2,1,1,1,2,2,1,1,1,2,2,2,2,1,1,2,4),(0.00384768372848343,
0.00388222405118274,0.00392143843553811,0.00399986720424885,0.0040782959729596,
0.00415672474167034,0.00417633193384803,0.00419593912602572,0.0042351535103811,
0.00431358227909184,0.00439201104780258,0.00443122543215796,0.00445083262433565,
0.00447043981651334,0.0045488685852241,0.00462729735393486,0.00470572612264562,
0.00472533331482332,0.00474494050700101,0.00478415489135639,0.00486258366006715,
0.0049410124287779,0.00498022681313327,0.00499983400531096,0.00501944119748865,
0.00509786996619946,0.00517629873491028,0.0052547275036211,0.00525766866554466),
 .UNSPECIFIED.);
#807=B_SPLINE_CURVE_WITH_KNOTS('',3,(#35497,#35498,#35499,#35500,#35501,
#35502,#35503,#35504,#35505,#35506,#35507,#35508,#35509,#35510,#35511,#35512,
#35513,#35514,#35515,#35516,#35517,#35518,#35519,#35520,#35521,#35522,#35523,
#35524,#35525,#35526,#35527,#35528,#35529,#35530,#35531,#35532,#35533,#35534,
#35535,#35536,#35537),.UNSPECIFIED.,.F.,.F.,(4,2,1,1,1,2,2,2,1,1,2,1,2,
2,1,1,2,2,2,1,1,2,2,2,1,4),(0.000238227468056005,0.00025489349831015,0.000274500690487856,
0.000313715074843255,0.000392143843554055,0.000470572612264855,0.000509786996620253,
0.000529394188797954,0.000549001380975655,0.000627430149686458,0.000705858918397262,
0.00074507330275266,0.000764680494930355,0.000784287687108051,0.000862716455818834,
0.000941145224529618,0.0010195739932404,0.00103918118541809,0.00105878837759578,
0.00109800276195116,0.00117643153066191,0.00125486029937267,0.00129407468372805,
0.00131368187590574,0.00133328906808343,0.00133762907826533),
 .UNSPECIFIED.);
#808=B_SPLINE_CURVE_WITH_KNOTS('',3,(#35579,#35580,#35581,#35582,#35583,
#35584,#35585,#35586,#35587,#35588,#35589,#35590),.UNSPECIFIED.,.F.,.F.,
(4,2,2,2,2,4),(-0.479639825472432,-0.462425217556728,-0.422203417432446,
-0.38131877878649,-0.344677987741986,-0.318946577997265),.UNSPECIFIED.);
#809=B_SPLINE_CURVE_WITH_KNOTS('',3,(#35594,#35595,#35596,#35597,#35598,
#35599,#35600,#35601,#35602,#35603,#35604,#35605),.UNSPECIFIED.,.F.,.F.,
(4,2,2,2,2,4),(-0.318946577997265,-0.30962423887292,-0.272340183092938,
-0.230649804158065,-0.19116895139264,-0.158267505542008),.UNSPECIFIED.);
#810=B_SPLINE_CURVE_WITH_KNOTS('',3,(#35626,#35627,#35628,#35629,#35630,
#35631,#35632,#35633,#35634,#35635,#35636,#35637,#35638,#35639,#35640,#35641,
#35642,#35643),.UNSPECIFIED.,.F.,.F.,(4,2,2,2,2,2,2,2,4),(0.191281861861795,
0.215459032327926,0.239636202794058,0.259584872085487,0.279533541376917,
0.299482210668346,0.319430879959776,0.343608050425907,0.367785220892039),
 .UNSPECIFIED.);
#811=B_SPLINE_CURVE_WITH_KNOTS('',3,(#35649,#35650,#35651,#35652,#35653,
#35654,#35655,#35656,#35657,#35658,#35659,#35660,#35661,#35662,#35663,#35664,
#35665,#35666,#35667,#35668,#35669,#35670,#35671,#35672,#35673,#35674,#35675,
#35676,#35677),.UNSPECIFIED.,.F.,.F.,(4,2,2,2,2,2,2,2,1,2,2,2,1,1,2,4),
(6.50521303491303E-19,0.000157845345348291,0.000315690690696581,0.000473536036044871,
0.000552458708719019,0.000631381381393167,0.000789226726741468,0.000947072072089769,
0.00110491741743807,0.00126276276278637,0.00134168543546052,0.00142060810813467,
0.00157845345348297,0.00173629879883127,0.00189414414417957,0.00200452207066376),
 .UNSPECIFIED.);
#812=B_SPLINE_CURVE_WITH_KNOTS('',3,(#35679,#35680,#35681,#35682,#35683,
#35684,#35685,#35686,#35687,#35688,#35689,#35690,#35691,#35692,#35693,#35694,
#35695,#35696,#35697,#35698,#35699,#35700,#35701,#35702,#35703,#35704,#35705,
#35706,#35707,#35708,#35709,#35710,#35711,#35712,#35713,#35714,#35715),
 .UNSPECIFIED.,.F.,.F.,(4,3,3,3,3,3,3,3,3,3,3,3,4),(0.00200452207066376,
0.00220435629196357,0.00220983483487617,0.00236485788351544,0.00236768018022447,
0.0024451673964532,0.00244660285289862,0.00248533519715336,0.00248606418923569,
0.00250542216027589,0.00250579485740423,0.00251566019148849,0.00252552552557276),
 .UNSPECIFIED.);
#813=B_SPLINE_CURVE_WITH_KNOTS('',3,(#35721,#35722,#35723,#35724,#35725,
#35726),.UNSPECIFIED.,.F.,.F.,(4,2,4),(0.349196728876737,0.42160526861445,
0.509180501662979),.UNSPECIFIED.);
#814=B_SPLINE_CURVE_WITH_KNOTS('',3,(#35730,#35731,#35732,#35733,#35734,
#35735,#35736,#35737,#35738,#35739,#35740,#35741,#35742,#35743,#35744,#35745,
#35746,#35747,#35748,#35749,#35750,#35751,#35752,#35753,#35754,#35755,#35756,
#35757,#35758,#35759,#35760,#35761),.UNSPECIFIED.,.F.,.F.,(4,2,2,2,2,2,
2,2,2,2,2,2,2,2,2,4),(7.16841165822491E-9,0.00425984757262436,0.00882897338789379,
0.0181258595954712,0.0305987420002868,0.0373352764230015,0.0407040742822413,
0.0431630789194017,0.043233331588091,0.0457202883506083,0.0491738834305336,
0.055954122831043,0.0681757856187753,0.0771431840484888,0.0815121266890984,
0.0855915470562766),.UNSPECIFIED.);
#815=B_SPLINE_CURVE_WITH_KNOTS('',3,(#35771,#35772,#35773,#35774,#35775,
#35776,#35777,#35778,#35779,#35780,#35781,#35782,#35783,#35784),
 .UNSPECIFIED.,.F.,.F.,(4,2,2,2,2,2,4),(-0.0980600308872719,-0.0842479162203947,
-0.0683859734106203,-0.0469108894184264,-0.0242175938214273,0.,0.000471941323681861),
 .UNSPECIFIED.);
#816=B_SPLINE_CURVE_WITH_KNOTS('',3,(#35787,#35788,#35789,#35790,#35791,
#35792,#35793,#35794,#35795,#35796,#35797,#35798,#35799,#35800),
 .UNSPECIFIED.,.F.,.F.,(4,2,2,2,2,2,4),(-0.196928117070007,-0.196454849983009,
-0.172108534559874,-0.149310110641706,-0.127840368210239,-0.112006418277474,
-0.0982274249914714),.UNSPECIFIED.);
#817=B_SPLINE_CURVE_WITH_KNOTS('',3,(#35806,#35807,#35808,#35809,#35810,
#35811,#35812,#35813,#35814,#35815,#35816,#35817,#35818,#35819),
 .UNSPECIFIED.,.F.,.F.,(4,2,2,2,2,2,4),(0.101628267880583,0.107985189525145,
0.12609609523943,0.147834637699368,0.176750861538421,0.211678254053418,
0.212173672568657),.UNSPECIFIED.);
#818=B_SPLINE_CURVE_WITH_KNOTS('',3,(#35822,#35823,#35824,#35825,#35826,
#35827,#35828,#35829,#35830,#35831,#35832,#35833,#35834,#35835),
 .UNSPECIFIED.,.F.,.F.,(4,2,2,2,2,2,4),(-0.000412787679576289,0.,0.028368264114848,
0.0526479899563425,0.0709415556712408,0.0861626427766698,0.0917971386711219),
 .UNSPECIFIED.);
#819=B_SPLINE_CURVE_WITH_KNOTS('',3,(#35849,#35850,#35851,#35852,#35853,
#35854,#35855,#35856,#35857,#35858,#35859,#35860,#35861,#35862,#35863,#35864,
#35865,#35866,#35867,#35868,#35869,#35870,#35871,#35872,#35873,#35874,#35875,
#35876,#35877,#35878,#35879,#35880,#35881,#35882,#35883,#35884,#35885,#35886,
#35887,#35888,#35889,#35890,#35891,#35892,#35893,#35894,#35895,#35896,#35897,
#35898,#35899,#35900,#35901,#35902,#35903,#35904,#35905,#35906,#35907,#35908,
#35909,#35910,#35911,#35912,#35913,#35914,#35915,#35916,#35917,#35918,#35919,
#35920,#35921,#35922,#35923,#35924,#35925,#35926,#35927,#35928,#35929,#35930),
 .UNSPECIFIED.,.F.,.F.,(4,3,3,3,3,3,3,3,3,3,3,3,3,3,3,3,3,3,3,3,3,3,3,3,
3,3,3,4),(0.,5.46238072139918E-5,5.46768793257778E-5,0.000109353758651556,
0.000109437314960514,0.000218707517303111,0.000219131968308402,0.000328755035108541,
0.000437415034606219,0.000438315027410997,0.000656122551909328,0.000657273966688997,
0.000874830069212436,0.000876055977850079,0.00109353758651554,0.00109465839290278,
0.00131224510381865,0.0013130925134312,0.00153095262112176,0.00153141677949933,
0.00164030637977332,0.00164055507316062,0.00169498325909909,0.00169512122666045,
0.00172232169876198,0.00173599091859343,0.00174282552850915,0.00174966013842488),
 .UNSPECIFIED.);
#820=B_SPLINE_CURVE_WITH_KNOTS('',3,(#35932,#35933,#35934,#35935,#35936,
#35937,#35938,#35939,#35940,#35941,#35942,#35943,#35944,#35945,#35946,#35947,
#35948,#35949,#35950,#35951,#35952,#35953,#35954,#35955,#35956,#35957,#35958,
#35959,#35960,#35961,#35962,#35963,#35964,#35965,#35966,#35967,#35968,#35969,
#35970,#35971,#35972,#35973,#35974,#35975,#35976,#35977,#35978,#35979,#35980,
#35981,#35982,#35983,#35984,#35985,#35986,#35987,#35988,#35989,#35990,#35991,
#35992,#35993,#35994,#35995,#35996,#35997,#35998,#35999,#36000,#36001,#36002,
#36003,#36004,#36005,#36006,#36007,#36008,#36009,#36010,#36011,#36012,#36013),
 .UNSPECIFIED.,.F.,.F.,(4,3,3,3,3,3,3,3,3,3,3,3,3,3,3,3,3,3,3,3,3,3,3,3,
3,3,3,4),(-0.00174966013842491,-0.00174282552850919,-0.00173599091859347,
-0.00172232169876202,-0.00169512122666047,-0.00169498325909913,-0.00164055507316067,
-0.00164030637977336,-0.00153141677949938,-0.0015309526211218,-0.00131309251343127,
-0.00131224510381869,-0.00109465839290291,-0.00109353758651557,-0.000876055977850256,
-0.000874830069212459,-0.000657273966689205,-0.000656122551909345,-0.000438315027411205,
-0.000437415034606232,-0.000328755035108803,-0.000219131968308682,-0.000218707517303118,
-0.000109437314960775,-0.000109353758651561,-5.46768793257806E-5,-5.46238072142483E-5,
0.),.UNSPECIFIED.);
#821=B_SPLINE_CURVE_WITH_KNOTS('',3,(#36017,#36018,#36019,#36020,#36021,
#36022,#36023,#36024,#36025,#36026,#36027,#36028,#36029,#36030,#36031,#36032,
#36033,#36034,#36035,#36036,#36037,#36038,#36039,#36040,#36041,#36042,#36043,
#36044,#36045,#36046,#36047,#36048,#36049,#36050,#36051,#36052,#36053,#36054,
#36055,#36056),.UNSPECIFIED.,.F.,.F.,(4,3,3,3,3,3,3,3,3,3,3,3,3,4),(-0.00117485636691483,
-0.00113814210544875,-0.00110142784398266,-0.00102799932105048,-0.000881142275186127,
-0.000734285229321772,-0.000587428183457417,-0.000440571137593065,-0.000367142614660889,
-0.0003304283531948,-0.000293714091728711,-0.000146857045864357,-7.34285229321804E-5,
-3.03576608295941E-18),.UNSPECIFIED.);
#822=B_SPLINE_CURVE_WITH_KNOTS('',3,(#36062,#36063,#36064,#36065,#36066,
#36067,#36068,#36069,#36070,#36071),.UNSPECIFIED.,.F.,.F.,(4,2,2,2,4),(1.53451257034264E-7,
0.029053924592895,0.0610074471336537,0.12119991311449,0.121660810563458),
 .UNSPECIFIED.);
#823=B_SPLINE_CURVE_WITH_KNOTS('',3,(#36083,#36084,#36085,#36086,#36087,
#36088,#36089,#36090,#36091,#36092,#36093,#36094,#36095,#36096,#36097,#36098,
#36099,#36100),.UNSPECIFIED.,.F.,.F.,(4,2,2,2,2,2,2,2,4),(0.,0.0183029863676503,
0.0369119205731603,0.0559574729187805,0.0754931586326105,0.0951574217307725,
0.114505006447861,0.133267605428501,0.151453893017012),.UNSPECIFIED.);
#824=B_SPLINE_CURVE_WITH_KNOTS('',3,(#36104,#36105,#36106,#36107,#36108,
#36109,#36110,#36111,#36112,#36113,#36114,#36115,#36116,#36117),
 .UNSPECIFIED.,.F.,.F.,(4,2,2,2,2,2,4),(-0.000435818162108814,0.,0.0202992281610604,
0.039554052242145,0.0609562628819672,0.0778728931374231,0.0930628095475932),
 .UNSPECIFIED.);
#825=B_SPLINE_CURVE_WITH_KNOTS('',3,(#36122,#36123,#36124,#36125,#36126,
#36127,#36128,#36129,#36130,#36131,#36132,#36133),.UNSPECIFIED.,.F.,.F.,
(4,2,2,2,2,4),(0.142068886233636,0.167609243368551,0.19603253462721,0.222593243513583,
0.249806989712963,0.263543332734459),.UNSPECIFIED.);
#826=B_SPLINE_CURVE_WITH_KNOTS('',3,(#36161,#36162,#36163,#36164,#36165,
#36166,#36167,#36168,#36169,#36170,#36171,#36172,#36173,#36174,#36175,#36176,
#36177,#36178,#36179,#36180,#36181,#36182,#36183,#36184,#36185,#36186,#36187,
#36188,#36189,#36190,#36191,#36192,#36193,#36194,#36195,#36196,#36197,#36198,
#36199,#36200,#36201,#36202,#36203,#36204,#36205,#36206,#36207,#36208,#36209,
#36210,#36211,#36212,#36213,#36214,#36215,#36216,#36217,#36218,#36219,#36220,
#36221,#36222,#36223,#36224,#36225,#36226,#36227,#36228,#36229,#36230,#36231,
#36232,#36233,#36234,#36235,#36236,#36237,#36238,#36239,#36240,#36241,#36242,
#36243,#36244,#36245,#36246,#36247,#36248,#36249,#36250,#36251,#36252,#36253,
#36254,#36255,#36256,#36257,#36258,#36259,#36260,#36261,#36262,#36263,#36264,
#36265,#36266,#36267,#36268,#36269,#36270,#36271,#36272,#36273,#36274,#36275,
#36276,#36277,#36278,#36279,#36280,#36281,#36282,#36283,#36284,#36285,#36286,
#36287,#36288,#36289,#36290,#36291,#36292,#36293,#36294,#36295,#36296,#36297,
#36298,#36299,#36300,#36301,#36302,#36303,#36304,#36305,#36306,#36307,#36308,
#36309,#36310,#36311,#36312,#36313,#36314,#36315,#36316,#36317,#36318,#36319,
#36320,#36321,#36322,#36323,#36324,#36325,#36326,#36327,#36328,#36329,#36330,
#36331,#36332,#36333,#36334,#36335,#36336,#36337,#36338,#36339,#36340,#36341,
#36342,#36343,#36344),.UNSPECIFIED.,.F.,.F.,(4,3,3,3,3,3,3,3,3,3,3,3,3,
3,3,3,3,3,3,3,3,3,3,3,3,3,3,3,3,3,3,3,3,3,3,3,3,3,3,3,3,3,3,3,3,3,3,3,3,
3,3,3,3,3,3,3,3,3,3,3,3,4),(0.,0.000128793534426601,0.00013962725990874,
0.000201016480722258,0.000209440889863109,0.000237434536323755,0.000244347704840294,
0.000261801112328888,0.000274052527794055,0.000279254519817482,0.00041888177972623,
0.000421647685873793,0.000453788594703417,0.00045883099046583,0.000471242002192011,
0.000488695409680604,0.000496118975663363,0.000558509039634977,0.000570636153253297,
0.000698136299543724,0.000719219607406552,0.00073304311452091,0.000737751289965753,
0.000756269271015657,0.000767949929498096,0.000793191569626417,0.000837763559452467,
0.000866553502704528,0.000939320971633026,0.000975498896073627,0.00097739081936121,
0.000994844226849804,0.00101154198603956,0.0010122976343384,0.00104720444931558,
0.00111701807926996,0.00115415716089184,0.00125664533917869,0.00129450416296831,
0.00132645896913306,0.00132927157967002,0.00136136578411025,0.00136391871428646,
0.00139627259908743,0.00143289627153442,0.00153589985899619,0.00156968013137839,
0.00167552711890494,0.00170498962299591,0.00174534074885932,0.00177210055146248,
0.00178024756383651,0.00180552305617786,0.0018151543788137,0.00183887693334027,
0.00195478163872244,0.00197157657898437,0.00209440889863119,0.00210313115169305,
0.00212931571360838,0.00216422252858556,0.00223403615853994),
 .UNSPECIFIED.);
#827=B_SPLINE_CURVE_WITH_KNOTS('',3,(#36372,#36373,#36374,#36375,#36376,
#36377,#36378,#36379),.UNSPECIFIED.,.F.,.F.,(4,2,2,4),(-0.000445639589289738,
2.41755400420818E-15,0.0218391627722744,0.0289287082360094),
 .UNSPECIFIED.);
#828=B_SPLINE_CURVE_WITH_KNOTS('',3,(#36380,#36381,#36382,#36383,#36384,
#36385,#36386,#36387,#36388,#36389),.UNSPECIFIED.,.F.,.F.,(4,2,2,2,4),(0.411799298598375,
0.425924242071472,0.471726463519739,0.518409691411597,0.519022594153393),
 .UNSPECIFIED.);
#829=B_SPLINE_CURVE_WITH_KNOTS('',3,(#36393,#36394,#36395,#36396),
 .UNSPECIFIED.,.F.,.F.,(4,4),(-0.165567381125288,0.),.UNSPECIFIED.);
#830=B_SPLINE_CURVE_WITH_KNOTS('',3,(#36399,#36400,#36401,#36402,#36403,
#36404,#36405,#36406,#36407,#36408,#36409,#36410,#36411,#36412),
 .UNSPECIFIED.,.F.,.F.,(4,2,2,2,2,2,4),(0.0886615337454204,0.0907389095987879,
0.107041588865597,0.126817625016882,0.151565024549916,0.17449873389057,
0.174855361254283),.UNSPECIFIED.);
#831=B_SPLINE_CURVE_WITH_KNOTS('',3,(#36418,#36419,#36420,#36421,#36422,
#36423,#36424,#36425,#36426,#36427,#36428,#36429,#36430,#36431,#36432,#36433,
#36434,#36435,#36436,#36437,#36438,#36439,#36440,#36441,#36442,#36443,#36444,
#36445,#36446,#36447,#36448,#36449,#36450,#36451,#36452,#36453,#36454,#36455,
#36456,#36457,#36458,#36459,#36460,#36461,#36462,#36463,#36464,#36465,#36466,
#36467,#36468,#36469,#36470,#36471,#36472,#36473,#36474,#36475,#36476,#36477,
#36478,#36479,#36480,#36481,#36482,#36483,#36484,#36485,#36486,#36487,#36488,
#36489,#36490,#36491,#36492,#36493),.UNSPECIFIED.,.F.,.F.,(4,3,3,3,3,3,
3,3,3,3,3,3,3,3,3,3,3,3,3,3,3,3,3,3,3,4),(0.,9.73982238296995E-5,0.00019252004578257,
0.000194796447659399,0.000386060232528244,0.000389592895318797,0.00048315329443271,
0.000486991119148497,0.000531772924316341,0.000535690231063349,0.000560039787020775,
0.000580448963267321,0.000584389342978202,0.000776048112241012,0.000779185790637598,
0.000972895646006936,0.000973982238296993,0.00116877868595639,0.00117078841989245,
0.00126617690978609,0.0012700803416338,0.00131487602170093,0.00131980634716294,
0.00136357513361578,0.00136956336468157,0.00155837158127518),
 .UNSPECIFIED.);
#832=B_SPLINE_CURVE_WITH_KNOTS('',3,(#36494,#36495,#36496,#36497,#36498,
#36499,#36500,#36501,#36502,#36503,#36504,#36505,#36506,#36507,#36508,#36509,
#36510,#36511),.UNSPECIFIED.,.F.,.F.,(4,2,2,2,2,2,2,2,4),(-0.0823451520596356,
-0.0814641421114946,-0.079425143459902,-0.0765099977525957,-0.0745681831222406,
-0.0719848385051725,-0.0616691295558334,-0.0411719274467013,-9.99999319448164E-7),
 .UNSPECIFIED.);
#833=B_SPLINE_CURVE_WITH_KNOTS('',3,(#36513,#36514,#36515,#36516,#36517,
#36518,#36519,#36520,#36521,#36522,#36523,#36524,#36525,#36526,#36527,#36528,
#36529,#36530,#36531,#36532,#36533,#36534,#36535,#36536),.UNSPECIFIED.,
 .F.,.F.,(4,2,2,2,2,2,2,2,2,2,2,4),(-0.0818582793612237,-0.0408986769732426,
-0.0209173548870604,-0.0104500150359698,-0.00782862189102446,-0.00585645230784232,
-0.00289285619024227,-0.00141717783860899,-0.000679168113099727,-0.000303120243851664,
9.19584838832144E-10,7.57349769233838E-5),.UNSPECIFIED.);
#834=B_SPLINE_CURVE_WITH_KNOTS('',3,(#36538,#36539,#36540,#36541,#36542,
#36543,#36544,#36545,#36546,#36547,#36548,#36549,#36550,#36551,#36552,#36553,
#36554,#36555,#36556,#36557,#36558,#36559,#36560,#36561,#36562,#36563,#36564,
#36565,#36566,#36567,#36568,#36569,#36570,#36571,#36572,#36573,#36574,#36575,
#36576,#36577,#36578,#36579,#36580),.UNSPECIFIED.,.F.,.F.,(4,3,3,3,3,3,
3,3,3,3,3,3,3,3,4),(0.,0.000190596447604055,0.00024082472131754,0.00029102168932238,
0.000391254019785099,0.000589924182320116,0.00078656557642682,0.000983206970533523,
0.00100778714479686,0.00103236731906019,0.00108152766758686,0.0011798483646402,
0.00137648975874687,0.0014748104558002,0.00157313115285354),
 .UNSPECIFIED.);
#835=B_SPLINE_CURVE_WITH_KNOTS('',3,(#36586,#36587,#36588,#36589,#36590,
#36591,#36592,#36593,#36594,#36595),.UNSPECIFIED.,.F.,.F.,(4,2,2,2,4),(3.55271367880046E-15,
0.0721202303819016,0.0993400302468658,0.108173654477862,0.117007278708857),
 .UNSPECIFIED.);
#836=B_SPLINE_CURVE_WITH_KNOTS('',3,(#36613,#36614,#36615,#36616,#36617,
#36618,#36619,#36620,#36621,#36622,#36623,#36624,#36625,#36626,#36627,#36628,
#36629,#36630),.UNSPECIFIED.,.F.,.F.,(4,2,2,2,2,2,2,2,4),(-0.235513448497787,
-0.193326783450969,-0.151140118404152,-0.130797807210953,-0.117756724248895,
-0.104715641286835,-0.0843733300936382,-0.0421866650468191,0.),
 .UNSPECIFIED.);
#837=B_SPLINE_CURVE_WITH_KNOTS('',3,(#36636,#36637,#36638,#36639),
 .UNSPECIFIED.,.F.,.F.,(4,4),(0.000727522519127799,1.),.UNSPECIFIED.);
#838=B_SPLINE_CURVE_WITH_KNOTS('',3,(#36641,#36642,#36643,#36644,#36645,
#36646,#36647,#36648,#36649,#36650,#36651,#36652,#36653,#36654,#36655,#36656,
#36657,#36658,#36659,#36660,#36661,#36662,#36663,#36664,#36665,#36666,#36667,
#36668,#36669,#36670,#36671,#36672,#36673),.UNSPECIFIED.,.F.,.F.,(4,2,2,
1,2,2,2,1,1,1,2,2,2,2,2,1,2,2,4),(0.,0.0312500000000692,0.0468750000001036,
0.0546875000001194,0.0585937500001273,0.0625000000001351,0.125000000000152,
0.187500000000169,0.218750000000179,0.234375000000176,0.242187500000173,
0.250000000000169,0.375000000000013,0.437499999999922,0.468749999999877,
0.484374999999857,0.492187499999846,0.499999999999836,1.),.UNSPECIFIED.);
#839=B_SPLINE_CURVE_WITH_KNOTS('',3,(#36681,#36682,#36683,#36684,#36685,
#36686,#36687,#36688,#36689,#36690,#36691,#36692,#36693,#36694),
 .UNSPECIFIED.,.F.,.F.,(4,2,2,2,2,2,4),(-0.000385328305412479,1.70572106786282E-15,
0.0247793867166103,0.0515184272333669,0.0728860150158388,0.090500714324551,
0.092745274890908),.UNSPECIFIED.);
#840=B_SPLINE_CURVE_WITH_KNOTS('',3,(#36703,#36704,#36705,#36706,#36707,
#36708,#36709,#36710,#36711,#36712,#36713,#36714,#36715,#36716),
 .UNSPECIFIED.,.F.,.F.,(4,2,2,2,2,2,4),(-0.188304267635631,-0.187862880607499,
-0.166848428722395,-0.146905071719613,-0.125416885847754,-0.108754500181454,
-0.093931440303973),.UNSPECIFIED.);
#841=B_SPLINE_CURVE_WITH_KNOTS('',3,(#36719,#36720,#36721,#36722,#36723,
#36724,#36725,#36726,#36727,#36728,#36729,#36730,#36731,#36732),
 .UNSPECIFIED.,.F.,.F.,(4,2,2,2,2,2,4),(-0.0941733161862731,-0.079403572048281,
-0.0627829232813007,-0.0412936751319212,-0.02119709561475,0.,0.000443350791763836),
 .UNSPECIFIED.);
#842=B_SPLINE_CURVE_WITH_KNOTS('',3,(#36738,#36739,#36740,#36741,#36742,
#36743,#36744,#36745,#36746,#36747,#36748,#36749),.UNSPECIFIED.,.F.,.F.,
(4,2,2,2,2,4),(-0.000448819179553114,0.,0.0386802167200726,0.0689319278190867,
0.0909429437939334,0.108526726087003),.UNSPECIFIED.);
#843=B_SPLINE_CURVE_WITH_KNOTS('',3,(#36752,#36753,#36754,#36755,#36756,
#36757,#36758,#36759,#36760,#36761,#36762,#36763),.UNSPECIFIED.,.F.,.F.,
(4,2,2,2,2,4),(0.0962258393311769,0.110643300407674,0.128682242640802,0.153430032575363,
0.185007561669907,0.18537469972712),.UNSPECIFIED.);
#844=B_SPLINE_CURVE_WITH_KNOTS('',3,(#38300,#38301,#38302,#38303,#38304,
#38305,#38306,#38307,#38308,#38309,#38310,#38311,#38312,#38313,#38314,#38315,
#38316,#38317,#38318,#38319,#38320,#38321,#38322,#38323,#38324,#38325,#38326,
#38327,#38328,#38329,#38330,#38331,#38332,#38333,#38334,#38335,#38336,#38337,
#38338,#38339,#38340,#38341,#38342,#38343,#38344,#38345,#38346,#38347,#38348,
#38349,#38350,#38351,#38352,#38353,#38354,#38355,#38356,#38357,#38358,#38359,
#38360,#38361,#38362,#38363,#38364,#38365,#38366,#38367,#38368,#38369,#38370,
#38371,#38372,#38373,#38374,#38375,#38376,#38377,#38378,#38379,#38380,#38381,
#38382,#38383,#38384,#38385,#38386,#38387,#38388,#38389,#38390,#38391,#38392,
#38393,#38394,#38395,#38396,#38397,#38398,#38399,#38400,#38401,#38402,#38403,
#38404,#38405,#38406,#38407,#38408,#38409,#38410,#38411,#38412,#38413,#38414,
#38415,#38416,#38417,#38418,#38419,#38420,#38421,#38422,#38423,#38424,#38425,
#38426,#38427,#38428,#38429,#38430,#38431,#38432,#38433,#38434,#38435,#38436,
#38437,#38438,#38439,#38440,#38441,#38442,#38443,#38444,#38445,#38446,#38447,
#38448,#38449,#38450,#38451,#38452,#38453,#38454,#38455,#38456,#38457,#38458,
#38459,#38460,#38461,#38462,#38463,#38464,#38465,#38466,#38467,#38468,#38469,
#38470,#38471,#38472,#38473,#38474,#38475,#38476,#38477,#38478,#38479,#38480,
#38481,#38482,#38483,#38484,#38485,#38486,#38487,#38488,#38489,#38490,#38491,
#38492,#38493,#38494,#38495,#38496,#38497,#38498,#38499,#38500,#38501,#38502,
#38503,#38504,#38505,#38506,#38507,#38508,#38509,#38510,#38511,#38512,#38513),
 .UNSPECIFIED.,.F.,.F.,(4,3,3,3,3,3,3,3,3,3,3,3,3,3,3,3,3,3,3,3,3,3,3,3,
3,3,3,3,3,3,3,3,3,3,3,3,3,3,3,3,3,3,3,3,3,3,3,3,3,3,3,3,3,3,3,3,3,3,3,3,
3,3,3,3,3,3,3,3,3,3,3,4),(0.00181838839577617,0.00182764386550164,0.00184964353720942,
0.00187794335639532,0.00190763520719598,0.00190930945776452,0.00192250723231261,
0.00192422593790331,0.00193742583690015,0.00193914241804209,0.00196897537831967,
0.00199710160830158,0.00199880833859725,0.0020120204119779,0.00201372481873603,
0.00202693953123418,0.00202864129887482,0.00205677738648887,0.00208830721942998,
0.00211645310942199,0.00211814017970755,0.00212391258051836,0.00213137205065051,
0.00213305665984635,0.00214629098961237,0.00214797313998514,0.00217612888023953,
0.00220596674733626,0.00220763906054031,0.0022208856864302,0.0022225555406791,
0.00222834514776207,0.00223580462220084,0.0022374720208179,0.00226730498109548,
0.00229547760561947,0.00232531799373752,0.00232697090165065,0.00234023727065812,
0.00234188738178944,0.00235515613654191,0.00235680386192822,0.00238663682220578,
0.00241483189593419,0.00241646978248335,0.00242975087335353,0.00243138626262213,
0.00244466977649174,0.00244630274276092,0.00247450763036943,0.00250596866331607,
0.00253418361230688,0.00253580162359365,0.0025416420294745,0.00254910146409367,
0.00256402127173024,0.00256563458387123,0.00259385882465156,0.00262369701173162,
0.00262530050442639,0.00263861585880305,0.00264021698456519,0.00265353488839818,
0.00265513346470398,0.00268496642498156,0.00271321069336538,0.00271479938525913,
0.00272812950694487,0.00272971586539792,0.00274304860630799,0.00274463234553671,
0.00277288643986402),.UNSPECIFIED.);
#845=B_SPLINE_CURVE_WITH_KNOTS('',3,(#38962,#38963,#38964,#38965,#38966,
#38967,#38968,#38969,#38970,#38971,#38972,#38973,#38974,#38975,#38976,#38977,
#38978,#38979,#38980,#38981,#38982,#38983,#38984,#38985,#38986,#38987,#38988,
#38989,#38990,#38991,#38992,#38993,#38994,#38995,#38996,#38997,#38998,#38999,
#39000,#39001,#39002,#39003,#39004,#39005,#39006,#39007,#39008,#39009,#39010,
#39011,#39012,#39013,#39014,#39015,#39016,#39017,#39018,#39019,#39020,#39021,
#39022,#39023,#39024,#39025,#39026,#39027,#39028,#39029,#39030,#39031,#39032,
#39033,#39034,#39035,#39036,#39037,#39038,#39039,#39040,#39041,#39042,#39043,
#39044,#39045,#39046,#39047,#39048,#39049,#39050,#39051,#39052,#39053,#39054,
#39055,#39056,#39057,#39058,#39059,#39060,#39061,#39062,#39063,#39064,#39065,
#39066,#39067,#39068,#39069,#39070,#39071,#39072,#39073,#39074,#39075,#39076,
#39077,#39078,#39079,#39080,#39081,#39082,#39083,#39084,#39085,#39086,#39087,
#39088,#39089,#39090,#39091,#39092,#39093,#39094,#39095,#39096,#39097,#39098,
#39099,#39100,#39101,#39102,#39103,#39104,#39105,#39106,#39107,#39108,#39109,
#39110,#39111,#39112,#39113,#39114,#39115,#39116,#39117,#39118,#39119,#39120,
#39121,#39122,#39123,#39124,#39125,#39126,#39127,#39128,#39129,#39130,#39131,
#39132,#39133,#39134,#39135,#39136,#39137,#39138,#39139,#39140,#39141,#39142,
#39143,#39144,#39145,#39146,#39147,#39148,#39149,#39150,#39151,#39152,#39153,
#39154,#39155,#39156,#39157,#39158,#39159,#39160,#39161,#39162,#39163,#39164,
#39165,#39166,#39167,#39168,#39169,#39170,#39171,#39172,#39173,#39174,#39175),
 .UNSPECIFIED.,.F.,.F.,(4,3,3,3,3,3,3,3,3,3,3,3,3,3,3,3,3,3,3,3,3,3,3,3,
3,3,3,3,3,3,3,3,3,3,3,3,3,3,3,3,3,3,3,3,3,3,3,3,3,3,3,3,3,3,3,3,3,3,3,3,
3,3,3,3,3,3,3,3,3,3,3,4),(1.16051834735224E-5,1.493476621997E-5,2.986953243994E-5,
4.14803381536968E-5,5.973906487988E-5,7.13545593270396E-5,8.960859731982E-5,
0.00010122861902708,0.000104543363539795,0.000116165788001039,0.00011947812975977,
0.000131102516262791,0.00017921719463969,0.000190851997707725,0.000209086727079646,
0.000220725563339751,0.000224021493299624,0.000238956259519601,0.000250599218308967,
0.000298695324399528,0.000310347338597952,0.000313630090619511,0.000325284880712085,
0.000328564856839494,0.000340221602554756,0.000358434389279461,0.00037009570634431,
0.000399969818859634,0.000414906878365008,0.000418173454159394,0.000422375399610592,
0.000429843922048107,0.000433108220379377,0.000448042986599361,0.000477912519039327,
0.000489592134427833,0.000507782051479294,0.000519466263512958,0.000522716817699277,
0.000534403777182626,0.00053765158391926,0.000549340376544938,0.000597390648799192,
0.000609090041569225,0.000624026559493112,0.00062726018123916,0.00063896232213999,
0.000642194947459142,0.000657129713679124,0.000668836802496252,0.000716868778559061,
0.000728584194058549,0.000731803544779041,0.000743521593993477,0.00074673831099902,
0.000758459202638857,0.000776607843438971,0.000788333309895947,0.000806477375878921,
0.000818207334889621,0.000821412142098897,0.000833144688766855,0.000836346908318872,
0.000848081531617883,0.000896085973198773,0.000907828831845864,0.000922766520025946,
0.000925955505638724,0.000937704197704619,0.000940890271858694,0.000955825038078664,
0.000967577998166243),.UNSPECIFIED.);
#846=B_SPLINE_CURVE_WITH_KNOTS('',3,(#39182,#39183,#39184,#39185,#39186,
#39187,#39188,#39189,#39190,#39191,#39192,#39193,#39194,#39195,#39196,#39197,
#39198,#39199,#39200,#39201,#39202,#39203,#39204,#39205,#39206,#39207,#39208,
#39209,#39210,#39211,#39212,#39213,#39214,#39215,#39216,#39217,#39218,#39219,
#39220,#39221,#39222,#39223,#39224,#39225,#39226,#39227,#39228,#39229,#39230,
#39231,#39232,#39233,#39234,#39235,#39236,#39237,#39238,#39239,#39240,#39241,
#39242,#39243,#39244,#39245,#39246,#39247,#39248,#39249,#39250,#39251,#39252,
#39253,#39254,#39255,#39256,#39257,#39258,#39259,#39260,#39261,#39262,#39263,
#39264,#39265,#39266,#39267,#39268,#39269,#39270,#39271,#39272,#39273,#39274,
#39275,#39276,#39277,#39278,#39279,#39280,#39281,#39282,#39283,#39284,#39285,
#39286,#39287,#39288,#39289,#39290,#39291,#39292,#39293,#39294,#39295,#39296,
#39297,#39298,#39299,#39300,#39301,#39302,#39303,#39304,#39305,#39306,#39307,
#39308,#39309,#39310,#39311,#39312,#39313,#39314,#39315,#39316,#39317,#39318,
#39319,#39320,#39321,#39322,#39323,#39324,#39325,#39326,#39327,#39328,#39329,
#39330,#39331,#39332,#39333,#39334,#39335,#39336,#39337,#39338,#39339,#39340,
#39341,#39342,#39343,#39344,#39345,#39346,#39347,#39348,#39349,#39350,#39351,
#39352,#39353,#39354,#39355,#39356,#39357,#39358,#39359,#39360,#39361,#39362,
#39363,#39364,#39365,#39366,#39367,#39368,#39369,#39370,#39371,#39372,#39373,
#39374,#39375,#39376,#39377,#39378,#39379,#39380,#39381,#39382,#39383),
 .UNSPECIFIED.,.F.,.F.,(4,3,3,3,3,3,3,3,3,3,3,3,3,3,3,3,3,3,3,3,3,3,3,3,
3,3,3,3,3,3,3,3,3,3,3,3,3,3,3,3,3,3,3,3,3,3,3,3,3,3,3,3,3,3,3,3,3,3,3,3,
3,3,3,3,3,3,3,4),(0.000863576982099504,0.000893415377688714,0.000894988808327375,
0.000908326951236741,0.000923246281154781,0.000954654728882556,0.000982928494721109,
0.000984487689160143,0.00099784771503611,0.000999404169298931,0.00101276621276172,
0.00101432064943772,0.0010426043099559,0.00107398656999286,0.00110228001659828,
0.00110381953027044,0.0011321178395976,0.00113365249054802,0.00116195519971085,
0.00119179359098349,0.00119331841110319,0.00120671253144932,0.00120823489124197,
0.00122163150653409,0.00122315137138076,0.00125298433165833,0.00128130729281906,
0.00128281729193591,0.00129622608400764,0.00129773377207469,0.00131114520917519,
0.00131265025221348,0.00134098306403575,0.00137231617276862,0.0014006587939414,
0.00140214913304619,0.0014081182647691,0.00141557773488575,0.00141706561318497,
0.00143049667390546,0.00143198209332375,0.00146033456285987,0.00149017243153675,
0.00149164801387886,0.00150509127393628,0.00150656449401764,0.00152001034775925,
0.00152148097415642,0.00155131393443396,0.00157968447035871,0.00160952384680422,
0.00161097985498904,0.0016169840698581,0.00162444291082146,0.00162589633512782,
0.00163936182129664,0.00164081281526659,0.00167064577554414,0.00169903758015923,
0.00170047873582169,0.00171395651569461,0.00172887545911729,0.00173031169609923,
0.0017587131784449,0.00178855120104918,0.00178997761665432,0.0018048940967931,
0.00181838839577617),.UNSPECIFIED.);
#847=B_SPLINE_CURVE_WITH_KNOTS('',3,(#39828,#39829,#39830,#39831,#39832,
#39833,#39834,#39835,#39836,#39837,#39838,#39839,#39840,#39841,#39842,#39843,
#39844,#39845,#39846,#39847,#39848,#39849,#39850,#39851,#39852,#39853,#39854,
#39855,#39856,#39857,#39858,#39859,#39860,#39861,#39862,#39863,#39864,#39865,
#39866,#39867,#39868,#39869,#39870,#39871,#39872,#39873,#39874,#39875,#39876,
#39877,#39878,#39879,#39880,#39881,#39882,#39883,#39884,#39885,#39886,#39887,
#39888,#39889,#39890,#39891,#39892,#39893,#39894,#39895,#39896,#39897,#39898,
#39899,#39900,#39901,#39902,#39903,#39904,#39905,#39906,#39907,#39908,#39909,
#39910,#39911,#39912,#39913,#39914,#39915,#39916,#39917,#39918,#39919,#39920,
#39921,#39922,#39923,#39924,#39925,#39926,#39927,#39928,#39929,#39930,#39931,
#39932,#39933,#39934,#39935,#39936,#39937,#39938,#39939,#39940,#39941,#39942,
#39943,#39944,#39945,#39946,#39947,#39948,#39949,#39950,#39951,#39952,#39953,
#39954,#39955,#39956,#39957,#39958,#39959,#39960,#39961,#39962,#39963,#39964,
#39965,#39966,#39967,#39968,#39969,#39970,#39971,#39972,#39973,#39974,#39975,
#39976,#39977,#39978,#39979,#39980,#39981,#39982,#39983,#39984,#39985,#39986,
#39987,#39988,#39989,#39990,#39991,#39992,#39993,#39994,#39995,#39996,#39997,
#39998,#39999,#40000,#40001,#40002,#40003,#40004,#40005,#40006,#40007,#40008,
#40009,#40010,#40011,#40012,#40013,#40014,#40015,#40016,#40017,#40018,#40019,
#40020,#40021,#40022,#40023,#40024,#40025,#40026,#40027,#40028,#40029,#40030,
#40031,#40032,#40033,#40034,#40035,#40036,#40037,#40038),.UNSPECIFIED.,
 .F.,.F.,(4,3,3,3,3,3,3,3,3,3,3,3,3,3,3,3,3,3,3,3,3,3,3,3,3,3,3,3,3,3,3,
3,3,3,3,3,3,3,3,3,3,3,3,3,3,3,3,3,3,3,3,3,3,3,3,3,3,3,3,3,3,3,3,3,3,3,3,
3,3,3,4),(0.000967577998166243,0.000985694570518615,0.000997452104970326,
0.00101238917013626,0.00101556410295857,0.00102732620518103,0.00107530316783846,
0.00108707491923346,0.00110201144791451,0.0011051727002784,0.00110947846831176,
0.00111694691155728,0.00113504223271835,0.00114682263399536,0.00119478129759824,
0.00120657015384326,0.00120971606381822,0.00122150734177849,0.0012246508300382,
0.00123644503461287,0.00125452036247816,0.0012663191435441,0.00128438989491812,
0.00129619324251587,0.00129932466113811,0.00131112984419676,0.00131425942735809,
0.00132606550487095,0.00137399849223803,0.0013858155767176,0.00140075265939606,
0.00140386802467799,0.0014082211872552,0.00141568971683767,0.00141880279089798,
0.00143373755711796,0.00144556379707782,0.00149347662199789,0.00150531189682198,
0.00150841138821788,0.0015202496101457,0.00152334615443786,0.00153518618508574,
0.00155321568687783,0.00156506022979621,0.00159493423161199,0.00160987166971053,
0.00161295475175777,0.00162480857197639,0.00162788951797776,0.00164282428419775,
0.00167269381663772,0.00168455672937543,0.00170256334907769,0.00171443152813003,
0.00171749811529767,0.00172189869624108,0.00172936775988772,0.00173243288151765,
0.00174430495412123,0.00179217194639758,0.00180405320053485,0.00180710671261757,
0.00181898963002168,0.00182204147883755,0.0018339180528411,0.00185191101127753,
0.00186374210842334,0.00189350855411201,0.00191165007615749,0.00192325525963101),
 .UNSPECIFIED.);
#848=B_SPLINE_CURVE_WITH_KNOTS('',3,(#41383,#41384,#41385,#41386,#41387,
#41388,#41389,#41390,#41391,#41392,#41393,#41394,#41395,#41396,#41397,#41398),
 .UNSPECIFIED.,.F.,.F.,(4,2,2,2,2,2,2,4),(-0.00044779014185856,0.,0.0229409691169892,
0.0448607972358344,0.0664784333744104,0.0823924396306553,0.0961964805679204,
0.0962258393298038),.UNSPECIFIED.);
#849=B_SPLINE_CURVE_WITH_KNOTS('',3,(#41401,#41402,#41403,#41404,#41405,
#41406,#41407,#41408,#41409,#41410,#41411,#41412),.UNSPECIFIED.,.F.,.F.,
(4,2,2,2,2,4),(0.0963708477811746,0.110766905123989,0.128787592759141,0.15355503814959,
0.185223004044538,0.185590457789025),.UNSPECIFIED.);
#850=B_SPLINE_CURVE_WITH_KNOTS('',3,(#41417,#41418,#41419,#41420,#41421,
#41422,#41423,#41424,#41425,#41426,#41427,#41428,#41429,#41430),
 .UNSPECIFIED.,.F.,.F.,(4,2,2,2,2,2,4),(-0.0939314403051867,-0.0791083804274454,
-0.062445994760847,-0.0409578088886071,-0.0210144518854656,-2.88935542158697E-14,
0.000441387027557035),.UNSPECIFIED.);
#851=B_SPLINE_CURVE_WITH_KNOTS('',3,(#41433,#41434,#41435,#41436,#41437,
#41438,#41439,#41440,#41441,#41442,#41443,#41444,#41445,#41446),
 .UNSPECIFIED.,.F.,.F.,(4,2,2,2,2,2,4),(-0.188789983926297,-0.188346633130585,
-0.167149537440147,-0.147052957839446,-0.125563709600744,-0.108943060764686,
-0.0941733165652966),.UNSPECIFIED.);
#852=B_SPLINE_CURVE_WITH_KNOTS('',3,(#41454,#41455,#41456,#41457,#41458,
#41459,#41460,#41461,#41462,#41463,#41464,#41465,#41466,#41467),
 .UNSPECIFIED.,.F.,.F.,(4,2,2,2,2,2,4),(-0.210772012984322,-0.210280903065,
-0.177423583499178,-0.148314265031791,-0.126331471038667,-0.108064160223483,
-0.100943721292222),.UNSPECIFIED.);
#853=B_SPLINE_CURVE_WITH_KNOTS('',3,(#41471,#41472,#41473,#41474,#41475,
#41476,#41477,#41478,#41479,#41480,#41481,#41482,#41483,#41484),
 .UNSPECIFIED.,.F.,.F.,(4,2,2,2,2,2,4),(-0.000412787679576566,0.,0.0283682641149075,
0.0526479899564725,0.0709415556714253,0.0861626427768875,0.0917971386713504),
 .UNSPECIFIED.);
#854=B_SPLINE_CURVE_WITH_KNOTS('',3,(#41635,#41636,#41637,#41638,#41639,
#41640,#41641,#41642,#41643,#41644),.UNSPECIFIED.,.F.,.F.,(4,2,2,2,4),(-0.00349842735434734,
-2.74352589257898E-12,0.0521414590439604,0.0796329571011274,0.104846643196789),
 .UNSPECIFIED.);
#855=B_SPLINE_CURVE_WITH_KNOTS('',3,(#41800,#41801,#41802,#41803,#41804,
#41805,#41806,#41807,#41808,#41809,#41810,#41811,#41812,#41813,#41814,#41815,
#41816,#41817,#41818,#41819,#41820,#41821,#41822,#41823,#41824,#41825,#41826,
#41827,#41828,#41829,#41830,#41831,#41832,#41833,#41834,#41835,#41836,#41837,
#41838,#41839,#41840,#41841,#41842,#41843,#41844,#41845,#41846,#41847,#41848,
#41849,#41850,#41851,#41852,#41853,#41854,#41855,#41856,#41857,#41858,#41859,
#41860,#41861,#41862,#41863,#41864,#41865,#41866,#41867,#41868,#41869,#41870,
#41871,#41872,#41873,#41874,#41875,#41876,#41877,#41878,#41879,#41880,#41881,
#41882,#41883,#41884,#41885,#41886,#41887,#41888,#41889,#41890,#41891,#41892,
#41893,#41894,#41895,#41896,#41897,#41898,#41899,#41900,#41901,#41902,#41903,
#41904,#41905,#41906,#41907,#41908,#41909,#41910,#41911,#41912,#41913,#41914,
#41915,#41916,#41917,#41918,#41919,#41920,#41921,#41922,#41923,#41924,#41925,
#41926,#41927,#41928,#41929,#41930,#41931,#41932,#41933,#41934,#41935,#41936,
#41937,#41938,#41939,#41940,#41941,#41942,#41943,#41944,#41945,#41946,#41947,
#41948,#41949,#41950,#41951,#41952,#41953),.UNSPECIFIED.,.F.,.F.,(4,3,3,
3,3,3,3,3,3,3,3,3,3,3,3,3,3,3,3,3,3,3,3,3,3,3,3,3,3,3,3,3,3,3,3,3,3,3,3,
3,3,3,3,3,3,3,3,3,3,3,3,4),(0.,3.75072506682356E-5,6.03395682026754E-5,
7.50145013364712E-5,8.43913140035302E-5,9.37681266705891E-5,0.000112521752004707,
0.000118020145270055,0.000131275377338824,0.000132487485027507,0.000147073827762125,
0.000150029002672942,0.000176606237268957,0.000187536253341185,0.000206289878675303,
0.000225043504009422,0.000237243896542391,0.00024379712934354,0.000253016586246074,
0.000262550754677658,0.000269091009696469,0.000300058005345894,0.000302111818529164,
0.000337565256014129,0.000371377991455727,0.000375072506682365,0.000393826132016483,
0.000407518571944512,0.000412579757350601,0.000444600452064642,0.000450087008018838,
0.000515403930086837,0.000521321544297857,0.000525101509355314,0.00060011601069179,
0.000601142173193074,0.000621551460391748,0.000637623261360026,0.00064212154415199,
0.000675130512028263,0.00068361343341191,0.000750145013364734,0.000767896109444578,
0.000853794321857111,0.000900174016037677,0.000941224992165524,0.000975188517374148,
0.000985498887476787,0.00101269576804238,0.00103003827125258,0.00105020301871062,
0.00120023202138355),.UNSPECIFIED.);
#856=B_SPLINE_CURVE_WITH_KNOTS('',3,(#41971,#41972,#41973,#41974,#41975,
#41976,#41977,#41978,#41979,#41980,#41981,#41982,#41983,#41984),
 .UNSPECIFIED.,.F.,.F.,(4,2,2,2,2,2,4),(0.0886615337472132,0.0907389096006223,
0.107041588867765,0.126817625019457,0.151565024553096,0.174498733894337,
0.174855361258075),.UNSPECIFIED.);
#857=B_SPLINE_CURVE_WITH_KNOTS('',3,(#41986,#41987,#41988,#41989,#41990,
#41991,#41992,#41993,#41994,#41995),.UNSPECIFIED.,.F.,.F.,(4,2,2,2,4),(0.0745079449586904,
0.0933896612732089,0.112173398676393,0.130768592867116,0.149172319853601),
 .UNSPECIFIED.);
#858=B_SPLINE_CURVE_WITH_KNOTS('',3,(#42017,#42018,#42019,#42020,#42021,
#42022,#42023,#42024,#42025,#42026,#42027,#42028,#42029,#42030),
 .UNSPECIFIED.,.F.,.F.,(4,2,2,2,2,2,4),(0.0886615337459981,0.0907389095993787,
0.107041588866303,0.126817625017728,0.151565024551055,0.174498733892164,
0.174855361255883),.UNSPECIFIED.);
#859=B_SPLINE_CURVE_WITH_KNOTS('',3,(#42235,#42236,#42237,#42238,#42239,
#42240,#42241,#42242,#42243,#42244,#42245,#42246,#42247,#42248,#42249,#42250,
#42251,#42252,#42253,#42254,#42255,#42256,#42257,#42258,#42259,#42260,#42261,
#42262,#42263,#42264,#42265,#42266,#42267,#42268,#42269,#42270,#42271,#42272,
#42273,#42274,#42275,#42276,#42277,#42278,#42279,#42280,#42281,#42282,#42283,
#42284,#42285,#42286,#42287,#42288,#42289,#42290,#42291,#42292,#42293,#42294,
#42295,#42296,#42297,#42298,#42299,#42300,#42301,#42302,#42303,#42304,#42305,
#42306,#42307,#42308,#42309,#42310,#42311,#42312,#42313,#42314,#42315,#42316,
#42317,#42318,#42319,#42320,#42321,#42322,#42323,#42324,#42325,#42326,#42327,
#42328,#42329,#42330,#42331,#42332,#42333,#42334,#42335,#42336,#42337,#42338,
#42339,#42340,#42341,#42342,#42343,#42344,#42345,#42346,#42347,#42348,#42349,
#42350,#42351,#42352,#42353,#42354,#42355,#42356,#42357,#42358,#42359,#42360,
#42361,#42362,#42363,#42364,#42365,#42366,#42367,#42368,#42369,#42370,#42371,
#42372,#42373,#42374,#42375,#42376,#42377,#42378,#42379,#42380,#42381,#42382,
#42383,#42384,#42385,#42386,#42387,#42388,#42389,#42390,#42391,#42392,#42393,
#42394,#42395,#42396,#42397),.UNSPECIFIED.,.F.,.F.,(4,3,3,3,3,3,3,3,3,3,
3,3,3,3,3,3,3,3,3,3,3,3,3,3,3,3,3,3,3,3,3,3,3,3,3,3,3,3,3,3,3,3,3,3,3,3,
3,3,3,3,3,3,3,3,4),(0.,0.0340147436347705,0.0796654100921325,0.121150235206392,
0.16258274933431,0.189677904438364,0.227859710016422,0.242187499996718,
0.246836013781419,0.249999999996616,0.288220212410142,0.311288214891701,
0.34470470346921,0.365172426794162,0.371093749995032,0.374999999994983,
0.389696018730405,0.405679200193564,0.409288359158387,0.427230980167802,
0.433593749994273,0.437208894920299,0.437499999994228,0.45349495870215,
0.466556751031909,0.482527649839429,0.49804687499366,0.499999999993643,
0.514675935726806,0.526075117753044,0.542334433873725,0.556301931927462,
0.558593749994405,0.561295009043853,0.562499999994452,0.567510296898257,
0.597538662312543,0.60937499999504,0.619397988471943,0.624837579898199,
0.624999999995238,0.657086602514375,0.68282993630191,0.717724404284978,
0.742187499996745,0.747700569938847,0.749999999996844,0.751088206824535,
0.783457115912507,0.818040475412505,0.860724294573825,0.904220867740056,
0.952110414151086,0.994093280424259,0.999999960562115),.UNSPECIFIED.);
#860=B_SPLINE_CURVE_WITH_KNOTS('',3,(#42399,#42400,#42401,#42402,#42403,
#42404,#42405,#42406),.UNSPECIFIED.,.F.,.F.,(4,2,2,4),(-0.000330927471132683,
-4.60980603380267E-9,0.0122588170368006,0.0209462363748979),
 .UNSPECIFIED.);
#861=B_SPLINE_CURVE_WITH_KNOTS('',3,(#42518,#42519,#42520,#42521,#42522,
#42523,#42524,#42525,#42526,#42527,#42528,#42529,#42530,#42531,#42532,#42533,
#42534,#42535,#42536,#42537,#42538,#42539,#42540,#42541,#42542,#42543,#42544,
#42545,#42546,#42547,#42548,#42549,#42550,#42551,#42552,#42553,#42554,#42555,
#42556,#42557,#42558,#42559,#42560),.UNSPECIFIED.,.F.,.F.,(4,3,3,3,3,3,
3,3,3,3,3,3,3,3,4),(0.,0.083607507194038,0.166803753597019,0.25,0.328236652674478,
0.406218055000426,0.484054848510691,0.5,0.578122914091021,0.656344013643421,
0.734920106325271,0.75,0.834722429329149,0.92066309428102,0.999999651298147),
 .UNSPECIFIED.);
#862=B_SPLINE_CURVE_WITH_KNOTS('',3,(#42643,#42644,#42645,#42646,#42647,
#42648,#42649,#42650,#42651,#42652,#42653,#42654,#42655,#42656,#42657,#42658,
#42659,#42660,#42661,#42662,#42663,#42664,#42665),.UNSPECIFIED.,.F.,.F.,
(4,1,1,1,2,2,2,2,2,1,1,2,2,4),(6.31448876631291E-18,0.000104906811635738,
0.000209813623271469,0.000314720434907201,0.000419627246542932,0.000524534058178664,
0.00057698746399653,0.000629440869814395,0.000734347681450129,0.000786801087267997,
0.000813027790176931,0.000826141141631399,0.00083269781735863,0.000839254493085862),
 .UNSPECIFIED.);
#863=B_SPLINE_CURVE_WITH_KNOTS('',3,(#42666,#42667,#42668,#42669,#42670,
#42671,#42672,#42673,#42674,#42675,#42676,#42677,#42678,#42679,#42680,#42681),
 .UNSPECIFIED.,.F.,.F.,(4,2,2,2,2,2,2,4),(0.,0.000213634091527792,0.00026704261440974,
0.000320451137291689,0.00042726818305558,0.000640902274583368,0.000747719320347264,
0.000854536366111159),.UNSPECIFIED.);
#864=B_SPLINE_CURVE_WITH_KNOTS('',3,(#42764,#42765,#42766,#42767,#42768,
#42769,#42770,#42771,#42772,#42773,#42774,#42775,#42776,#42777,#42778,#42779,
#42780,#42781,#42782,#42783,#42784,#42785,#42786,#42787,#42788,#42789,#42790,
#42791,#42792,#42793,#42794,#42795,#42796,#42797,#42798,#42799,#42800,#42801,
#42802,#42803,#42804,#42805,#42806,#42807,#42808,#42809,#42810,#42811,#42812,
#42813,#42814,#42815,#42816,#42817,#42818,#42819,#42820,#42821,#42822,#42823,
#42824,#42825,#42826,#42827,#42828,#42829,#42830,#42831,#42832,#42833,#42834,
#42835,#42836,#42837,#42838,#42839,#42840,#42841,#42842,#42843,#42844,#42845,
#42846,#42847,#42848),.UNSPECIFIED.,.F.,.F.,(4,3,3,3,3,3,3,3,3,3,3,3,3,
3,3,3,3,3,3,3,3,3,3,3,3,3,3,3,4),(-0.00084007102973227,-0.000833507974812657,
-0.00082694491989287,-0.000813818810053298,-0.000799319178203659,-0.000787566590374158,
-0.000757799963646104,-0.000735062151015878,-0.000673123074247421,-0.000630053272299322,
-0.000586475425630851,-0.000525044393582767,-0.000497658838514586,-0.000472539954224489,
-0.000420035514866211,-0.000335812876675837,-0.000315026636149658,-0.000310877818697253,
-0.000232328685341806,-0.000210017757433106,-0.000137430443904471,-0.000107807929015954,
-0.000105008878716553,-5.25044393582766E-5,-2.62522196791383E-5,-1.31261098395691E-5,
-6.56305491978457E-6,-3.28152745989229E-6,0.),.UNSPECIFIED.);
#865=B_SPLINE_CURVE_WITH_KNOTS('',3,(#42849,#42850,#42851,#42852,#42853,
#42854,#42855,#42856,#42857,#42858,#42859,#42860,#42861,#42862,#42863),
 .UNSPECIFIED.,.F.,.F.,(4,2,2,2,2,2,1,4),(0.,0.000106412085437288,0.000212824170874576,
0.00042564834174915,0.000532060427186437,0.00058526646990508,0.000638472512623723,
0.000851296683498299),.UNSPECIFIED.);
#866=B_SPLINE_CURVE_WITH_KNOTS('',3,(#42869,#42870,#42871,#42872,#42873,
#42874,#42875,#42876,#42877,#42878,#42879,#42880,#42881,#42882,#42883,#42884,
#42885,#42886,#42887,#42888,#42889,#42890,#42891,#42892,#42893,#42894,#42895,
#42896,#42897,#42898,#42899,#42900,#42901,#42902,#42903,#42904,#42905,#42906,
#42907,#42908,#42909,#42910,#42911,#42912,#42913,#42914,#42915,#42916,#42917,
#42918,#42919,#42920,#42921,#42922,#42923,#42924,#42925,#42926,#42927,#42928,
#42929,#42930,#42931,#42932,#42933,#42934,#42935,#42936,#42937,#42938,#42939,
#42940,#42941,#42942,#42943,#42944,#42945,#42946,#42947,#42948,#42949,#42950,
#42951,#42952,#42953,#42954,#42955,#42956,#42957,#42958,#42959,#42960,#42961,
#42962,#42963,#42964,#42965,#42966,#42967,#42968),.UNSPECIFIED.,.F.,.F.,
(4,3,3,3,3,3,3,3,3,3,3,3,3,3,3,3,3,3,3,3,3,3,3,3,3,3,3,3,3,3,3,3,3,4),(-0.00256394233172042,
-0.00254391153225385,-0.00252388073278728,-0.00248381913385415,-0.00240369593598789,
-0.00224344954025536,-0.00192295674879031,-0.00190873837330291,-0.00160246395732526,
-0.00158284541228051,-0.00144221756159274,-0.00141973271419307,-0.00137890325788483,
-0.00136209436372648,-0.00133806214634055,-0.00128197116586021,-0.00125658871715488,
-0.000961478374395163,-0.000933814475721374,-0.000801231978662637,-0.000774027171965909,
-0.000640985582930111,-0.000615098742888476,-0.000575479456072158,-0.000560862385063846,
-0.000535906116609504,-0.000520800786130713,-0.000480739187197579,-0.000457228296741512,
-0.000320492791465053,-0.000302025544602755,-0.000160246395732526,-0.000149632584598168,
0.),.UNSPECIFIED.);
#867=B_SPLINE_CURVE_WITH_KNOTS('',3,(#42973,#42974,#42975,#42976,#42977,
#42978,#42979,#42980,#42981,#42982,#42983,#42984,#42985,#42986),
 .UNSPECIFIED.,.F.,.F.,(4,2,2,2,2,2,4),(-0.0927452748896928,-0.0905007143233686,
-0.0728860150149103,-0.0515184272327515,-0.024779386716326,0.,0.000385328304981227),
 .UNSPECIFIED.);
#868=B_SPLINE_CURVE_WITH_KNOTS('',3,(#43123,#43124,#43125,#43126,#43127,
#43128,#43129,#43130,#43131,#43132),.UNSPECIFIED.,.F.,.F.,(4,2,2,2,4),(0.148156232466478,
0.185223245600188,0.222275576316647,0.259307076631218,0.296319939605705),
 .UNSPECIFIED.);
#869=B_SPLINE_CURVE_WITH_KNOTS('',3,(#43148,#43149,#43150,#43151,#43152,
#43153,#43154,#43155,#43156,#43157,#43158,#43159,#43160,#43161,#43162,#43163,
#43164,#43165,#43166,#43167,#43168,#43169,#43170,#43171,#43172,#43173,#43174,
#43175),.UNSPECIFIED.,.F.,.F.,(4,2,2,1,1,1,1,2,2,2,1,2,2,1,2,1,1,4),(-0.000564130987588538,
-0.000559723714247997,-0.000558621895912863,-0.000557520077577729,-0.000555316440907461,
-0.000546501894226388,-0.000528872800864246,-0.000511243707502104,-0.000493614614139961,
-0.000423098240691392,-0.000352581867242823,-0.000282065493794254,-0.000264436400432113,
-0.000246807307069971,-0.000211549120345689,-0.000141032746897126,-7.0516373448563E-5,
0.),.UNSPECIFIED.);
#870=B_SPLINE_CURVE_WITH_KNOTS('',3,(#43215,#43216,#43217,#43218,#43219,
#43220),.UNSPECIFIED.,.F.,.F.,(4,2,4),(-0.296319939605705,-0.259307076631217,
-0.246794048708148),.UNSPECIFIED.);
#871=B_SPLINE_CURVE_WITH_KNOTS('',3,(#43286,#43287,#43288,#43289,#43290,
#43291,#43292,#43293,#43294,#43295),.UNSPECIFIED.,.F.,.F.,(4,2,2,2,4),(1.85749660968514E-7,
0.0288862347368519,0.0436805225665364,0.0576117094512964,0.0578367161617181),
 .UNSPECIFIED.);
#872=B_SPLINE_CURVE_WITH_KNOTS('',3,(#43352,#43353,#43354,#43355,#43356,
#43357,#43358,#43359,#43360,#43361),.UNSPECIFIED.,.F.,.F.,(4,2,2,2,4),(-0.000222102919063948,
5.84805343767944E-7,0.0138000274043402,0.0285383241859604,0.0573925375846453),
 .UNSPECIFIED.);
#873=B_SPLINE_CURVE_WITH_KNOTS('',3,(#43365,#43366,#43367,#43368,#43369,
#43370,#43371,#43372,#43373,#43374,#43375,#43376,#43377,#43378),
 .UNSPECIFIED.,.F.,.F.,(4,2,2,2,2,2,4),(0.0946327170802488,0.104761312570622,
0.122042430928541,0.143220348291086,0.167141047893638,0.19192929334763,
0.192359096840082),.UNSPECIFIED.);
#874=B_SPLINE_CURVE_WITH_KNOTS('',3,(#43381,#43382,#43383,#43384,#43385,
#43386,#43387,#43388,#43389,#43390,#43391,#43392,#43393,#43394),
 .UNSPECIFIED.,.F.,.F.,(4,2,2,2,2,2,4),(-0.000411443668019523,0.,0.0275273122201118,
0.0519146118706548,0.0703314286321732,0.0856354757935221,0.0916008603165112),
 .UNSPECIFIED.);
#875=B_SPLINE_CURVE_WITH_KNOTS('',3,(#43404,#43405,#43406,#43407,#43408,
#43409,#43410,#43411,#43412,#43413,#43414,#43415,#43416,#43417,#43418,#43419,
#43420,#43421,#43422,#43423,#43424,#43425,#43426,#43427,#43428,#43429,#43430,
#43431,#43432,#43433,#43434,#43435,#43436,#43437,#43438,#43439,#43440,#43441,
#43442,#43443,#43444,#43445,#43446,#43447,#43448,#43449,#43450,#43451,#43452,
#43453,#43454,#43455,#43456,#43457,#43458,#43459,#43460,#43461,#43462,#43463,
#43464,#43465,#43466,#43467,#43468,#43469,#43470,#43471,#43472,#43473,#43474,
#43475,#43476,#43477,#43478,#43479,#43480,#43481,#43482,#43483,#43484,#43485,
#43486,#43487,#43488,#43489,#43490,#43491,#43492,#43493,#43494,#43495,#43496,
#43497,#43498,#43499,#43500,#43501,#43502,#43503,#43504,#43505,#43506,#43507,
#43508,#43509,#43510,#43511,#43512,#43513,#43514,#43515,#43516,#43517,#43518,
#43519,#43520,#43521,#43522,#43523,#43524,#43525,#43526,#43527,#43528,#43529,
#43530,#43531,#43532,#43533,#43534,#43535,#43536,#43537,#43538,#43539,#43540,
#43541,#43542,#43543,#43544,#43545,#43546,#43547,#43548),.UNSPECIFIED.,
 .F.,.F.,(4,3,3,3,3,3,3,3,3,3,3,3,3,3,3,3,3,3,3,3,3,3,3,3,3,3,3,3,3,3,3,
3,3,3,3,3,3,3,3,3,3,3,3,3,3,3,3,3,4),(0.,7.25281274128516E-5,0.000100260712346105,
0.000145056254825703,0.000202140779546393,0.000290112509651402,0.000305551005043421,
0.000326376573357828,0.000331630115588394,0.000357792042008772,0.000362640637064254,
0.000410099908754193,0.000435168764477103,0.000507696891889952,0.000514262478642334,
0.000580225019302801,0.000617529589805025,0.00065275314671565,0.00066867663759029,
0.000689017210422073,0.000694078722306658,0.000719282121091699,0.000725281274128496,
0.000797809401541343,0.000817729131006324,0.00087033752895419,0.000906601592660614,
0.000911548617891743,0.000924733624513829,0.000934113589543727,0.000942865656367043,
0.000956289830416614,0.000979129720073469,0.000999397033360985,0.00101539378377989,
0.00104069347247581,0.00105165784748632,0.00106059531852788,0.00106072386341293,
0.00106978987933953,0.00107035367576909,0.00108001823510808,0.00108792191119275,
0.00111511995897257,0.0011295215242621,0.00113889549736231,0.00114231800675239,
0.00115419999406486,0.0011604500386056),.UNSPECIFIED.);
#876=B_SPLINE_CURVE_WITH_KNOTS('',3,(#43733,#43734,#43735,#43736,#43737,
#43738,#43739,#43740,#43741,#43742),.UNSPECIFIED.,.F.,.F.,(4,2,2,2,4),(-0.112036818610838,
-0.0880588875106408,-0.0481932450937528,0.,0.000430202592559268),
 .UNSPECIFIED.);
#877=B_SPLINE_CURVE_WITH_KNOTS('',3,(#43770,#43771,#43772,#43773,#43774,
#43775,#43776,#43777,#43778,#43779),.UNSPECIFIED.,.F.,.F.,(4,2,2,2,4),(0.299155723157873,
0.33592702742144,0.373117039271119,0.410786177696965,0.448805976438876),
 .UNSPECIFIED.);
#878=B_SPLINE_CURVE_WITH_KNOTS('',3,(#43824,#43825,#43826,#43827,#43828,
#43829,#43830,#43831,#43832,#43833),.UNSPECIFIED.,.F.,.F.,(4,2,2,2,4),(-0.150773602000823,
-0.131921867952132,-0.113070133903442,-0.0942115691388773,-0.0753530043743127),
 .UNSPECIFIED.);
#879=B_SPLINE_CURVE_WITH_KNOTS('',3,(#43834,#43835,#43836,#43837,#43838,
#43839,#43840,#43841,#43842,#43843),.UNSPECIFIED.,.F.,.F.,(4,2,2,2,4),(-0.226162872426322,
-0.207310338477511,-0.1884578045287,-0.169609037891303,-0.150760271253907),
 .UNSPECIFIED.);
#880=B_SPLINE_CURVE_WITH_KNOTS('',3,(#43846,#43847,#43848,#43849,#43850,
#43851,#43852,#43853,#43854,#43855,#43856,#43857),.UNSPECIFIED.,.F.,.F.,
(4,2,2,2,2,4),(-0.185807739244323,-0.185439968351168,-0.153680951419909,
-0.128893958592289,-0.110891637254666,-0.0965169641148303),
 .UNSPECIFIED.);
#881=B_SPLINE_CURVE_WITH_KNOTS('',3,(#43858,#43859,#43860,#43861,#43862,
#43863,#43864,#43865,#43866,#43867,#43868,#43869,#43870,#43871,#43872,#43873),
 .UNSPECIFIED.,.F.,.F.,(4,2,2,2,2,2,2,4),(-0.000448819179353507,2.36681334253586E-15,
0.0230636769571239,0.0450898293250805,0.0666977239398038,0.0825811068581514,
0.096351648403139,0.0963708477819653),.UNSPECIFIED.);
#882=B_SPLINE_CURVE_WITH_KNOTS('',3,(#43876,#43877,#43878,#43879,#43880,
#43881,#43882,#43883,#43884,#43885,#43886,#43887,#43888,#43889),
 .UNSPECIFIED.,.F.,.F.,(4,2,2,2,2,2,4),(0.0936926976814215,0.108568843397411,
0.125272597642247,0.146759187794151,0.166551065492561,0.187385395362841,
0.187824844805022),.UNSPECIFIED.);
#883=B_SPLINE_CURVE_WITH_KNOTS('',3,(#43892,#43893,#43894,#43895,#43896,
#43897,#43898,#43899,#43900,#43901,#43902,#43903,#43904,#43905),
 .UNSPECIFIED.,.F.,.F.,(4,2,2,2,2,2,4),(-0.0939314403057516,-0.079108380427945,
-0.0624459947612743,-0.0409578088889437,-0.021014451885627,0.,0.000441387027955698),
 .UNSPECIFIED.);
#884=B_SPLINE_CURVE_WITH_KNOTS('',3,(#43907,#43908,#43909,#43910,#43911,
#43912),.UNSPECIFIED.,.F.,.F.,(4,2,4),(-0.0864860550818585,-0.0617458959675404,
0.),.UNSPECIFIED.);
#885=B_SPLINE_CURVE_WITH_KNOTS('',3,(#43919,#43920,#43921,#43922,#43923,
#43924,#43925,#43926),.UNSPECIFIED.,.F.,.F.,(4,2,2,4),(0.,0.0332644074051895,
0.0665288148103791,0.0864490647425511),.UNSPECIFIED.);
#886=B_SPLINE_CURVE_WITH_KNOTS('',3,(#43927,#43928,#43929,#43930,#43931,
#43932,#43933,#43934),.UNSPECIFIED.,.F.,.F.,(4,2,2,4),(0.292643145412176,
0.312563395344359,0.345827802749548,0.379092210154738),.UNSPECIFIED.);
#887=B_SPLINE_CURVE_WITH_KNOTS('',3,(#43939,#43940,#43941,#43942,#43943,
#43944,#43945,#43946,#43947,#43948,#43949,#43950,#43951,#43952,#43953,#43954,
#43955,#43956,#43957,#43958,#43959,#43960,#43961,#43962,#43963,#43964,#43965,
#43966,#43967,#43968,#43969,#43970,#43971,#43972,#43973,#43974),
 .UNSPECIFIED.,.F.,.F.,(4,1,2,2,1,1,2,2,2,1,1,1,2,2,1,1,1,2,2,2,1,1,1,4),
(8.26379378955844E-9,9.84772534748752E-5,0.00019695450694975,0.000246193133687188,
0.000295431760424625,0.0003939090138995,0.000492386267374374,0.000541624894111811,
0.000566244207480527,0.000590863520849243,0.000689340774324121,0.000787818027798999,
0.000886295281273877,0.000910914594642603,0.00093553390801133,0.000984772534748781,
0.00108324978822369,0.0011817270416986,0.00123096566843606,0.00125558498180478,
0.00128020429517351,0.00137868154864839,0.00147715880212328,0.00157563605559816),
 .UNSPECIFIED.);
#888=B_SPLINE_CURVE_WITH_KNOTS('',3,(#44219,#44220,#44221,#44222,#44223,
#44224,#44225,#44226,#44227,#44228,#44229,#44230,#44231,#44232),
 .UNSPECIFIED.,.F.,.F.,(4,2,2,2,2,2,4),(0.0980600308863261,0.111872145553039,
0.127734088362621,0.149209172354546,0.171902467951158,0.196120061772115,
0.196592003096005),.UNSPECIFIED.);
#889=B_SPLINE_CURVE_WITH_KNOTS('',3,(#44233,#44234,#44235,#44236,#44237,
#44238,#44239,#44240,#44241,#44242,#44243,#44244,#44245,#44246),
 .UNSPECIFIED.,.F.,.F.,(4,2,2,2,2,2,4),(-0.0919962992060375,-0.0866822297910484,
-0.0715424159762288,-0.0533700787866219,-0.0291975579830104,0.,0.000414145167341223),
 .UNSPECIFIED.);
#890=B_SPLINE_CURVE_WITH_KNOTS('',3,(#44248,#44249,#44250,#44251,#44252,
#44253,#44254,#44255,#44256,#44257,#44258,#44259,#44260,#44261),
 .UNSPECIFIED.,.F.,.F.,(4,2,2,2,2,2,4),(-0.000473267087033522,0.,0.024346315423422,
0.0471447393419604,0.0686144817737718,0.0844484317067967,0.0982274249930373),
 .UNSPECIFIED.);
#891=B_SPLINE_CURVE_WITH_KNOTS('',3,(#44262,#44263,#44264,#44265,#44266,
#44267,#44268,#44269,#44270,#44271,#44272,#44273,#44274,#44275),
 .UNSPECIFIED.,.F.,.F.,(4,2,2,2,2,2,4),(-0.211473737795484,-0.210980472033705,
-0.177081462686025,-0.148068102900271,-0.126207979465772,-0.108019352485251,
-0.101286341673499),.UNSPECIFIED.);
#892=B_SPLINE_CURVE_WITH_KNOTS('',3,(#44363,#44364,#44365,#44366,#44367,
#44368,#44369,#44370,#44371,#44372,#44373,#44374,#44375,#44376),
 .UNSPECIFIED.,.F.,.F.,(4,2,2,2,2,2,4),(-0.19692811707828,-0.196454849991217,
-0.172108534567229,-0.149310110648075,-0.127840368215671,-0.112006418282226,
-0.0982274249956043),.UNSPECIFIED.);
#893=B_SPLINE_CURVE_WITH_KNOTS('',3,(#44377,#44378,#44379,#44380,#44381,
#44382,#44383,#44384,#44385,#44386,#44387,#44388,#44389,#44390),
 .UNSPECIFIED.,.F.,.F.,(4,2,2,2,2,2,4),(-0.0983962336263429,-0.0846504542685971,
-0.0688446450995894,-0.0473804831279508,-0.0244761756223594,0.,0.000474604118846155),
 .UNSPECIFIED.);
#894=B_SPLINE_CURVE_WITH_KNOTS('',3,(#44394,#44395,#44396,#44397,#44398,
#44399,#44400,#44401,#44402,#44403,#44404,#44405,#44406,#44407),
 .UNSPECIFIED.,.F.,.F.,(4,2,2,2,2,2,4),(-0.21147373779364,-0.210980472031872,
-0.177081462684556,-0.148068102899106,-0.126207979464849,-0.108019352484536,
-0.101286341672861),.UNSPECIFIED.);
#895=B_SPLINE_CURVE_WITH_KNOTS('',3,(#44409,#44410,#44411,#44412,#44413,
#44414,#44415,#44416,#44417,#44418,#44419,#44420),.UNSPECIFIED.,.F.,.F.,
(4,2,2,2,2,4),(0.319067164078173,0.339664273857546,0.372500022353856,0.411302550267559,
0.451625546677781,0.452232637057266),.UNSPECIFIED.);
#1041=CONICAL_SURFACE('',#15890,4.,0.785398163397448);
#1636=LINE('',#35550,#2829);
#1637=LINE('',#35558,#2830);
#1638=LINE('',#35565,#2831);
#1639=LINE('',#35571,#2832);
#1640=LINE('',#35575,#2833);
#1641=LINE('',#35592,#2834);
#1642=LINE('',#35609,#2835);
#1643=LINE('',#35613,#2836);
#1644=LINE('',#35620,#2837);
#1645=LINE('',#35624,#2838);
#1646=LINE('',#35645,#2839);
#1647=LINE('',#35717,#2840);
#1648=LINE('',#35728,#2841);
#1649=LINE('',#35841,#2842);
#1650=LINE('',#35844,#2843);
#1651=LINE('',#36060,#2844);
#1652=LINE('',#36075,#2845);
#1653=LINE('',#36079,#2846);
#1654=LINE('',#36151,#2847);
#1655=LINE('',#36159,#2848);
#1656=LINE('',#36347,#2849);
#1657=LINE('',#36349,#2850);
#1658=LINE('',#36352,#2851);
#1659=LINE('',#36355,#2852);
#1660=LINE('',#36360,#2853);
#1661=LINE('',#36366,#2854);
#1662=LINE('',#36584,#2855);
#1663=LINE('',#36599,#2856);
#1664=LINE('',#36603,#2857);
#1665=LINE('',#36607,#2858);
#1666=LINE('',#36611,#2859);
#1667=LINE('',#36631,#2860);
#1668=LINE('',#36634,#2861);
#1669=LINE('',#36678,#2862);
#1670=LINE('',#39178,#2863);
#1671=LINE('',#39180,#2864);
#1672=LINE('',#41332,#2865);
#1673=LINE('',#41333,#2866);
#1674=LINE('',#41336,#2867);
#1675=LINE('',#41338,#2868);
#1676=LINE('',#41339,#2869);
#1677=LINE('',#41341,#2870);
#1678=LINE('',#41342,#2871);
#1679=LINE('',#41343,#2872);
#1680=LINE('',#41345,#2873);
#1681=LINE('',#41346,#2874);
#1682=LINE('',#41347,#2875);
#1683=LINE('',#41351,#2876);
#1684=LINE('',#41353,#2877);
#1685=LINE('',#41355,#2878);
#1686=LINE('',#41356,#2879);
#1687=LINE('',#41360,#2880);
#1688=LINE('',#41362,#2881);
#1689=LINE('',#41364,#2882);
#1690=LINE('',#41365,#2883);
#1691=LINE('',#41369,#2884);
#1692=LINE('',#41371,#2885);
#1693=LINE('',#41373,#2886);
#1694=LINE('',#41374,#2887);
#1695=LINE('',#41376,#2888);
#1696=LINE('',#41378,#2889);
#1697=LINE('',#41380,#2890);
#1698=LINE('',#41416,#2891);
#1699=LINE('',#41447,#2892);
#1700=LINE('',#41449,#2893);
#1701=LINE('',#41451,#2894);
#1702=LINE('',#41496,#2895);
#1703=LINE('',#41497,#2896);
#1704=LINE('',#41503,#2897);
#1705=LINE('',#41505,#2898);
#1706=LINE('',#41506,#2899);
#1707=LINE('',#41652,#2900);
#1708=LINE('',#41655,#2901);
#1709=LINE('',#41957,#2902);
#1710=LINE('',#41958,#2903);
#1711=LINE('',#41961,#2904);
#1712=LINE('',#41962,#2905);
#1713=LINE('',#41964,#2906);
#1714=LINE('',#41965,#2907);
#1715=LINE('',#41966,#2908);
#1716=LINE('',#41968,#2909);
#1717=LINE('',#42001,#2910);
#1718=LINE('',#42003,#2911);
#1719=LINE('',#42005,#2912);
#1720=LINE('',#42007,#2913);
#1721=LINE('',#42010,#2914);
#1722=LINE('',#42011,#2915);
#1723=LINE('',#42033,#2916);
#1724=LINE('',#42410,#2917);
#1725=LINE('',#42414,#2918);
#1726=LINE('',#42563,#2919);
#1727=LINE('',#43117,#2920);
#1728=LINE('',#43136,#2921);
#1729=LINE('',#43140,#2922);
#1730=LINE('',#43145,#2923);
#1731=LINE('',#43147,#2924);
#1732=LINE('',#43176,#2925);
#1733=LINE('',#43187,#2926);
#1734=LINE('',#43192,#2927);
#1735=LINE('',#43196,#2928);
#1736=LINE('',#43197,#2929);
#1737=LINE('',#43199,#2930);
#1738=LINE('',#43203,#2931);
#1739=LINE('',#43204,#2932);
#1740=LINE('',#43206,#2933);
#1741=LINE('',#43207,#2934);
#1742=LINE('',#43211,#2935);
#1743=LINE('',#43213,#2936);
#1744=LINE('',#43221,#2937);
#1745=LINE('',#43223,#2938);
#1746=LINE('',#43225,#2939);
#1747=LINE('',#43226,#2940);
#1748=LINE('',#43230,#2941);
#1749=LINE('',#43380,#2942);
#1750=LINE('',#43549,#2943);
#1751=LINE('',#43750,#2944);
#1752=LINE('',#43753,#2945);
#1753=LINE('',#43756,#2946);
#1754=LINE('',#43759,#2947);
#1755=LINE('',#43763,#2948);
#1756=LINE('',#43769,#2949);
#1757=LINE('',#43787,#2950);
#1758=LINE('',#43790,#2951);
#1759=LINE('',#43794,#2952);
#1760=LINE('',#43799,#2953);
#1761=LINE('',#43803,#2954);
#1762=LINE('',#43807,#2955);
#1763=LINE('',#43810,#2956);
#1764=LINE('',#43812,#2957);
#1765=LINE('',#43814,#2958);
#1766=LINE('',#43815,#2959);
#1767=LINE('',#43914,#2960);
#1768=LINE('',#43936,#2961);
#1769=LINE('',#43977,#2962);
#1770=LINE('',#43979,#2963);
#1771=LINE('',#44215,#2964);
#1772=LINE('',#44216,#2965);
#1773=LINE('',#44427,#2966);
#1774=LINE('',#44428,#2967);
#1775=LINE('',#44430,#2968);
#2829=VECTOR('',#18639,4.);
#2830=VECTOR('',#18648,4.);
#2831=VECTOR('',#18657,4.);
#2832=VECTOR('',#18662,2.8);
#2833=VECTOR('',#18665,1000.);
#2834=VECTOR('',#18668,1000.);
#2835=VECTOR('',#18671,1000.);
#2836=VECTOR('',#18674,1000.);
#2837=VECTOR('',#18683,2.5);
#2838=VECTOR('',#18686,1000.);
#2839=VECTOR('',#18687,1000.);
#2840=VECTOR('',#18690,1000.);
#2841=VECTOR('',#18693,1000.);
#2842=VECTOR('',#18718,1000.);
#2843=VECTOR('',#18721,1000.);
#2844=VECTOR('',#18730,1000.);
#2845=VECTOR('',#18733,1000.);
#2846=VECTOR('',#18736,1000.);
#2847=VECTOR('',#18767,1.5);
#2848=VECTOR('',#18776,1000.);
#2849=VECTOR('',#18779,1000.);
#2850=VECTOR('',#18780,1000.);
#2851=VECTOR('',#18783,1000.);
#2852=VECTOR('',#18786,1000.);
#2853=VECTOR('',#18791,1000.);
#2854=VECTOR('',#18798,1000.);
#2855=VECTOR('',#18815,1000.);
#2856=VECTOR('',#18818,1000.);
#2857=VECTOR('',#18821,1000.);
#2858=VECTOR('',#18824,1000.);
#2859=VECTOR('',#18827,1000.);
#2860=VECTOR('',#18828,1000.);
#2861=VECTOR('',#18831,1000.);
#2862=VECTOR('',#18836,1000.);
#2863=VECTOR('',#18865,0.8);
#2864=VECTOR('',#18868,0.8);
#2865=VECTOR('',#18875,1000.);
#2866=VECTOR('',#18876,1000.);
#2867=VECTOR('',#18879,1000.);
#2868=VECTOR('',#18880,1000.);
#2869=VECTOR('',#18881,1000.);
#2870=VECTOR('',#18884,1000.);
#2871=VECTOR('',#18885,1000.);
#2872=VECTOR('',#18886,1000.);
#2873=VECTOR('',#18889,1000.);
#2874=VECTOR('',#18890,1000.);
#2875=VECTOR('',#18891,1000.);
#2876=VECTOR('',#18894,1000.);
#2877=VECTOR('',#18895,1000.);
#2878=VECTOR('',#18896,1000.);
#2879=VECTOR('',#18897,1000.);
#2880=VECTOR('',#18900,1000.);
#2881=VECTOR('',#18901,1000.);
#2882=VECTOR('',#18902,1000.);
#2883=VECTOR('',#18903,1000.);
#2884=VECTOR('',#18906,1000.);
#2885=VECTOR('',#18907,1000.);
#2886=VECTOR('',#18908,1000.);
#2887=VECTOR('',#18909,1000.);
#2888=VECTOR('',#18912,1000.);
#2889=VECTOR('',#18915,1000.);
#2890=VECTOR('',#18918,1000.);
#2891=VECTOR('',#18927,1000.);
#2892=VECTOR('',#18930,1000.);
#2893=VECTOR('',#18933,1000.);
#2894=VECTOR('',#18936,1000.);
#2895=VECTOR('',#18955,1000.);
#2896=VECTOR('',#18956,1000.);
#2897=VECTOR('',#18961,1000.);
#2898=VECTOR('',#18962,1000.);
#2899=VECTOR('',#18963,1000.);
#2900=VECTOR('',#18972,1000.);
#2901=VECTOR('',#18975,1000.);
#2902=VECTOR('',#18980,1000.);
#2903=VECTOR('',#18981,1000.);
#2904=VECTOR('',#18984,1000.);
#2905=VECTOR('',#18985,1000.);
#2906=VECTOR('',#18986,1000.);
#2907=VECTOR('',#18987,1000.);
#2908=VECTOR('',#18988,1000.);
#2909=VECTOR('',#18991,1000.);
#2910=VECTOR('',#19000,1000.);
#2911=VECTOR('',#19003,1000.);
#2912=VECTOR('',#19006,1000.);
#2913=VECTOR('',#19009,1000.);
#2914=VECTOR('',#19012,1000.);
#2915=VECTOR('',#19013,1000.);
#2916=VECTOR('',#19022,1000.);
#2917=VECTOR('',#19031,1000.);
#2918=VECTOR('',#19036,1000.);
#2919=VECTOR('',#19041,1000.);
#2920=VECTOR('',#19068,1000.);
#2921=VECTOR('',#19079,1000.);
#2922=VECTOR('',#19082,1000.);
#2923=VECTOR('',#19087,1000.);
#2924=VECTOR('',#19088,1000.);
#2925=VECTOR('',#19089,1000.);
#2926=VECTOR('',#19104,1000.);
#2927=VECTOR('',#19111,1000.);
#2928=VECTOR('',#19116,1000.);
#2929=VECTOR('',#19117,1000.);
#2930=VECTOR('',#19120,1000.);
#2931=VECTOR('',#19123,1000.);
#2932=VECTOR('',#19124,1000.);
#2933=VECTOR('',#19125,1000.);
#2934=VECTOR('',#19126,1000.);
#2935=VECTOR('',#19129,1000.);
#2936=VECTOR('',#19130,1000.);
#2937=VECTOR('',#19131,1000.);
#2938=VECTOR('',#19132,1000.);
#2939=VECTOR('',#19133,1000.);
#2940=VECTOR('',#19134,1000.);
#2941=VECTOR('',#19139,1000.);
#2942=VECTOR('',#19146,1000.);
#2943=VECTOR('',#19161,1000.);
#2944=VECTOR('',#19180,1000.);
#2945=VECTOR('',#19183,1000.);
#2946=VECTOR('',#19186,1000.);
#2947=VECTOR('',#19187,1000.);
#2948=VECTOR('',#19190,1000.);
#2949=VECTOR('',#19201,1000.);
#2950=VECTOR('',#19212,1000.);
#2951=VECTOR('',#19217,1000.);
#2952=VECTOR('',#19220,1000.);
#2953=VECTOR('',#19225,1000.);
#2954=VECTOR('',#19228,1000.);
#2955=VECTOR('',#19233,1000.);
#2956=VECTOR('',#19236,1000.);
#2957=VECTOR('',#19239,1000.);
#2958=VECTOR('',#19240,1000.);
#2959=VECTOR('',#19241,1000.);
#2960=VECTOR('',#19274,1000.);
#2961=VECTOR('',#19283,1000.);
#2962=VECTOR('',#19290,1000.);
#2963=VECTOR('',#19291,1000.);
#2964=VECTOR('',#19306,1000.);
#2965=VECTOR('',#19307,1000.);
#2966=VECTOR('',#19338,1000.);
#2967=VECTOR('',#19339,1000.);
#2968=VECTOR('',#19342,1000.);
#3486=CYLINDRICAL_SURFACE('',#15887,4.);
#3487=CYLINDRICAL_SURFACE('',#15894,4.);
#3488=CYLINDRICAL_SURFACE('',#15897,2.8);
#3489=CYLINDRICAL_SURFACE('',#15905,2.5);
#3490=CYLINDRICAL_SURFACE('',#15920,17.);
#3491=CYLINDRICAL_SURFACE('',#15923,17.);
#3492=CYLINDRICAL_SURFACE('',#15942,1.5);
#3493=CYLINDRICAL_SURFACE('',#15945,3.8);
#3494=CYLINDRICAL_SURFACE('',#15950,0.499999999999999);
#3495=CYLINDRICAL_SURFACE('',#15953,1.);
#3496=CYLINDRICAL_SURFACE('',#15961,2.5);
#3497=CYLINDRICAL_SURFACE('',#15968,0.500000000000002);
#3498=CYLINDRICAL_SURFACE('',#15984,0.8);
#3499=CYLINDRICAL_SURFACE('',#15985,0.8);
#3500=CYLINDRICAL_SURFACE('',#15988,6.);
#3501=CYLINDRICAL_SURFACE('',#15996,0.5);
#3502=CYLINDRICAL_SURFACE('',#15997,0.5);
#3503=CYLINDRICAL_SURFACE('',#16001,0.5);
#3504=CYLINDRICAL_SURFACE('',#16002,0.5);
#3505=CYLINDRICAL_SURFACE('',#16003,0.5);
#3506=CYLINDRICAL_SURFACE('',#16004,0.5);
#3507=CYLINDRICAL_SURFACE('',#16013,0.5);
#3508=CYLINDRICAL_SURFACE('',#16019,0.5);
#3509=CYLINDRICAL_SURFACE('',#16036,0.5);
#3510=CYLINDRICAL_SURFACE('',#16040,0.500000000000002);
#3511=CYLINDRICAL_SURFACE('',#16041,0.5);
#3512=CYLINDRICAL_SURFACE('',#16044,0.5);
#3513=CYLINDRICAL_SURFACE('',#16057,0.5);
#3514=CYLINDRICAL_SURFACE('',#16062,10.5);
#3515=CYLINDRICAL_SURFACE('',#16069,1.);
#3516=CYLINDRICAL_SURFACE('',#16072,1.);
#3517=CYLINDRICAL_SURFACE('',#16075,1.);
#3518=CYLINDRICAL_SURFACE('',#16081,0.5);
#3519=CYLINDRICAL_SURFACE('',#16085,0.499999999999999);
#3520=CYLINDRICAL_SURFACE('',#16092,0.5);
#3521=CYLINDRICAL_SURFACE('',#16093,3.8);
#3522=CYLINDRICAL_SURFACE('',#16111,10.5);
#3523=CYLINDRICAL_SURFACE('',#16113,10.5);
#3524=CYLINDRICAL_SURFACE('',#16125,6.);
#3525=CYLINDRICAL_SURFACE('',#16128,10.5);
#3526=CYLINDRICAL_SURFACE('',#16129,6.);
#3527=CYLINDRICAL_SURFACE('',#16132,6.);
#3528=CYLINDRICAL_SURFACE('',#16135,0.5);
#3529=CYLINDRICAL_SURFACE('',#16136,0.5);
#3530=CYLINDRICAL_SURFACE('',#16137,0.5);
#3531=CYLINDRICAL_SURFACE('',#16139,0.5);
#3532=CYLINDRICAL_SURFACE('',#16141,1.);
#3533=CYLINDRICAL_SURFACE('',#16143,1.);
#3534=CYLINDRICAL_SURFACE('',#16144,0.5);
#3535=CYLINDRICAL_SURFACE('',#16149,0.5);
#3536=CYLINDRICAL_SURFACE('',#16152,0.5);
#3537=CYLINDRICAL_SURFACE('',#16153,4.5);
#3538=CYLINDRICAL_SURFACE('',#16156,0.5);
#3539=CYLINDRICAL_SURFACE('',#16157,0.5);
#3540=CYLINDRICAL_SURFACE('',#16161,0.5);
#3541=CYLINDRICAL_SURFACE('',#16162,0.5);
#3542=CYLINDRICAL_SURFACE('',#16164,0.5);
#3543=CYLINDRICAL_SURFACE('',#16165,13.5);
#3544=CYLINDRICAL_SURFACE('',#16172,0.499999999999999);
#4004=FACE_OUTER_BOUND('',#4901,.T.);
#4005=FACE_OUTER_BOUND('',#4902,.T.);
#4006=FACE_OUTER_BOUND('',#4903,.T.);
#4007=FACE_OUTER_BOUND('',#4904,.T.);
#4008=FACE_OUTER_BOUND('',#4905,.T.);
#4009=FACE_OUTER_BOUND('',#4906,.T.);
#4010=FACE_OUTER_BOUND('',#4907,.T.);
#4011=FACE_OUTER_BOUND('',#4908,.T.);
#4012=FACE_OUTER_BOUND('',#4909,.T.);
#4013=FACE_OUTER_BOUND('',#4910,.T.);
#4014=FACE_OUTER_BOUND('',#4911,.T.);
#4015=FACE_OUTER_BOUND('',#4913,.T.);
#4016=FACE_OUTER_BOUND('',#4914,.T.);
#4017=FACE_OUTER_BOUND('',#4915,.T.);
#4018=FACE_OUTER_BOUND('',#4916,.T.);
#4019=FACE_OUTER_BOUND('',#4917,.T.);
#4020=FACE_OUTER_BOUND('',#4918,.T.);
#4021=FACE_OUTER_BOUND('',#4919,.T.);
#4022=FACE_OUTER_BOUND('',#4920,.T.);
#4023=FACE_OUTER_BOUND('',#4921,.T.);
#4024=FACE_OUTER_BOUND('',#4922,.T.);
#4025=FACE_OUTER_BOUND('',#4923,.T.);
#4026=FACE_OUTER_BOUND('',#4924,.T.);
#4027=FACE_OUTER_BOUND('',#4925,.T.);
#4028=FACE_OUTER_BOUND('',#4926,.T.);
#4029=FACE_OUTER_BOUND('',#4927,.T.);
#4030=FACE_OUTER_BOUND('',#4928,.T.);
#4031=FACE_OUTER_BOUND('',#4929,.T.);
#4032=FACE_OUTER_BOUND('',#4930,.T.);
#4033=FACE_OUTER_BOUND('',#4931,.T.);
#4034=FACE_OUTER_BOUND('',#4932,.T.);
#4035=FACE_OUTER_BOUND('',#4933,.T.);
#4036=FACE_OUTER_BOUND('',#4934,.T.);
#4037=FACE_OUTER_BOUND('',#4935,.T.);
#4038=FACE_OUTER_BOUND('',#4936,.T.);
#4039=FACE_OUTER_BOUND('',#4937,.T.);
#4040=FACE_OUTER_BOUND('',#4938,.T.);
#4041=FACE_OUTER_BOUND('',#4939,.T.);
#4042=FACE_OUTER_BOUND('',#4940,.T.);
#4043=FACE_OUTER_BOUND('',#4941,.T.);
#4044=FACE_OUTER_BOUND('',#4942,.T.);
#4045=FACE_OUTER_BOUND('',#4943,.T.);
#4046=FACE_OUTER_BOUND('',#4944,.T.);
#4047=FACE_OUTER_BOUND('',#4945,.T.);
#4048=FACE_OUTER_BOUND('',#4946,.T.);
#4049=FACE_OUTER_BOUND('',#4947,.T.);
#4050=FACE_OUTER_BOUND('',#4948,.T.);
#4051=FACE_OUTER_BOUND('',#4949,.T.);
#4052=FACE_OUTER_BOUND('',#4950,.T.);
#4053=FACE_OUTER_BOUND('',#4951,.T.);
#4054=FACE_OUTER_BOUND('',#4952,.T.);
#4055=FACE_OUTER_BOUND('',#4953,.T.);
#4056=FACE_OUTER_BOUND('',#4954,.T.);
#4057=FACE_OUTER_BOUND('',#4955,.T.);
#4058=FACE_OUTER_BOUND('',#4956,.T.);
#4059=FACE_OUTER_BOUND('',#4957,.T.);
#4060=FACE_OUTER_BOUND('',#4958,.T.);
#4061=FACE_OUTER_BOUND('',#4959,.T.);
#4062=FACE_OUTER_BOUND('',#4960,.T.);
#4063=FACE_OUTER_BOUND('',#4961,.T.);
#4064=FACE_OUTER_BOUND('',#4962,.T.);
#4065=FACE_OUTER_BOUND('',#4963,.T.);
#4066=FACE_OUTER_BOUND('',#4964,.T.);
#4067=FACE_OUTER_BOUND('',#4965,.T.);
#4068=FACE_OUTER_BOUND('',#4966,.T.);
#4069=FACE_OUTER_BOUND('',#4967,.T.);
#4070=FACE_OUTER_BOUND('',#4968,.T.);
#4071=FACE_OUTER_BOUND('',#4969,.T.);
#4072=FACE_OUTER_BOUND('',#4970,.T.);
#4073=FACE_OUTER_BOUND('',#4971,.T.);
#4074=FACE_OUTER_BOUND('',#4972,.T.);
#4075=FACE_OUTER_BOUND('',#4973,.T.);
#4076=FACE_OUTER_BOUND('',#4974,.T.);
#4077=FACE_OUTER_BOUND('',#4975,.T.);
#4078=FACE_OUTER_BOUND('',#4976,.T.);
#4079=FACE_OUTER_BOUND('',#4977,.T.);
#4080=FACE_OUTER_BOUND('',#4978,.T.);
#4081=FACE_OUTER_BOUND('',#4979,.T.);
#4082=FACE_OUTER_BOUND('',#4980,.T.);
#4083=FACE_OUTER_BOUND('',#4981,.T.);
#4084=FACE_OUTER_BOUND('',#4982,.T.);
#4085=FACE_OUTER_BOUND('',#4983,.T.);
#4086=FACE_OUTER_BOUND('',#4984,.T.);
#4087=FACE_OUTER_BOUND('',#4985,.T.);
#4088=FACE_OUTER_BOUND('',#4986,.T.);
#4089=FACE_OUTER_BOUND('',#4987,.T.);
#4090=FACE_OUTER_BOUND('',#4988,.T.);
#4091=FACE_OUTER_BOUND('',#4989,.T.);
#4092=FACE_OUTER_BOUND('',#4990,.T.);
#4093=FACE_OUTER_BOUND('',#4991,.T.);
#4094=FACE_OUTER_BOUND('',#4992,.T.);
#4095=FACE_OUTER_BOUND('',#4993,.T.);
#4096=FACE_OUTER_BOUND('',#4994,.T.);
#4097=FACE_OUTER_BOUND('',#4995,.T.);
#4098=FACE_OUTER_BOUND('',#4996,.T.);
#4099=FACE_OUTER_BOUND('',#4997,.T.);
#4100=FACE_OUTER_BOUND('',#4998,.T.);
#4101=FACE_OUTER_BOUND('',#4999,.T.);
#4102=FACE_OUTER_BOUND('',#5000,.T.);
#4103=FACE_OUTER_BOUND('',#5001,.T.);
#4104=FACE_OUTER_BOUND('',#5002,.T.);
#4105=FACE_OUTER_BOUND('',#5003,.T.);
#4106=FACE_OUTER_BOUND('',#5004,.T.);
#4107=FACE_OUTER_BOUND('',#5005,.T.);
#4108=FACE_OUTER_BOUND('',#5006,.T.);
#4109=FACE_OUTER_BOUND('',#5007,.T.);
#4110=FACE_OUTER_BOUND('',#5008,.T.);
#4111=FACE_OUTER_BOUND('',#5009,.T.);
#4112=FACE_OUTER_BOUND('',#5010,.T.);
#4113=FACE_OUTER_BOUND('',#5011,.T.);
#4114=FACE_OUTER_BOUND('',#5016,.T.);
#4115=FACE_OUTER_BOUND('',#5018,.T.);
#4116=FACE_OUTER_BOUND('',#5019,.T.);
#4117=FACE_OUTER_BOUND('',#5020,.T.);
#4118=FACE_OUTER_BOUND('',#5021,.T.);
#4119=FACE_OUTER_BOUND('',#5022,.T.);
#4120=FACE_OUTER_BOUND('',#5023,.T.);
#4121=FACE_OUTER_BOUND('',#5024,.T.);
#4122=FACE_OUTER_BOUND('',#5025,.T.);
#4123=FACE_OUTER_BOUND('',#5026,.T.);
#4124=FACE_OUTER_BOUND('',#5027,.T.);
#4125=FACE_OUTER_BOUND('',#5028,.T.);
#4126=FACE_OUTER_BOUND('',#5029,.T.);
#4127=FACE_OUTER_BOUND('',#5030,.T.);
#4128=FACE_OUTER_BOUND('',#5031,.T.);
#4129=FACE_OUTER_BOUND('',#5032,.T.);
#4130=FACE_OUTER_BOUND('',#5033,.T.);
#4131=FACE_OUTER_BOUND('',#5034,.T.);
#4132=FACE_OUTER_BOUND('',#5035,.T.);
#4133=FACE_OUTER_BOUND('',#5036,.T.);
#4134=FACE_OUTER_BOUND('',#5037,.T.);
#4135=FACE_OUTER_BOUND('',#5038,.T.);
#4136=FACE_OUTER_BOUND('',#5039,.T.);
#4137=FACE_OUTER_BOUND('',#5040,.T.);
#4138=FACE_OUTER_BOUND('',#5041,.T.);
#4139=FACE_OUTER_BOUND('',#5042,.T.);
#4140=FACE_OUTER_BOUND('',#5044,.T.);
#4141=FACE_OUTER_BOUND('',#5045,.T.);
#4142=FACE_OUTER_BOUND('',#5046,.T.);
#4143=FACE_OUTER_BOUND('',#5047,.T.);
#4144=FACE_OUTER_BOUND('',#5048,.T.);
#4145=FACE_OUTER_BOUND('',#5049,.T.);
#4146=FACE_OUTER_BOUND('',#5051,.T.);
#4147=FACE_OUTER_BOUND('',#5052,.T.);
#4148=FACE_OUTER_BOUND('',#5053,.T.);
#4149=FACE_OUTER_BOUND('',#5054,.T.);
#4150=FACE_OUTER_BOUND('',#5055,.T.);
#4151=FACE_OUTER_BOUND('',#5056,.T.);
#4152=FACE_OUTER_BOUND('',#5057,.T.);
#4153=FACE_OUTER_BOUND('',#5058,.T.);
#4154=FACE_OUTER_BOUND('',#5059,.T.);
#4155=FACE_OUTER_BOUND('',#5060,.T.);
#4156=FACE_OUTER_BOUND('',#5061,.T.);
#4157=FACE_OUTER_BOUND('',#5062,.T.);
#4158=FACE_OUTER_BOUND('',#5063,.T.);
#4159=FACE_OUTER_BOUND('',#5064,.T.);
#4160=FACE_OUTER_BOUND('',#5065,.T.);
#4161=FACE_OUTER_BOUND('',#5066,.T.);
#4162=FACE_OUTER_BOUND('',#5067,.T.);
#4163=FACE_OUTER_BOUND('',#5068,.T.);
#4164=FACE_OUTER_BOUND('',#5069,.T.);
#4165=FACE_OUTER_BOUND('',#5070,.T.);
#4166=FACE_OUTER_BOUND('',#5071,.T.);
#4901=EDGE_LOOP('',(#11411,#11412,#11413,#11414,#11415,#11416,#11417,#11418));
#4902=EDGE_LOOP('',(#11419,#11420,#11421,#11422,#11423,#11424,#11425,#11426));
#4903=EDGE_LOOP('',(#11427,#11428,#11429,#11430,#11431,#11432,#11433,#11434,
#11435));
#4904=EDGE_LOOP('',(#11436,#11437,#11438,#11439,#11440,#11441,#11442));
#4905=EDGE_LOOP('',(#11443,#11444,#11445,#11446,#11447));
#4906=EDGE_LOOP('',(#11448,#11449,#11450,#11451,#11452));
#4907=EDGE_LOOP('',(#11453,#11454,#11455,#11456));
#4908=EDGE_LOOP('',(#11457,#11458,#11459,#11460,#11461));
#4909=EDGE_LOOP('',(#11462,#11463,#11464,#11465,#11466,#11467));
#4910=EDGE_LOOP('',(#11468,#11469,#11470,#11471,#11472,#11473,#11474,#11475,
#11476,#11477,#11478,#11479,#11480,#11481,#11482));
#4911=EDGE_LOOP('',(#11483,#11484,#11485,#11486,#11487,#11488,#11489,#11490,
#11491,#11492,#11493,#11494,#11495,#11496,#11497));
#4912=EDGE_LOOP('',(#11498,#11499,#11500));
#4913=EDGE_LOOP('',(#11501,#11502,#11503,#11504,#11505));
#4914=EDGE_LOOP('',(#11506,#11507,#11508,#11509));
#4915=EDGE_LOOP('',(#11510,#11511,#11512,#11513));
#4916=EDGE_LOOP('',(#11514,#11515,#11516,#11517));
#4917=EDGE_LOOP('',(#11518,#11519,#11520,#11521,#11522,#11523,#11524,#11525,
#11526,#11527,#11528,#11529,#11530,#11531));
#4918=EDGE_LOOP('',(#11532,#11533,#11534,#11535,#11536,#11537,#11538,#11539));
#4919=EDGE_LOOP('',(#11540,#11541,#11542,#11543));
#4920=EDGE_LOOP('',(#11544,#11545,#11546,#11547));
#4921=EDGE_LOOP('',(#11548,#11549,#11550,#11551));
#4922=EDGE_LOOP('',(#11552,#11553,#11554,#11555,#11556,#11557,#11558,#11559,
#11560,#11561,#11562));
#4923=EDGE_LOOP('',(#11563,#11564,#11565,#11566,#11567));
#4924=EDGE_LOOP('',(#11568,#11569,#11570,#11571,#11572));
#4925=EDGE_LOOP('',(#11573,#11574,#11575,#11576,#11577));
#4926=EDGE_LOOP('',(#11578,#11579,#11580,#11581,#11582));
#4927=EDGE_LOOP('',(#11583,#11584,#11585,#11586,#11587,#11588,#11589,#11590,
#11591,#11592,#11593,#11594,#11595,#11596,#11597,#11598,#11599,#11600));
#4928=EDGE_LOOP('',(#11601,#11602,#11603,#11604,#11605,#11606,#11607));
#4929=EDGE_LOOP('',(#11608,#11609,#11610,#11611));
#4930=EDGE_LOOP('',(#11612,#11613,#11614,#11615));
#4931=EDGE_LOOP('',(#11616,#11617,#11618,#11619));
#4932=EDGE_LOOP('',(#11620,#11621,#11622,#11623,#11624,#11625));
#4933=EDGE_LOOP('',(#11626,#11627,#11628,#11629,#11630));
#4934=EDGE_LOOP('',(#11631,#11632,#11633,#11634,#11635,#11636));
#4935=EDGE_LOOP('',(#11637,#11638,#11639,#11640));
#4936=EDGE_LOOP('',(#11641,#11642,#11643,#11644));
#4937=EDGE_LOOP('',(#11645,#11646));
#4938=EDGE_LOOP('',(#11647,#11648,#11649,#11650,#11651));
#4939=EDGE_LOOP('',(#11652,#11653,#11654,#11655,#11656));
#4940=EDGE_LOOP('',(#11657,#11658));
#4941=EDGE_LOOP('',(#11659,#11660,#11661,#11662,#11663,#11664));
#4942=EDGE_LOOP('',(#11665,#11666,#11667,#11668));
#4943=EDGE_LOOP('',(#11669,#11670,#11671,#11672));
#4944=EDGE_LOOP('',(#11673,#11674,#11675,#11676));
#4945=EDGE_LOOP('',(#11677,#11678,#11679,#11680));
#4946=EDGE_LOOP('',(#11681,#11682,#11683,#11684));
#4947=EDGE_LOOP('',(#11685,#11686,#11687,#11688));
#4948=EDGE_LOOP('',(#11689,#11690,#11691,#11692));
#4949=EDGE_LOOP('',(#11693,#11694,#11695));
#4950=EDGE_LOOP('',(#11696,#11697,#11698,#11699));
#4951=EDGE_LOOP('',(#11700,#11701,#11702,#11703));
#4952=EDGE_LOOP('',(#11704,#11705,#11706,#11707));
#4953=EDGE_LOOP('',(#11708,#11709,#11710,#11711));
#4954=EDGE_LOOP('',(#11712,#11713,#11714,#11715));
#4955=EDGE_LOOP('',(#11716,#11717,#11718,#11719));
#4956=EDGE_LOOP('',(#11720,#11721,#11722,#11723));
#4957=EDGE_LOOP('',(#11724,#11725,#11726,#11727));
#4958=EDGE_LOOP('',(#11728,#11729,#11730,#11731));
#4959=EDGE_LOOP('',(#11732,#11733,#11734,#11735));
#4960=EDGE_LOOP('',(#11736,#11737,#11738,#11739));
#4961=EDGE_LOOP('',(#11740,#11741,#11742,#11743));
#4962=EDGE_LOOP('',(#11744,#11745,#11746,#11747));
#4963=EDGE_LOOP('',(#11748,#11749,#11750,#11751));
#4964=EDGE_LOOP('',(#11752,#11753,#11754,#11755,#11756));
#4965=EDGE_LOOP('',(#11757,#11758,#11759,#11760,#11761,#11762));
#4966=EDGE_LOOP('',(#11763,#11764,#11765));
#4967=EDGE_LOOP('',(#11766,#11767,#11768,#11769));
#4968=EDGE_LOOP('',(#11770,#11771,#11772,#11773,#11774,#11775));
#4969=EDGE_LOOP('',(#11776,#11777,#11778));
#4970=EDGE_LOOP('',(#11779,#11780,#11781));
#4971=EDGE_LOOP('',(#11782,#11783,#11784));
#4972=EDGE_LOOP('',(#11785,#11786,#11787,#11788));
#4973=EDGE_LOOP('',(#11789,#11790,#11791,#11792));
#4974=EDGE_LOOP('',(#11793,#11794,#11795,#11796,#11797));
#4975=EDGE_LOOP('',(#11798,#11799,#11800,#11801));
#4976=EDGE_LOOP('',(#11802,#11803,#11804,#11805));
#4977=EDGE_LOOP('',(#11806,#11807,#11808,#11809,#11810,#11811));
#4978=EDGE_LOOP('',(#11812,#11813,#11814,#11815,#11816));
#4979=EDGE_LOOP('',(#11817,#11818,#11819,#11820));
#4980=EDGE_LOOP('',(#11821));
#4981=EDGE_LOOP('',(#11822,#11823));
#4982=EDGE_LOOP('',(#11824,#11825,#11826,#11827));
#4983=EDGE_LOOP('',(#11828,#11829,#11830,#11831,#11832));
#4984=EDGE_LOOP('',(#11833,#11834,#11835,#11836,#11837));
#4985=EDGE_LOOP('',(#11838,#11839,#11840,#11841));
#4986=EDGE_LOOP('',(#11842,#11843,#11844,#11845));
#4987=EDGE_LOOP('',(#11846,#11847,#11848,#11849));
#4988=EDGE_LOOP('',(#11850,#11851,#11852,#11853));
#4989=EDGE_LOOP('',(#11854,#11855,#11856,#11857));
#4990=EDGE_LOOP('',(#11858,#11859,#11860,#11861,#11862));
#4991=EDGE_LOOP('',(#11863,#11864,#11865,#11866));
#4992=EDGE_LOOP('',(#11867,#11868,#11869,#11870));
#4993=EDGE_LOOP('',(#11871,#11872,#11873,#11874));
#4994=EDGE_LOOP('',(#11875,#11876,#11877,#11878));
#4995=EDGE_LOOP('',(#11879,#11880,#11881,#11882,#11883));
#4996=EDGE_LOOP('',(#11884,#11885,#11886));
#4997=EDGE_LOOP('',(#11887,#11888,#11889,#11890));
#4998=EDGE_LOOP('',(#11891,#11892,#11893,#11894,#11895,#11896,#11897,#11898));
#4999=EDGE_LOOP('',(#11899,#11900,#11901,#11902));
#5000=EDGE_LOOP('',(#11903,#11904,#11905,#11906));
#5001=EDGE_LOOP('',(#11907,#11908,#11909,#11910));
#5002=EDGE_LOOP('',(#11911,#11912,#11913,#11914));
#5003=EDGE_LOOP('',(#11915,#11916,#11917,#11918));
#5004=EDGE_LOOP('',(#11919,#11920,#11921,#11922));
#5005=EDGE_LOOP('',(#11923,#11924,#11925,#11926));
#5006=EDGE_LOOP('',(#11927,#11928,#11929,#11930));
#5007=EDGE_LOOP('',(#11931,#11932,#11933,#11934,#11935));
#5008=EDGE_LOOP('',(#11936,#11937,#11938,#11939,#11940));
#5009=EDGE_LOOP('',(#11941,#11942,#11943,#11944,#11945,#11946,#11947,#11948));
#5010=EDGE_LOOP('',(#11949,#11950,#11951));
#5011=EDGE_LOOP('',(#11952,#11953,#11954,#11955,#11956,#11957));
#5012=EDGE_LOOP('',(#11958,#11959,#11960,#11961));
#5013=EDGE_LOOP('',(#11962,#11963,#11964,#11965));
#5014=EDGE_LOOP('',(#11966,#11967,#11968,#11969));
#5015=EDGE_LOOP('',(#11970));
#5016=EDGE_LOOP('',(#11971,#11972,#11973,#11974,#11975,#11976,#11977,#11978));
#5017=EDGE_LOOP('',(#11979));
#5018=EDGE_LOOP('',(#11980,#11981,#11982,#11983));
#5019=EDGE_LOOP('',(#11984,#11985,#11986,#11987));
#5020=EDGE_LOOP('',(#11988,#11989,#11990,#11991));
#5021=EDGE_LOOP('',(#11992,#11993,#11994,#11995,#11996,#11997,#11998,#11999,
#12000,#12001,#12002,#12003,#12004,#12005,#12006));
#5022=EDGE_LOOP('',(#12007,#12008,#12009,#12010));
#5023=EDGE_LOOP('',(#12011,#12012,#12013,#12014));
#5024=EDGE_LOOP('',(#12015,#12016,#12017,#12018));
#5025=EDGE_LOOP('',(#12019,#12020,#12021,#12022));
#5026=EDGE_LOOP('',(#12023,#12024,#12025,#12026));
#5027=EDGE_LOOP('',(#12027,#12028,#12029,#12030));
#5028=EDGE_LOOP('',(#12031,#12032,#12033,#12034,#12035,#12036));
#5029=EDGE_LOOP('',(#12037,#12038,#12039,#12040));
#5030=EDGE_LOOP('',(#12041,#12042,#12043,#12044));
#5031=EDGE_LOOP('',(#12045,#12046,#12047,#12048));
#5032=EDGE_LOOP('',(#12049,#12050,#12051,#12052));
#5033=EDGE_LOOP('',(#12053,#12054,#12055,#12056));
#5034=EDGE_LOOP('',(#12057,#12058,#12059,#12060));
#5035=EDGE_LOOP('',(#12061,#12062,#12063,#12064,#12065));
#5036=EDGE_LOOP('',(#12066,#12067,#12068));
#5037=EDGE_LOOP('',(#12069,#12070,#12071,#12072,#12073));
#5038=EDGE_LOOP('',(#12074,#12075,#12076,#12077));
#5039=EDGE_LOOP('',(#12078,#12079,#12080,#12081,#12082));
#5040=EDGE_LOOP('',(#12083,#12084,#12085,#12086));
#5041=EDGE_LOOP('',(#12087,#12088,#12089,#12090));
#5042=EDGE_LOOP('',(#12091,#12092,#12093,#12094,#12095,#12096,#12097));
#5043=EDGE_LOOP('',(#12098));
#5044=EDGE_LOOP('',(#12099,#12100,#12101,#12102,#12103));
#5045=EDGE_LOOP('',(#12104,#12105,#12106,#12107,#12108));
#5046=EDGE_LOOP('',(#12109,#12110,#12111,#12112));
#5047=EDGE_LOOP('',(#12113,#12114,#12115,#12116));
#5048=EDGE_LOOP('',(#12117,#12118,#12119,#12120));
#5049=EDGE_LOOP('',(#12121,#12122,#12123,#12124,#12125,#12126,#12127,#12128,
#12129,#12130,#12131,#12132,#12133,#12134,#12135,#12136,#12137,#12138,#12139,
#12140,#12141,#12142,#12143,#12144,#12145,#12146,#12147,#12148,#12149,#12150,
#12151));
#5050=EDGE_LOOP('',(#12152));
#5051=EDGE_LOOP('',(#12153,#12154,#12155,#12156,#12157));
#5052=EDGE_LOOP('',(#12158,#12159,#12160,#12161));
#5053=EDGE_LOOP('',(#12162,#12163,#12164,#12165));
#5054=EDGE_LOOP('',(#12166,#12167,#12168,#12169));
#5055=EDGE_LOOP('',(#12170,#12171,#12172,#12173));
#5056=EDGE_LOOP('',(#12174,#12175,#12176,#12177));
#5057=EDGE_LOOP('',(#12178,#12179,#12180,#12181));
#5058=EDGE_LOOP('',(#12182,#12183,#12184,#12185));
#5059=EDGE_LOOP('',(#12186,#12187,#12188,#12189));
#5060=EDGE_LOOP('',(#12190,#12191,#12192,#12193));
#5061=EDGE_LOOP('',(#12194,#12195,#12196,#12197));
#5062=EDGE_LOOP('',(#12198,#12199,#12200,#12201));
#5063=EDGE_LOOP('',(#12202,#12203,#12204,#12205,#12206));
#5064=EDGE_LOOP('',(#12207,#12208,#12209,#12210,#12211));
#5065=EDGE_LOOP('',(#12212,#12213,#12214,#12215,#12216,#12217));
#5066=EDGE_LOOP('',(#12218,#12219,#12220,#12221,#12222));
#5067=EDGE_LOOP('',(#12223,#12224,#12225,#12226));
#5068=EDGE_LOOP('',(#12227,#12228,#12229,#12230));
#5069=EDGE_LOOP('',(#12231,#12232,#12233,#12234));
#5070=EDGE_LOOP('',(#12235));
#5071=EDGE_LOOP('',(#12236));
#5696=CIRCLE('',#15860,0.800000000000002);
#5697=CIRCLE('',#15861,0.800000000000002);
#5698=CIRCLE('',#15862,8.2);
#5699=CIRCLE('',#15863,0.800000000000002);
#5700=CIRCLE('',#15864,0.800000000000002);
#5701=CIRCLE('',#15865,0.800000000000002);
#5702=CIRCLE('',#15866,0.800000000000002);
#5703=CIRCLE('',#15868,0.799999999999999);
#5704=CIRCLE('',#15869,0.799999999999999);
#5705=CIRCLE('',#15870,0.799999999999999);
#5706=CIRCLE('',#15871,0.799999999999999);
#5707=CIRCLE('',#15872,8.2);
#5708=CIRCLE('',#15873,0.799999999999999);
#5709=CIRCLE('',#15874,0.799999999999999);
#5710=CIRCLE('',#15876,2.7);
#5711=CIRCLE('',#15877,0.800000000000002);
#5712=CIRCLE('',#15879,0.799999999999999);
#5713=CIRCLE('',#15880,3.2);
#5714=CIRCLE('',#15882,0.800000000000002);
#5715=CIRCLE('',#15883,1.2);
#5716=CIRCLE('',#15885,14.2);
#5717=CIRCLE('',#15886,0.799999999999999);
#5718=CIRCLE('',#15888,4.);
#5719=CIRCLE('',#15889,4.);
#5720=CIRCLE('',#15891,4.);
#5721=CIRCLE('',#15892,4.);
#5722=CIRCLE('',#15893,3.7);
#5723=CIRCLE('',#15895,4.);
#5724=CIRCLE('',#15896,4.);
#5725=CIRCLE('',#15898,2.8);
#5726=CIRCLE('',#15899,2.8);
#5727=CIRCLE('',#15900,2.8);
#5728=CIRCLE('',#15901,2.8);
#5729=CIRCLE('',#15902,2.8);
#5730=CIRCLE('',#15903,2.8);
#5731=CIRCLE('',#15904,2.8);
#5732=CIRCLE('',#15906,2.5);
#5733=CIRCLE('',#15907,2.5);
#5734=CIRCLE('',#15908,2.5);
#5735=CIRCLE('',#15909,2.5);
#5736=CIRCLE('',#15910,2.5);
#5737=CIRCLE('',#15912,4.5);
#5738=CIRCLE('',#15913,0.5);
#5739=CIRCLE('',#15915,10.5);
#5740=CIRCLE('',#15916,10.);
#5741=CIRCLE('',#15918,6.5);
#5742=CIRCLE('',#15919,6.);
#5743=CIRCLE('',#15921,17.);
#5744=CIRCLE('',#15922,17.);
#5745=CIRCLE('',#15924,17.);
#5746=CIRCLE('',#15925,17.);
#5747=CIRCLE('',#15927,17.);
#5748=CIRCLE('',#15928,17.);
#5749=CIRCLE('',#15929,17.);
#5750=CIRCLE('',#15931,3.8);
#5751=CIRCLE('',#15932,3.3);
#5752=CIRCLE('',#15933,3.3);
#5753=CIRCLE('',#15935,4.);
#5754=CIRCLE('',#15936,0.5);
#5755=CIRCLE('',#15937,4.5);
#5756=CIRCLE('',#15938,0.5);
#5757=CIRCLE('',#15940,1.);
#5758=CIRCLE('',#15941,1.5);
#5759=CIRCLE('',#15943,1.5);
#5760=CIRCLE('',#15944,1.5);
#5761=CIRCLE('',#15946,3.8);
#5762=CIRCLE('',#15947,3.8);
#5763=CIRCLE('',#15948,3.8);
#5764=CIRCLE('',#15949,3.8);
#5765=CIRCLE('',#15951,0.499999999999999);
#5766=CIRCLE('',#15952,0.499999999999999);
#5767=CIRCLE('',#15954,1.);
#5768=CIRCLE('',#15955,1.);
#5769=CIRCLE('',#15957,16.5);
#5770=CIRCLE('',#15958,0.499999999999999);
#5771=CIRCLE('',#15960,3.);
#5772=CIRCLE('',#15962,2.5);
#5773=CIRCLE('',#15963,2.5);
#5774=CIRCLE('',#15964,2.5);
#5775=CIRCLE('',#15965,2.5);
#5776=CIRCLE('',#15966,2.5);
#5777=CIRCLE('',#15967,2.5);
#5778=CIRCLE('',#15972,3.);
#5779=CIRCLE('',#15973,0.499999999999997);
#5780=CIRCLE('',#15975,5.5);
#5781=CIRCLE('',#15976,6.);
#5782=CIRCLE('',#15978,10.5);
#5783=CIRCLE('',#15979,11.);
#5784=CIRCLE('',#15980,0.499999999999988);
#5785=CIRCLE('',#15981,0.499999999999996);
#5786=CIRCLE('',#15982,0.499999999999997);
#5787=CIRCLE('',#15983,0.49999999999999);
#5788=CIRCLE('',#15999,11.);
#5789=CIRCLE('',#16000,10.5);
#5790=CIRCLE('',#16006,6.);
#5791=CIRCLE('',#16007,6.5);
#5792=CIRCLE('',#16009,0.5);
#5793=CIRCLE('',#16010,1.5);
#5794=CIRCLE('',#16011,0.500000000000001);
#5795=CIRCLE('',#16012,1.);
#5796=CIRCLE('',#16015,18.);
#5797=CIRCLE('',#16017,0.5);
#5798=CIRCLE('',#16020,0.5);
#5799=CIRCLE('',#16026,3.);
#5800=CIRCLE('',#16028,1.);
#5801=CIRCLE('',#16029,1.);
#5802=CIRCLE('',#16034,0.500000000000002);
#5803=CIRCLE('',#16035,3.);
#5804=CIRCLE('',#16037,0.5);
#5805=CIRCLE('',#16042,0.5);
#5806=CIRCLE('',#16047,1.5);
#5807=CIRCLE('',#16049,16.5);
#5808=CIRCLE('',#16050,0.499999999999999);
#5809=CIRCLE('',#16052,16.5);
#5810=CIRCLE('',#16053,0.500000000000001);
#5811=CIRCLE('',#16055,3.);
#5812=CIRCLE('',#16056,0.499999999999999);
#5813=CIRCLE('',#16060,14.5);
#5814=CIRCLE('',#16061,13.5);
#5815=CIRCLE('',#16063,10.5);
#5816=CIRCLE('',#16064,10.5);
#5817=CIRCLE('',#16067,10.);
#5818=CIRCLE('',#16068,0.500000000000001);
#5819=CIRCLE('',#16070,1.);
#5820=CIRCLE('',#16071,1.);
#5821=CIRCLE('',#16073,1.);
#5822=CIRCLE('',#16074,1.);
#5823=CIRCLE('',#16076,1.);
#5824=CIRCLE('',#16087,1.5);
#5825=CIRCLE('',#16088,0.5);
#5826=CIRCLE('',#16090,0.5);
#5827=CIRCLE('',#16091,4.3);
#5828=CIRCLE('',#16094,3.8);
#5829=CIRCLE('',#16095,3.8);
#5830=CIRCLE('',#16097,1.5);
#5831=CIRCLE('',#16098,1.5);
#5832=CIRCLE('',#16100,1.);
#5833=CIRCLE('',#16103,5.5);
#5834=CIRCLE('',#16104,6.);
#5835=CIRCLE('',#16105,11.);
#5836=CIRCLE('',#16106,5.5);
#5837=CIRCLE('',#16108,1.);
#5838=CIRCLE('',#16109,4.5);
#5839=CIRCLE('',#16112,10.5);
#5840=CIRCLE('',#16114,10.5);
#5841=CIRCLE('',#16115,10.5);
#5842=CIRCLE('',#16117,14.5);
#5843=CIRCLE('',#16118,6.5);
#5844=CIRCLE('',#16120,6.5);
#5845=CIRCLE('',#16121,10.);
#5846=CIRCLE('',#16123,10.);
#5847=CIRCLE('',#16126,6.);
#5848=CIRCLE('',#16127,6.);
#5849=CIRCLE('',#16130,6.);
#5850=CIRCLE('',#16131,6.);
#5851=CIRCLE('',#16148,1.50083490556055);
#5852=CIRCLE('',#16151,0.5);
#5853=CIRCLE('',#16166,13.5);
#6724=VERTEX_POINT('',#35151);
#6725=VERTEX_POINT('',#35152);
#6726=VERTEX_POINT('',#35155);
#6727=VERTEX_POINT('',#35157);
#6728=VERTEX_POINT('',#35159);
#6729=VERTEX_POINT('',#35161);
#6730=VERTEX_POINT('',#35165);
#6731=VERTEX_POINT('',#35166);
#6732=VERTEX_POINT('',#35168);
#6733=VERTEX_POINT('',#35170);
#6734=VERTEX_POINT('',#35173);
#6735=VERTEX_POINT('',#35175);
#6736=VERTEX_POINT('',#35179);
#6737=VERTEX_POINT('',#35180);
#6738=VERTEX_POINT('',#35197);
#6739=VERTEX_POINT('',#35226);
#6740=VERTEX_POINT('',#35265);
#6741=VERTEX_POINT('',#35308);
#6742=VERTEX_POINT('',#35361);
#6743=VERTEX_POINT('',#35365);
#6744=VERTEX_POINT('',#35367);
#6745=VERTEX_POINT('',#35369);
#6746=VERTEX_POINT('',#35413);
#6747=VERTEX_POINT('',#35451);
#6748=VERTEX_POINT('',#35539);
#6749=VERTEX_POINT('',#35543);
#6750=VERTEX_POINT('',#35547);
#6751=VERTEX_POINT('',#35549);
#6752=VERTEX_POINT('',#35553);
#6753=VERTEX_POINT('',#35554);
#6754=VERTEX_POINT('',#35557);
#6755=VERTEX_POINT('',#35561);
#6756=VERTEX_POINT('',#35562);
#6757=VERTEX_POINT('',#35567);
#6758=VERTEX_POINT('',#35568);
#6759=VERTEX_POINT('',#35570);
#6760=VERTEX_POINT('',#35572);
#6761=VERTEX_POINT('',#35574);
#6762=VERTEX_POINT('',#35576);
#6763=VERTEX_POINT('',#35578);
#6764=VERTEX_POINT('',#35591);
#6765=VERTEX_POINT('',#35593);
#6766=VERTEX_POINT('',#35606);
#6767=VERTEX_POINT('',#35608);
#6768=VERTEX_POINT('',#35610);
#6769=VERTEX_POINT('',#35612);
#6770=VERTEX_POINT('',#35617);
#6771=VERTEX_POINT('',#35619);
#6772=VERTEX_POINT('',#35621);
#6773=VERTEX_POINT('',#35623);
#6774=VERTEX_POINT('',#35625);
#6775=VERTEX_POINT('',#35644);
#6776=VERTEX_POINT('',#35646);
#6777=VERTEX_POINT('',#35648);
#6778=VERTEX_POINT('',#35678);
#6779=VERTEX_POINT('',#35716);
#6780=VERTEX_POINT('',#35718);
#6781=VERTEX_POINT('',#35720);
#6782=VERTEX_POINT('',#35727);
#6783=VERTEX_POINT('',#35763);
#6784=VERTEX_POINT('',#35767);
#6785=VERTEX_POINT('',#35768);
#6786=VERTEX_POINT('',#35770);
#6787=VERTEX_POINT('',#35785);
#6788=VERTEX_POINT('',#35802);
#6789=VERTEX_POINT('',#35803);
#6790=VERTEX_POINT('',#35805);
#6791=VERTEX_POINT('',#35820);
#6792=VERTEX_POINT('',#35837);
#6793=VERTEX_POINT('',#35838);
#6794=VERTEX_POINT('',#35840);
#6795=VERTEX_POINT('',#35842);
#6796=VERTEX_POINT('',#35846);
#6797=VERTEX_POINT('',#35848);
#6798=VERTEX_POINT('',#35931);
#6799=VERTEX_POINT('',#36014);
#6800=VERTEX_POINT('',#36016);
#6801=VERTEX_POINT('',#36057);
#6802=VERTEX_POINT('',#36059);
#6803=VERTEX_POINT('',#36061);
#6804=VERTEX_POINT('',#36072);
#6805=VERTEX_POINT('',#36074);
#6806=VERTEX_POINT('',#36076);
#6807=VERTEX_POINT('',#36078);
#6808=VERTEX_POINT('',#36082);
#6809=VERTEX_POINT('',#36101);
#6810=VERTEX_POINT('',#36103);
#6811=VERTEX_POINT('',#36118);
#6812=VERTEX_POINT('',#36120);
#6813=VERTEX_POINT('',#36135);
#6814=VERTEX_POINT('',#36136);
#6815=VERTEX_POINT('',#36138);
#6816=VERTEX_POINT('',#36140);
#6817=VERTEX_POINT('',#36144);
#6818=VERTEX_POINT('',#36148);
#6819=VERTEX_POINT('',#36150);
#6820=VERTEX_POINT('',#36154);
#6821=VERTEX_POINT('',#36156);
#6822=VERTEX_POINT('',#36158);
#6823=VERTEX_POINT('',#36160);
#6824=VERTEX_POINT('',#36345);
#6825=VERTEX_POINT('',#36348);
#6826=VERTEX_POINT('',#36350);
#6827=VERTEX_POINT('',#36354);
#6828=VERTEX_POINT('',#36356);
#6829=VERTEX_POINT('',#36358);
#6830=VERTEX_POINT('',#36362);
#6831=VERTEX_POINT('',#36364);
#6832=VERTEX_POINT('',#36368);
#6833=VERTEX_POINT('',#36369);
#6834=VERTEX_POINT('',#36371);
#6835=VERTEX_POINT('',#36392);
#6836=VERTEX_POINT('',#36397);
#6837=VERTEX_POINT('',#36414);
#6838=VERTEX_POINT('',#36415);
#6839=VERTEX_POINT('',#36417);
#6840=VERTEX_POINT('',#36512);
#6841=VERTEX_POINT('',#36537);
#6842=VERTEX_POINT('',#36581);
#6843=VERTEX_POINT('',#36583);
#6844=VERTEX_POINT('',#36585);
#6845=VERTEX_POINT('',#36596);
#6846=VERTEX_POINT('',#36598);
#6847=VERTEX_POINT('',#36600);
#6848=VERTEX_POINT('',#36602);
#6849=VERTEX_POINT('',#36604);
#6850=VERTEX_POINT('',#36606);
#6851=VERTEX_POINT('',#36608);
#6852=VERTEX_POINT('',#36610);
#6853=VERTEX_POINT('',#36612);
#6854=VERTEX_POINT('',#36633);
#6855=VERTEX_POINT('',#36635);
#6856=VERTEX_POINT('',#36640);
#6857=VERTEX_POINT('',#36674);
#6858=VERTEX_POINT('',#36676);
#6859=VERTEX_POINT('',#36680);
#6860=VERTEX_POINT('',#36695);
#6861=VERTEX_POINT('',#36699);
#6862=VERTEX_POINT('',#36700);
#6863=VERTEX_POINT('',#36702);
#6864=VERTEX_POINT('',#36717);
#6865=VERTEX_POINT('',#36734);
#6866=VERTEX_POINT('',#36735);
#6867=VERTEX_POINT('',#36737);
#6868=VERTEX_POINT('',#36750);
#6869=VERTEX_POINT('',#38297);
#6870=VERTEX_POINT('',#38299);
#6871=VERTEX_POINT('',#38959);
#6872=VERTEX_POINT('',#38961);
#6873=VERTEX_POINT('',#41335);
#6874=VERTEX_POINT('',#41337);
#6875=VERTEX_POINT('',#41349);
#6876=VERTEX_POINT('',#41350);
#6877=VERTEX_POINT('',#41352);
#6878=VERTEX_POINT('',#41354);
#6879=VERTEX_POINT('',#41358);
#6880=VERTEX_POINT('',#41359);
#6881=VERTEX_POINT('',#41361);
#6882=VERTEX_POINT('',#41363);
#6883=VERTEX_POINT('',#41367);
#6884=VERTEX_POINT('',#41368);
#6885=VERTEX_POINT('',#41370);
#6886=VERTEX_POINT('',#41372);
#6887=VERTEX_POINT('',#41382);
#6888=VERTEX_POINT('',#41399);
#6889=VERTEX_POINT('',#41415);
#6890=VERTEX_POINT('',#41432);
#6891=VERTEX_POINT('',#41453);
#6892=VERTEX_POINT('',#41468);
#6893=VERTEX_POINT('',#41470);
#6894=VERTEX_POINT('',#41487);
#6895=VERTEX_POINT('',#41488);
#6896=VERTEX_POINT('',#41490);
#6897=VERTEX_POINT('',#41492);
#6898=VERTEX_POINT('',#41499);
#6899=VERTEX_POINT('',#41500);
#6900=VERTEX_POINT('',#41502);
#6901=VERTEX_POINT('',#41504);
#6902=VERTEX_POINT('',#41633);
#6903=VERTEX_POINT('',#41634);
#6904=VERTEX_POINT('',#41645);
#6905=VERTEX_POINT('',#41647);
#6906=VERTEX_POINT('',#41651);
#6907=VERTEX_POINT('',#41653);
#6908=VERTEX_POINT('',#41956);
#6909=VERTEX_POINT('',#41960);
#6910=VERTEX_POINT('',#41963);
#6911=VERTEX_POINT('',#41970);
#6912=VERTEX_POINT('',#41985);
#6913=VERTEX_POINT('',#41998);
#6914=VERTEX_POINT('',#42000);
#6915=VERTEX_POINT('',#42009);
#6916=VERTEX_POINT('',#42013);
#6917=VERTEX_POINT('',#42015);
#6918=VERTEX_POINT('',#42032);
#6919=VERTEX_POINT('',#42233);
#6920=VERTEX_POINT('',#42234);
#6921=VERTEX_POINT('',#42398);
#6922=VERTEX_POINT('',#42412);
#6923=VERTEX_POINT('',#42517);
#6924=VERTEX_POINT('',#42642);
#6925=VERTEX_POINT('',#42763);
#6926=VERTEX_POINT('',#42868);
#6927=VERTEX_POINT('',#42972);
#6928=VERTEX_POINT('',#43116);
#6929=VERTEX_POINT('',#43120);
#6930=VERTEX_POINT('',#43122);
#6931=VERTEX_POINT('',#43135);
#6932=VERTEX_POINT('',#43137);
#6933=VERTEX_POINT('',#43139);
#6934=VERTEX_POINT('',#43143);
#6935=VERTEX_POINT('',#43144);
#6936=VERTEX_POINT('',#43146);
#6937=VERTEX_POINT('',#43178);
#6938=VERTEX_POINT('',#43185);
#6939=VERTEX_POINT('',#43186);
#6940=VERTEX_POINT('',#43191);
#6941=VERTEX_POINT('',#43195);
#6942=VERTEX_POINT('',#43201);
#6943=VERTEX_POINT('',#43202);
#6944=VERTEX_POINT('',#43205);
#6945=VERTEX_POINT('',#43209);
#6946=VERTEX_POINT('',#43210);
#6947=VERTEX_POINT('',#43212);
#6948=VERTEX_POINT('',#43214);
#6949=VERTEX_POINT('',#43222);
#6950=VERTEX_POINT('',#43224);
#6951=VERTEX_POINT('',#43228);
#6952=VERTEX_POINT('',#43285);
#6953=VERTEX_POINT('',#43351);
#6954=VERTEX_POINT('',#43364);
#6955=VERTEX_POINT('',#43379);
#6956=VERTEX_POINT('',#43396);
#6957=VERTEX_POINT('',#43400);
#6958=VERTEX_POINT('',#43731);
#6959=VERTEX_POINT('',#43752);
#6960=VERTEX_POINT('',#43754);
#6961=VERTEX_POINT('',#43757);
#6962=VERTEX_POINT('',#43758);
#6963=VERTEX_POINT('',#43760);
#6964=VERTEX_POINT('',#43762);
#6965=VERTEX_POINT('',#43784);
#6966=VERTEX_POINT('',#43786);
#6967=VERTEX_POINT('',#43791);
#6968=VERTEX_POINT('',#43793);
#6969=VERTEX_POINT('',#43797);
#6970=VERTEX_POINT('',#43798);
#6971=VERTEX_POINT('',#43800);
#6972=VERTEX_POINT('',#43802);
#6973=VERTEX_POINT('',#43806);
#6974=VERTEX_POINT('',#43808);
#6975=VERTEX_POINT('',#43813);
#6976=VERTEX_POINT('',#43918);
#6977=VERTEX_POINT('',#43976);
#6978=VERTEX_POINT('',#43978);
#6979=VERTEX_POINT('',#44426);
#8412=EDGE_CURVE('',#6724,#6725,#5696,.T.);
#8413=EDGE_CURVE('',#6725,#6724,#5697,.T.);
#8414=EDGE_CURVE('',#6724,#6726,#5698,.T.);
#8415=EDGE_CURVE('',#6726,#6727,#5699,.T.);
#8416=EDGE_CURVE('',#6727,#6728,#5700,.T.);
#8417=EDGE_CURVE('',#6728,#6729,#5701,.T.);
#8418=EDGE_CURVE('',#6729,#6726,#5702,.T.);
#8419=EDGE_CURVE('',#6730,#6731,#5703,.T.);
#8420=EDGE_CURVE('',#6732,#6730,#5704,.T.);
#8421=EDGE_CURVE('',#6733,#6732,#5705,.T.);
#8422=EDGE_CURVE('',#6731,#6733,#5706,.T.);
#8423=EDGE_CURVE('',#6731,#6734,#5707,.T.);
#8424=EDGE_CURVE('',#6735,#6734,#5708,.T.);
#8425=EDGE_CURVE('',#6734,#6735,#5709,.T.);
#8426=EDGE_CURVE('',#6736,#6737,#798,.T.);
#8427=EDGE_CURVE('',#6736,#6738,#799,.T.);
#8428=EDGE_CURVE('',#6738,#6739,#800,.T.);
#8429=EDGE_CURVE('',#6739,#6740,#801,.T.);
#8430=EDGE_CURVE('',#6740,#6741,#802,.T.);
#8431=EDGE_CURVE('',#6737,#6741,#803,.T.);
#8432=EDGE_CURVE('',#6737,#6742,#5710,.T.);
#8433=EDGE_CURVE('',#6742,#6742,#5711,.T.);
#8434=EDGE_CURVE('',#6743,#6743,#5712,.T.);
#8435=EDGE_CURVE('',#6743,#6744,#5713,.T.);
#8436=EDGE_CURVE('',#6744,#6745,#804,.T.);
#8437=EDGE_CURVE('',#6745,#6746,#805,.T.);
#8438=EDGE_CURVE('',#6746,#6747,#806,.T.);
#8439=EDGE_CURVE('',#6747,#6744,#807,.T.);
#8440=EDGE_CURVE('',#6748,#6748,#5714,.T.);
#8441=EDGE_CURVE('',#6748,#6725,#5715,.T.);
#8442=EDGE_CURVE('',#6735,#6749,#5716,.T.);
#8443=EDGE_CURVE('',#6749,#6749,#5717,.T.);
#8444=EDGE_CURVE('',#6750,#6750,#5718,.T.);
#8445=EDGE_CURVE('',#6750,#6751,#1636,.T.);
#8446=EDGE_CURVE('',#6751,#6751,#5719,.T.);
#8447=EDGE_CURVE('',#6752,#6753,#5720,.T.);
#8448=EDGE_CURVE('',#6753,#6752,#5721,.T.);
#8449=EDGE_CURVE('',#6753,#6754,#1637,.T.);
#8450=EDGE_CURVE('',#6754,#6754,#5722,.T.);
#8451=EDGE_CURVE('',#6755,#6756,#5723,.T.);
#8452=EDGE_CURVE('',#6756,#6755,#5724,.T.);
#8453=EDGE_CURVE('',#6755,#6752,#1638,.T.);
#8454=EDGE_CURVE('',#6757,#6758,#5725,.T.);
#8455=EDGE_CURVE('',#6758,#6759,#1639,.T.);
#8456=EDGE_CURVE('',#6759,#6760,#5726,.T.);
#8457=EDGE_CURVE('',#6761,#6760,#1640,.T.);
#8458=EDGE_CURVE('',#6761,#6762,#5727,.T.);
#8459=EDGE_CURVE('',#6762,#6763,#808,.T.);
#8460=EDGE_CURVE('',#6763,#6764,#1641,.T.);
#8461=EDGE_CURVE('',#6764,#6765,#809,.T.);
#8462=EDGE_CURVE('',#6765,#6766,#5728,.T.);
#8463=EDGE_CURVE('',#6767,#6766,#1642,.T.);
#8464=EDGE_CURVE('',#6767,#6768,#5729,.T.);
#8465=EDGE_CURVE('',#6768,#6769,#1643,.T.);
#8466=EDGE_CURVE('',#6769,#6759,#5730,.T.);
#8467=EDGE_CURVE('',#6758,#6757,#5731,.T.);
#8468=EDGE_CURVE('',#6770,#6770,#5732,.T.);
#8469=EDGE_CURVE('',#6770,#6771,#1644,.T.);
#8470=EDGE_CURVE('',#6771,#6772,#5733,.T.);
#8471=EDGE_CURVE('',#6772,#6773,#1645,.T.);
#8472=EDGE_CURVE('',#6773,#6774,#810,.T.);
#8473=EDGE_CURVE('',#6774,#6775,#1646,.T.);
#8474=EDGE_CURVE('',#6775,#6776,#5734,.T.);
#8475=EDGE_CURVE('',#6776,#6777,#811,.T.);
#8476=EDGE_CURVE('',#6777,#6778,#812,.T.);
#8477=EDGE_CURVE('',#6778,#6779,#1647,.T.);
#8478=EDGE_CURVE('',#6780,#6779,#5735,.T.);
#8479=EDGE_CURVE('',#6780,#6781,#813,.T.);
#8480=EDGE_CURVE('',#6782,#6781,#1648,.T.);
#8481=EDGE_CURVE('',#6782,#6771,#5736,.T.);
#8482=EDGE_CURVE('',#6741,#6736,#814,.T.);
#8483=EDGE_CURVE('',#6783,#6783,#5737,.T.);
#8484=EDGE_CURVE('',#6783,#6756,#5738,.T.);
#8485=EDGE_CURVE('',#6784,#6785,#5739,.T.);
#8486=EDGE_CURVE('',#6784,#6786,#815,.T.);
#8487=EDGE_CURVE('',#6787,#6786,#5740,.T.);
#8488=EDGE_CURVE('',#6787,#6785,#816,.T.);
#8489=EDGE_CURVE('',#6788,#6789,#5741,.T.);
#8490=EDGE_CURVE('',#6790,#6788,#817,.T.);
#8491=EDGE_CURVE('',#6791,#6790,#5742,.T.);
#8492=EDGE_CURVE('',#6789,#6791,#818,.T.);
#8493=EDGE_CURVE('',#6792,#6793,#5743,.T.);
#8494=EDGE_CURVE('',#6793,#6794,#1649,.T.);
#8495=EDGE_CURVE('',#6794,#6795,#5744,.T.);
#8496=EDGE_CURVE('',#6795,#6792,#1650,.T.);
#8497=EDGE_CURVE('',#6778,#6796,#5745,.T.);
#8498=EDGE_CURVE('',#6796,#6797,#819,.T.);
#8499=EDGE_CURVE('',#6797,#6798,#820,.T.);
#8500=EDGE_CURVE('',#6798,#6799,#5746,.T.);
#8501=EDGE_CURVE('',#6799,#6800,#821,.T.);
#8502=EDGE_CURVE('',#6800,#6801,#755,.T.);
#8503=EDGE_CURVE('',#6801,#6802,#1651,.T.);
#8504=EDGE_CURVE('',#6802,#6803,#822,.T.);
#8505=EDGE_CURVE('',#6803,#6804,#5747,.T.);
#8506=EDGE_CURVE('',#6804,#6805,#1652,.T.);
#8507=EDGE_CURVE('',#6806,#6805,#5748,.T.);
#8508=EDGE_CURVE('',#6806,#6807,#1653,.T.);
#8509=EDGE_CURVE('',#6779,#6807,#5749,.T.);
#8510=EDGE_CURVE('',#6808,#6769,#823,.T.);
#8511=EDGE_CURVE('',#6809,#6808,#5750,.T.);
#8512=EDGE_CURVE('',#6810,#6809,#824,.T.);
#8513=EDGE_CURVE('',#6811,#6810,#5751,.T.);
#8514=EDGE_CURVE('',#6812,#6811,#5752,.T.);
#8515=EDGE_CURVE('',#6760,#6812,#825,.F.);
#8516=EDGE_CURVE('',#6813,#6814,#5753,.T.);
#8517=EDGE_CURVE('',#6815,#6813,#5754,.T.);
#8518=EDGE_CURVE('',#6816,#6815,#5755,.T.);
#8519=EDGE_CURVE('',#6816,#6814,#5756,.T.);
#8520=EDGE_CURVE('',#6770,#6817,#5757,.T.);
#8521=EDGE_CURVE('',#6817,#6817,#5758,.T.);
#8522=EDGE_CURVE('',#6818,#6818,#5759,.T.);
#8523=EDGE_CURVE('',#6818,#6819,#1654,.T.);
#8524=EDGE_CURVE('',#6819,#6819,#5760,.T.);
#8525=EDGE_CURVE('',#6820,#6807,#5761,.T.);
#8526=EDGE_CURVE('',#6821,#6806,#5762,.T.);
#8527=EDGE_CURVE('',#6821,#6822,#1655,.T.);
#8528=EDGE_CURVE('',#6822,#6823,#826,.T.);
#8529=EDGE_CURVE('',#6823,#6824,#5763,.T.);
#8530=EDGE_CURVE('',#6824,#6809,#1656,.T.);
#8531=EDGE_CURVE('',#6825,#6808,#1657,.T.);
#8532=EDGE_CURVE('',#6825,#6826,#5764,.T.);
#8533=EDGE_CURVE('',#6820,#6826,#1658,.T.);
#8534=EDGE_CURVE('',#6827,#6773,#1659,.T.);
#8535=EDGE_CURVE('',#6828,#6827,#5765,.T.);
#8536=EDGE_CURVE('',#6829,#6828,#5766,.T.);
#8537=EDGE_CURVE('',#6774,#6829,#1660,.T.);
#8538=EDGE_CURVE('',#6761,#6830,#5767,.T.);
#8539=EDGE_CURVE('',#6831,#6812,#5768,.T.);
#8540=EDGE_CURVE('',#6830,#6831,#1661,.T.);
#8541=EDGE_CURVE('',#6832,#6833,#5769,.T.);
#8542=EDGE_CURVE('',#6832,#6834,#827,.T.);
#8543=EDGE_CURVE('',#6795,#6834,#828,.F.);
#8544=EDGE_CURVE('',#6833,#6794,#5770,.T.);
#8545=EDGE_CURVE('',#6835,#6782,#829,.T.);
#8546=EDGE_CURVE('',#6836,#6835,#5771,.T.);
#8547=EDGE_CURVE('',#6772,#6836,#830,.T.);
#8548=EDGE_CURVE('',#6837,#6838,#5772,.T.);
#8549=EDGE_CURVE('',#6838,#6839,#831,.T.);
#8550=EDGE_CURVE('',#6797,#6839,#832,.T.);
#8551=EDGE_CURVE('',#6840,#6797,#833,.T.);
#8552=EDGE_CURVE('',#6840,#6841,#834,.T.);
#8553=EDGE_CURVE('',#6841,#6842,#5773,.T.);
#8554=EDGE_CURVE('',#6843,#6842,#1662,.T.);
#8555=EDGE_CURVE('',#6843,#6844,#835,.T.);
#8556=EDGE_CURVE('',#6845,#6844,#5774,.T.);
#8557=EDGE_CURVE('',#6846,#6845,#1663,.T.);
#8558=EDGE_CURVE('',#6846,#6847,#5775,.T.);
#8559=EDGE_CURVE('',#6848,#6847,#1664,.T.);
#8560=EDGE_CURVE('',#6849,#6848,#5776,.T.);
#8561=EDGE_CURVE('',#6849,#6850,#1665,.T.);
#8562=EDGE_CURVE('',#6850,#6851,#5777,.T.);
#8563=EDGE_CURVE('',#6851,#6852,#1666,.T.);
#8564=EDGE_CURVE('',#6852,#6853,#836,.T.);
#8565=EDGE_CURVE('',#6837,#6853,#1667,.T.);
#8566=EDGE_CURVE('',#6854,#6852,#1668,.T.);
#8567=EDGE_CURVE('',#6855,#6854,#837,.T.);
#8568=EDGE_CURVE('',#6856,#6855,#838,.T.);
#8569=EDGE_CURVE('',#6856,#6857,#756,.T.);
#8570=EDGE_CURVE('',#6857,#6858,#757,.T.);
#8571=EDGE_CURVE('',#6853,#6858,#1669,.T.);
#8572=EDGE_CURVE('',#6859,#6837,#839,.T.);
#8573=EDGE_CURVE('',#6860,#6859,#5778,.T.);
#8574=EDGE_CURVE('',#6860,#6838,#5779,.T.);
#8575=EDGE_CURVE('',#6861,#6862,#5780,.T.);
#8576=EDGE_CURVE('',#6861,#6863,#840,.T.);
#8577=EDGE_CURVE('',#6864,#6863,#5781,.T.);
#8578=EDGE_CURVE('',#6864,#6862,#841,.T.);
#8579=EDGE_CURVE('',#6865,#6866,#5782,.T.);
#8580=EDGE_CURVE('',#6867,#6865,#842,.T.);
#8581=EDGE_CURVE('',#6868,#6867,#5783,.T.);
#8582=EDGE_CURVE('',#6866,#6868,#843,.T.);
#8583=EDGE_CURVE('',#6729,#6730,#71,.T.);
#8584=EDGE_CURVE('',#6727,#6733,#72,.T.);
#8585=EDGE_CURVE('',#6745,#6869,#5784,.T.);
#8586=EDGE_CURVE('',#6870,#6869,#844,.T.);
#8587=EDGE_CURVE('',#6747,#6870,#5785,.T.);
#8588=EDGE_CURVE('',#6740,#6871,#5786,.T.);
#8589=EDGE_CURVE('',#6872,#6871,#845,.T.);
#8590=EDGE_CURVE('',#6738,#6872,#5787,.T.);
#8591=EDGE_CURVE('',#6748,#6742,#1670,.T.);
#8592=EDGE_CURVE('',#6743,#6749,#1671,.T.);
#8593=EDGE_CURVE('',#6869,#6870,#846,.T.);
#8594=EDGE_CURVE('',#6871,#6872,#847,.T.);
#8595=EDGE_CURVE('',#6791,#6863,#1672,.T.);
#8596=EDGE_CURVE('',#6864,#6790,#1673,.T.);
#8597=EDGE_CURVE('',#6824,#6873,#1674,.T.);
#8598=EDGE_CURVE('',#6873,#6874,#1675,.T.);
#8599=EDGE_CURVE('',#6874,#6809,#1676,.T.);
#8600=EDGE_CURVE('',#6790,#6784,#1677,.T.);
#8601=EDGE_CURVE('',#6866,#6784,#1678,.T.);
#8602=EDGE_CURVE('',#6866,#6864,#1679,.T.);
#8603=EDGE_CURVE('',#6865,#6785,#1680,.T.);
#8604=EDGE_CURVE('',#6785,#6791,#1681,.T.);
#8605=EDGE_CURVE('',#6863,#6865,#1682,.T.);
#8606=EDGE_CURVE('',#6875,#6876,#1683,.T.);
#8607=EDGE_CURVE('',#6876,#6877,#1684,.T.);
#8608=EDGE_CURVE('',#6878,#6877,#1685,.T.);
#8609=EDGE_CURVE('',#6878,#6875,#1686,.T.);
#8610=EDGE_CURVE('',#6879,#6880,#1687,.T.);
#8611=EDGE_CURVE('',#6880,#6881,#1688,.T.);
#8612=EDGE_CURVE('',#6882,#6881,#1689,.T.);
#8613=EDGE_CURVE('',#6882,#6879,#1690,.T.);
#8614=EDGE_CURVE('',#6883,#6884,#1691,.T.);
#8615=EDGE_CURVE('',#6884,#6885,#1692,.T.);
#8616=EDGE_CURVE('',#6885,#6886,#1693,.T.);
#8617=EDGE_CURVE('',#6886,#6883,#1694,.T.);
#8618=EDGE_CURVE('',#6829,#6775,#1695,.T.);
#8619=EDGE_CURVE('',#6862,#6868,#1696,.T.);
#8620=EDGE_CURVE('',#6867,#6861,#1697,.T.);
#8621=EDGE_CURVE('',#6887,#6883,#848,.T.);
#8622=EDGE_CURVE('',#6888,#6887,#5788,.T.);
#8623=EDGE_CURVE('',#6878,#6888,#849,.T.);
#8624=EDGE_CURVE('',#6883,#6878,#5789,.T.);
#8625=EDGE_CURVE('',#6889,#6888,#1698,.T.);
#8626=EDGE_CURVE('',#6875,#6889,#850,.T.);
#8627=EDGE_CURVE('',#6890,#6886,#851,.T.);
#8628=EDGE_CURVE('',#6887,#6890,#1699,.T.);
#8629=EDGE_CURVE('',#6786,#6788,#1700,.T.);
#8630=EDGE_CURVE('',#6789,#6787,#1701,.T.);
#8631=EDGE_CURVE('',#6891,#6880,#852,.T.);
#8632=EDGE_CURVE('',#6892,#6880,#5790,.T.);
#8633=EDGE_CURVE('',#6893,#6892,#853,.T.);
#8634=EDGE_CURVE('',#6891,#6893,#5791,.T.);
#8635=EDGE_CURVE('',#6894,#6895,#5792,.T.);
#8636=EDGE_CURVE('',#6896,#6895,#5793,.T.);
#8637=EDGE_CURVE('',#6897,#6896,#5794,.T.);
#8638=EDGE_CURVE('',#6894,#6897,#5795,.T.);
#8639=EDGE_CURVE('',#6895,#6780,#1702,.T.);
#8640=EDGE_CURVE('',#6781,#6894,#1703,.T.);
#8641=EDGE_CURVE('',#6898,#6899,#5796,.T.);
#8642=EDGE_CURVE('',#6899,#6900,#1704,.T.);
#8643=EDGE_CURVE('',#6900,#6901,#1705,.T.);
#8644=EDGE_CURVE('',#6901,#6898,#1706,.T.);
#8645=EDGE_CURVE('',#6902,#6903,#854,.T.);
#8646=EDGE_CURVE('',#6902,#6904,#758,.T.);
#8647=EDGE_CURVE('',#6905,#6904,#5797,.T.);
#8648=EDGE_CURVE('',#6903,#6905,#759,.T.);
#8649=EDGE_CURVE('',#6906,#6904,#1707,.T.);
#8650=EDGE_CURVE('',#6907,#6906,#5798,.T.);
#8651=EDGE_CURVE('',#6905,#6907,#1708,.T.);
#8652=EDGE_CURVE('',#6907,#6799,#855,.T.);
#8653=EDGE_CURVE('',#6800,#6906,#760,.T.);
#8654=EDGE_CURVE('',#6904,#6908,#1709,.T.);
#8655=EDGE_CURVE('',#6801,#6908,#1710,.T.);
#8656=EDGE_CURVE('',#6909,#6902,#1711,.T.);
#8657=EDGE_CURVE('',#6903,#6757,#1712,.T.);
#8658=EDGE_CURVE('',#6910,#6757,#1713,.T.);
#8659=EDGE_CURVE('',#6910,#6815,#1714,.T.);
#8660=EDGE_CURVE('',#6815,#6909,#1715,.T.);
#8661=EDGE_CURVE('',#6772,#6827,#1716,.T.);
#8662=EDGE_CURVE('',#6851,#6911,#856,.T.);
#8663=EDGE_CURVE('',#6912,#6850,#857,.T.);
#8664=EDGE_CURVE('',#6911,#6912,#5799,.T.);
#8665=EDGE_CURVE('',#6847,#6913,#5800,.T.);
#8666=EDGE_CURVE('',#6913,#6914,#1717,.T.);
#8667=EDGE_CURVE('',#6914,#6846,#5801,.T.);
#8668=EDGE_CURVE('',#6848,#6845,#1718,.T.);
#8669=EDGE_CURVE('',#6858,#6837,#1719,.T.);
#8670=EDGE_CURVE('',#6851,#6854,#1720,.T.);
#8671=EDGE_CURVE('',#6842,#6915,#1721,.T.);
#8672=EDGE_CURVE('',#6915,#6843,#1722,.T.);
#8673=EDGE_CURVE('',#6841,#6916,#5802,.T.);
#8674=EDGE_CURVE('',#6917,#6916,#5803,.T.);
#8675=EDGE_CURVE('',#6842,#6917,#858,.T.);
#8676=EDGE_CURVE('',#6918,#6917,#1723,.T.);
#8677=EDGE_CURVE('',#6915,#6918,#5804,.T.);
#8678=EDGE_CURVE('',#6919,#6920,#859,.T.);
#8679=EDGE_CURVE('',#6921,#6919,#860,.T.);
#8680=EDGE_CURVE('',#6915,#6921,#761,.T.);
#8681=EDGE_CURVE('',#6920,#6918,#762,.T.);
#8682=EDGE_CURVE('',#6844,#6921,#1724,.T.);
#8683=EDGE_CURVE('',#6922,#6858,#5805,.T.);
#8684=EDGE_CURVE('',#6859,#6922,#1725,.T.);
#8685=EDGE_CURVE('',#6855,#6923,#861,.T.);
#8686=EDGE_CURVE('',#6922,#6923,#763,.T.);
#8687=EDGE_CURVE('',#6923,#6911,#1726,.T.);
#8688=EDGE_CURVE('',#6839,#6924,#862,.T.);
#8689=EDGE_CURVE('',#6924,#6860,#863,.T.);
#8690=EDGE_CURVE('',#6913,#6914,#5806,.T.);
#8691=EDGE_CURVE('',#6925,#6840,#864,.T.);
#8692=EDGE_CURVE('',#6916,#6925,#865,.T.);
#8693=EDGE_CURVE('',#6907,#6860,#5807,.T.);
#8694=EDGE_CURVE('',#6798,#6924,#5808,.T.);
#8695=EDGE_CURVE('',#6778,#6926,#866,.T.);
#8696=EDGE_CURVE('',#6916,#6926,#5809,.T.);
#8697=EDGE_CURVE('',#6796,#6925,#5810,.T.);
#8698=EDGE_CURVE('',#6775,#6927,#867,.T.);
#8699=EDGE_CURVE('',#6926,#6927,#5811,.T.);
#8700=EDGE_CURVE('',#6776,#6926,#5812,.T.);
#8701=EDGE_CURVE('',#6928,#6836,#1727,.T.);
#8702=EDGE_CURVE('',#6928,#6827,#764,.T.);
#8703=EDGE_CURVE('',#6929,#6762,#5813,.T.);
#8704=EDGE_CURVE('',#6929,#6930,#868,.T.);
#8705=EDGE_CURVE('',#6930,#6763,#5814,.T.);
#8706=EDGE_CURVE('',#6931,#6897,#1728,.T.);
#8707=EDGE_CURVE('',#6897,#6932,#5815,.T.);
#8708=EDGE_CURVE('',#6932,#6933,#1729,.T.);
#8709=EDGE_CURVE('',#6933,#6931,#5816,.T.);
#8710=EDGE_CURVE('',#6934,#6935,#1730,.T.);
#8711=EDGE_CURVE('',#6935,#6936,#1731,.T.);
#8712=EDGE_CURVE('',#6936,#6822,#869,.T.);
#8713=EDGE_CURVE('',#6821,#6934,#1732,.T.);
#8714=EDGE_CURVE('',#6937,#6896,#5817,.T.);
#8715=EDGE_CURVE('',#6932,#6937,#5818,.T.);
#8716=EDGE_CURVE('',#6932,#6935,#5819,.T.);
#8717=EDGE_CURVE('',#6933,#6934,#5820,.T.);
#8718=EDGE_CURVE('',#6938,#6939,#1733,.T.);
#8719=EDGE_CURVE('',#6938,#6794,#5821,.T.);
#8720=EDGE_CURVE('',#6939,#6793,#5822,.T.);
#8721=EDGE_CURVE('',#6894,#6940,#1734,.T.);
#8722=EDGE_CURVE('',#6940,#6931,#5823,.T.);
#8723=EDGE_CURVE('',#6768,#6941,#1735,.T.);
#8724=EDGE_CURVE('',#6941,#6825,#1736,.T.);
#8725=EDGE_CURVE('',#6941,#6767,#1737,.T.);
#8726=EDGE_CURVE('',#6942,#6943,#1738,.T.);
#8727=EDGE_CURVE('',#6943,#6816,#1739,.T.);
#8728=EDGE_CURVE('',#6816,#6944,#1740,.T.);
#8729=EDGE_CURVE('',#6944,#6942,#1741,.T.);
#8730=EDGE_CURVE('',#6945,#6946,#1742,.T.);
#8731=EDGE_CURVE('',#6946,#6947,#1743,.T.);
#8732=EDGE_CURVE('',#6948,#6947,#870,.T.);
#8733=EDGE_CURVE('',#6930,#6948,#1744,.T.);
#8734=EDGE_CURVE('',#6949,#6929,#1745,.T.);
#8735=EDGE_CURVE('',#6949,#6950,#1746,.T.);
#8736=EDGE_CURVE('',#6950,#6945,#1747,.T.);
#8737=EDGE_CURVE('',#6829,#6951,#765,.T.);
#8738=EDGE_CURVE('',#6927,#6951,#1748,.T.);
#8739=EDGE_CURVE('',#6952,#6928,#871,.T.);
#8740=EDGE_CURVE('',#6828,#6952,#766,.T.);
#8741=EDGE_CURVE('',#6951,#6953,#872,.T.);
#8742=EDGE_CURVE('',#6953,#6828,#767,.T.);
#8743=EDGE_CURVE('',#6824,#6954,#873,.T.);
#8744=EDGE_CURVE('',#6955,#6954,#1749,.T.);
#8745=EDGE_CURVE('',#6955,#6873,#874,.T.);
#8746=EDGE_CURVE('',#6956,#6937,#5824,.T.);
#8747=EDGE_CURVE('',#6956,#6935,#5825,.T.);
#8748=EDGE_CURVE('',#6957,#6823,#5826,.T.);
#8749=EDGE_CURVE('',#6954,#6957,#5827,.T.);
#8750=EDGE_CURVE('',#6957,#6936,#875,.T.);
#8751=EDGE_CURVE('',#6957,#6956,#1750,.T.);
#8752=EDGE_CURVE('',#6831,#6958,#5828,.T.);
#8753=EDGE_CURVE('',#6958,#6938,#876,.T.);
#8754=EDGE_CURVE('',#6939,#6830,#5829,.T.);
#8755=EDGE_CURVE('',#6811,#6958,#5830,.T.);
#8756=EDGE_CURVE('',#6833,#6811,#5831,.T.);
#8757=EDGE_CURVE('',#6792,#6949,#5832,.T.);
#8758=EDGE_CURVE('',#6826,#6941,#1751,.T.);
#8759=EDGE_CURVE('',#6810,#6959,#1752,.T.);
#8760=EDGE_CURVE('',#6959,#6960,#5833,.T.);
#8761=EDGE_CURVE('',#6960,#6832,#1753,.T.);
#8762=EDGE_CURVE('',#6961,#6962,#1754,.T.);
#8763=EDGE_CURVE('',#6963,#6962,#5834,.T.);
#8764=EDGE_CURVE('',#6963,#6964,#1755,.T.);
#8765=EDGE_CURVE('',#6964,#6961,#5835,.T.);
#8766=EDGE_CURVE('',#6890,#6889,#5836,.T.);
#8767=EDGE_CURVE('',#6901,#6942,#5837,.T.);
#8768=EDGE_CURVE('',#6944,#6910,#5838,.T.);
#8769=EDGE_CURVE('',#6757,#6805,#1756,.T.);
#8770=EDGE_CURVE('',#6804,#6898,#877,.T.);
#8771=EDGE_CURVE('',#6877,#6884,#5839,.T.);
#8772=EDGE_CURVE('',#6881,#6965,#5840,.T.);
#8773=EDGE_CURVE('',#6966,#6965,#1757,.T.);
#8774=EDGE_CURVE('',#6966,#6882,#5841,.T.);
#8775=EDGE_CURVE('',#6766,#6820,#1758,.T.);
#8776=EDGE_CURVE('',#6967,#6765,#5842,.T.);
#8777=EDGE_CURVE('',#6967,#6968,#1759,.T.);
#8778=EDGE_CURVE('',#6968,#6955,#5843,.T.);
#8779=EDGE_CURVE('',#6969,#6970,#1760,.T.);
#8780=EDGE_CURVE('',#6970,#6971,#5844,.T.);
#8781=EDGE_CURVE('',#6971,#6972,#1761,.T.);
#8782=EDGE_CURVE('',#6972,#6969,#5845,.T.);
#8783=EDGE_CURVE('',#6893,#6973,#1762,.T.);
#8784=EDGE_CURVE('',#6973,#6974,#5846,.T.);
#8785=EDGE_CURVE('',#6974,#6891,#1763,.T.);
#8786=EDGE_CURVE('',#6965,#6892,#1764,.T.);
#8787=EDGE_CURVE('',#6892,#6975,#1765,.T.);
#8788=EDGE_CURVE('',#6975,#6966,#1766,.T.);
#8789=EDGE_CURVE('',#6873,#6946,#5847,.T.);
#8790=EDGE_CURVE('',#6945,#6874,#5848,.T.);
#8791=EDGE_CURVE('',#6885,#6876,#5849,.T.);
#8792=EDGE_CURVE('',#6875,#6886,#5850,.T.);
#8793=EDGE_CURVE('',#6879,#6963,#878,.T.);
#8794=EDGE_CURVE('',#6962,#6975,#879,.T.);
#8795=EDGE_CURVE('',#6964,#6882,#880,.T.);
#8796=EDGE_CURVE('',#6961,#6966,#881,.T.);
#8797=EDGE_CURVE('',#6874,#6959,#882,.T.);
#8798=EDGE_CURVE('',#6945,#6960,#883,.T.);
#8799=EDGE_CURVE('',#6834,#6950,#884,.T.);
#8800=EDGE_CURVE('',#6953,#6952,#1767,.T.);
#8801=EDGE_CURVE('',#6900,#6976,#885,.T.);
#8802=EDGE_CURVE('',#6976,#6943,#886,.T.);
#8803=EDGE_CURVE('',#6908,#6813,#1768,.T.);
#8804=EDGE_CURVE('',#6908,#6909,#768,.T.);
#8805=EDGE_CURVE('',#6803,#6899,#887,.T.);
#8806=EDGE_CURVE('',#6814,#6977,#1769,.T.);
#8807=EDGE_CURVE('',#6977,#6978,#1770,.T.);
#8808=EDGE_CURVE('',#6978,#6802,#5851,.T.);
#8809=EDGE_CURVE('',#6977,#6976,#769,.T.);
#8810=EDGE_CURVE('',#6978,#6899,#5852,.T.);
#8811=EDGE_CURVE('',#6940,#6835,#1771,.T.);
#8812=EDGE_CURVE('',#6912,#6920,#1772,.T.);
#8813=EDGE_CURVE('',#6884,#6972,#888,.T.);
#8814=EDGE_CURVE('',#6885,#6971,#889,.T.);
#8815=EDGE_CURVE('',#6969,#6877,#890,.T.);
#8816=EDGE_CURVE('',#6970,#6876,#891,.T.);
#8817=EDGE_CURVE('',#6973,#6965,#892,.T.);
#8818=EDGE_CURVE('',#6881,#6974,#893,.T.);
#8819=EDGE_CURVE('',#6968,#6946,#894,.T.);
#8820=EDGE_CURVE('',#6947,#6967,#895,.T.);
#8821=EDGE_CURVE('',#6948,#6764,#5853,.T.);
#8822=EDGE_CURVE('',#6979,#6849,#1773,.T.);
#8823=EDGE_CURVE('',#6919,#6979,#1774,.T.);
#8824=EDGE_CURVE('',#6844,#6979,#1775,.T.);
#11411=ORIENTED_EDGE('',*,*,#8412,.T.);
#11412=ORIENTED_EDGE('',*,*,#8413,.T.);
#11413=ORIENTED_EDGE('',*,*,#8414,.T.);
#11414=ORIENTED_EDGE('',*,*,#8415,.T.);
#11415=ORIENTED_EDGE('',*,*,#8416,.T.);
#11416=ORIENTED_EDGE('',*,*,#8417,.T.);
#11417=ORIENTED_EDGE('',*,*,#8418,.T.);
#11418=ORIENTED_EDGE('',*,*,#8414,.F.);
#11419=ORIENTED_EDGE('',*,*,#8419,.F.);
#11420=ORIENTED_EDGE('',*,*,#8420,.F.);
#11421=ORIENTED_EDGE('',*,*,#8421,.F.);
#11422=ORIENTED_EDGE('',*,*,#8422,.F.);
#11423=ORIENTED_EDGE('',*,*,#8423,.T.);
#11424=ORIENTED_EDGE('',*,*,#8424,.F.);
#11425=ORIENTED_EDGE('',*,*,#8425,.F.);
#11426=ORIENTED_EDGE('',*,*,#8423,.F.);
#11427=ORIENTED_EDGE('',*,*,#8426,.F.);
#11428=ORIENTED_EDGE('',*,*,#8427,.T.);
#11429=ORIENTED_EDGE('',*,*,#8428,.T.);
#11430=ORIENTED_EDGE('',*,*,#8429,.T.);
#11431=ORIENTED_EDGE('',*,*,#8430,.T.);
#11432=ORIENTED_EDGE('',*,*,#8431,.F.);
#11433=ORIENTED_EDGE('',*,*,#8432,.T.);
#11434=ORIENTED_EDGE('',*,*,#8433,.F.);
#11435=ORIENTED_EDGE('',*,*,#8432,.F.);
#11436=ORIENTED_EDGE('',*,*,#8434,.T.);
#11437=ORIENTED_EDGE('',*,*,#8435,.T.);
#11438=ORIENTED_EDGE('',*,*,#8436,.T.);
#11439=ORIENTED_EDGE('',*,*,#8437,.T.);
#11440=ORIENTED_EDGE('',*,*,#8438,.T.);
#11441=ORIENTED_EDGE('',*,*,#8439,.T.);
#11442=ORIENTED_EDGE('',*,*,#8435,.F.);
#11443=ORIENTED_EDGE('',*,*,#8440,.T.);
#11444=ORIENTED_EDGE('',*,*,#8441,.T.);
#11445=ORIENTED_EDGE('',*,*,#8412,.F.);
#11446=ORIENTED_EDGE('',*,*,#8413,.F.);
#11447=ORIENTED_EDGE('',*,*,#8441,.F.);
#11448=ORIENTED_EDGE('',*,*,#8425,.T.);
#11449=ORIENTED_EDGE('',*,*,#8442,.T.);
#11450=ORIENTED_EDGE('',*,*,#8443,.F.);
#11451=ORIENTED_EDGE('',*,*,#8442,.F.);
#11452=ORIENTED_EDGE('',*,*,#8424,.T.);
#11453=ORIENTED_EDGE('',*,*,#8444,.F.);
#11454=ORIENTED_EDGE('',*,*,#8445,.T.);
#11455=ORIENTED_EDGE('',*,*,#8446,.T.);
#11456=ORIENTED_EDGE('',*,*,#8445,.F.);
#11457=ORIENTED_EDGE('',*,*,#8447,.F.);
#11458=ORIENTED_EDGE('',*,*,#8448,.F.);
#11459=ORIENTED_EDGE('',*,*,#8449,.T.);
#11460=ORIENTED_EDGE('',*,*,#8450,.F.);
#11461=ORIENTED_EDGE('',*,*,#8449,.F.);
#11462=ORIENTED_EDGE('',*,*,#8451,.T.);
#11463=ORIENTED_EDGE('',*,*,#8452,.T.);
#11464=ORIENTED_EDGE('',*,*,#8453,.T.);
#11465=ORIENTED_EDGE('',*,*,#8447,.T.);
#11466=ORIENTED_EDGE('',*,*,#8448,.T.);
#11467=ORIENTED_EDGE('',*,*,#8453,.F.);
#11468=ORIENTED_EDGE('',*,*,#8454,.T.);
#11469=ORIENTED_EDGE('',*,*,#8455,.T.);
#11470=ORIENTED_EDGE('',*,*,#8456,.T.);
#11471=ORIENTED_EDGE('',*,*,#8457,.F.);
#11472=ORIENTED_EDGE('',*,*,#8458,.T.);
#11473=ORIENTED_EDGE('',*,*,#8459,.T.);
#11474=ORIENTED_EDGE('',*,*,#8460,.T.);
#11475=ORIENTED_EDGE('',*,*,#8461,.T.);
#11476=ORIENTED_EDGE('',*,*,#8462,.T.);
#11477=ORIENTED_EDGE('',*,*,#8463,.F.);
#11478=ORIENTED_EDGE('',*,*,#8464,.T.);
#11479=ORIENTED_EDGE('',*,*,#8465,.T.);
#11480=ORIENTED_EDGE('',*,*,#8466,.T.);
#11481=ORIENTED_EDGE('',*,*,#8455,.F.);
#11482=ORIENTED_EDGE('',*,*,#8467,.T.);
#11483=ORIENTED_EDGE('',*,*,#8468,.T.);
#11484=ORIENTED_EDGE('',*,*,#8469,.T.);
#11485=ORIENTED_EDGE('',*,*,#8470,.T.);
#11486=ORIENTED_EDGE('',*,*,#8471,.T.);
#11487=ORIENTED_EDGE('',*,*,#8472,.T.);
#11488=ORIENTED_EDGE('',*,*,#8473,.T.);
#11489=ORIENTED_EDGE('',*,*,#8474,.T.);
#11490=ORIENTED_EDGE('',*,*,#8475,.T.);
#11491=ORIENTED_EDGE('',*,*,#8476,.T.);
#11492=ORIENTED_EDGE('',*,*,#8477,.T.);
#11493=ORIENTED_EDGE('',*,*,#8478,.F.);
#11494=ORIENTED_EDGE('',*,*,#8479,.T.);
#11495=ORIENTED_EDGE('',*,*,#8480,.F.);
#11496=ORIENTED_EDGE('',*,*,#8481,.T.);
#11497=ORIENTED_EDGE('',*,*,#8469,.F.);
#11498=ORIENTED_EDGE('',*,*,#8426,.T.);
#11499=ORIENTED_EDGE('',*,*,#8431,.T.);
#11500=ORIENTED_EDGE('',*,*,#8482,.T.);
#11501=ORIENTED_EDGE('',*,*,#8483,.F.);
#11502=ORIENTED_EDGE('',*,*,#8484,.T.);
#11503=ORIENTED_EDGE('',*,*,#8451,.F.);
#11504=ORIENTED_EDGE('',*,*,#8452,.F.);
#11505=ORIENTED_EDGE('',*,*,#8484,.F.);
#11506=ORIENTED_EDGE('',*,*,#8485,.F.);
#11507=ORIENTED_EDGE('',*,*,#8486,.T.);
#11508=ORIENTED_EDGE('',*,*,#8487,.F.);
#11509=ORIENTED_EDGE('',*,*,#8488,.T.);
#11510=ORIENTED_EDGE('',*,*,#8489,.F.);
#11511=ORIENTED_EDGE('',*,*,#8490,.F.);
#11512=ORIENTED_EDGE('',*,*,#8491,.F.);
#11513=ORIENTED_EDGE('',*,*,#8492,.F.);
#11514=ORIENTED_EDGE('',*,*,#8493,.T.);
#11515=ORIENTED_EDGE('',*,*,#8494,.T.);
#11516=ORIENTED_EDGE('',*,*,#8495,.T.);
#11517=ORIENTED_EDGE('',*,*,#8496,.T.);
#11518=ORIENTED_EDGE('',*,*,#8497,.T.);
#11519=ORIENTED_EDGE('',*,*,#8498,.T.);
#11520=ORIENTED_EDGE('',*,*,#8499,.T.);
#11521=ORIENTED_EDGE('',*,*,#8500,.T.);
#11522=ORIENTED_EDGE('',*,*,#8501,.T.);
#11523=ORIENTED_EDGE('',*,*,#8502,.T.);
#11524=ORIENTED_EDGE('',*,*,#8503,.T.);
#11525=ORIENTED_EDGE('',*,*,#8504,.T.);
#11526=ORIENTED_EDGE('',*,*,#8505,.T.);
#11527=ORIENTED_EDGE('',*,*,#8506,.T.);
#11528=ORIENTED_EDGE('',*,*,#8507,.F.);
#11529=ORIENTED_EDGE('',*,*,#8508,.T.);
#11530=ORIENTED_EDGE('',*,*,#8509,.F.);
#11531=ORIENTED_EDGE('',*,*,#8477,.F.);
#11532=ORIENTED_EDGE('',*,*,#8466,.F.);
#11533=ORIENTED_EDGE('',*,*,#8510,.F.);
#11534=ORIENTED_EDGE('',*,*,#8511,.F.);
#11535=ORIENTED_EDGE('',*,*,#8512,.F.);
#11536=ORIENTED_EDGE('',*,*,#8513,.F.);
#11537=ORIENTED_EDGE('',*,*,#8514,.F.);
#11538=ORIENTED_EDGE('',*,*,#8515,.F.);
#11539=ORIENTED_EDGE('',*,*,#8456,.F.);
#11540=ORIENTED_EDGE('',*,*,#8516,.F.);
#11541=ORIENTED_EDGE('',*,*,#8517,.F.);
#11542=ORIENTED_EDGE('',*,*,#8518,.F.);
#11543=ORIENTED_EDGE('',*,*,#8519,.T.);
#11544=ORIENTED_EDGE('',*,*,#8468,.F.);
#11545=ORIENTED_EDGE('',*,*,#8520,.T.);
#11546=ORIENTED_EDGE('',*,*,#8521,.F.);
#11547=ORIENTED_EDGE('',*,*,#8520,.F.);
#11548=ORIENTED_EDGE('',*,*,#8522,.F.);
#11549=ORIENTED_EDGE('',*,*,#8523,.T.);
#11550=ORIENTED_EDGE('',*,*,#8524,.T.);
#11551=ORIENTED_EDGE('',*,*,#8523,.F.);
#11552=ORIENTED_EDGE('',*,*,#8525,.T.);
#11553=ORIENTED_EDGE('',*,*,#8508,.F.);
#11554=ORIENTED_EDGE('',*,*,#8526,.F.);
#11555=ORIENTED_EDGE('',*,*,#8527,.T.);
#11556=ORIENTED_EDGE('',*,*,#8528,.T.);
#11557=ORIENTED_EDGE('',*,*,#8529,.T.);
#11558=ORIENTED_EDGE('',*,*,#8530,.T.);
#11559=ORIENTED_EDGE('',*,*,#8511,.T.);
#11560=ORIENTED_EDGE('',*,*,#8531,.F.);
#11561=ORIENTED_EDGE('',*,*,#8532,.T.);
#11562=ORIENTED_EDGE('',*,*,#8533,.F.);
#11563=ORIENTED_EDGE('',*,*,#8472,.F.);
#11564=ORIENTED_EDGE('',*,*,#8534,.F.);
#11565=ORIENTED_EDGE('',*,*,#8535,.F.);
#11566=ORIENTED_EDGE('',*,*,#8536,.F.);
#11567=ORIENTED_EDGE('',*,*,#8537,.F.);
#11568=ORIENTED_EDGE('',*,*,#8538,.F.);
#11569=ORIENTED_EDGE('',*,*,#8457,.T.);
#11570=ORIENTED_EDGE('',*,*,#8515,.T.);
#11571=ORIENTED_EDGE('',*,*,#8539,.F.);
#11572=ORIENTED_EDGE('',*,*,#8540,.F.);
#11573=ORIENTED_EDGE('',*,*,#8541,.F.);
#11574=ORIENTED_EDGE('',*,*,#8542,.T.);
#11575=ORIENTED_EDGE('',*,*,#8543,.F.);
#11576=ORIENTED_EDGE('',*,*,#8495,.F.);
#11577=ORIENTED_EDGE('',*,*,#8544,.F.);
#11578=ORIENTED_EDGE('',*,*,#8481,.F.);
#11579=ORIENTED_EDGE('',*,*,#8545,.F.);
#11580=ORIENTED_EDGE('',*,*,#8546,.F.);
#11581=ORIENTED_EDGE('',*,*,#8547,.F.);
#11582=ORIENTED_EDGE('',*,*,#8470,.F.);
#11583=ORIENTED_EDGE('',*,*,#8548,.T.);
#11584=ORIENTED_EDGE('',*,*,#8549,.T.);
#11585=ORIENTED_EDGE('',*,*,#8550,.F.);
#11586=ORIENTED_EDGE('',*,*,#8551,.F.);
#11587=ORIENTED_EDGE('',*,*,#8552,.T.);
#11588=ORIENTED_EDGE('',*,*,#8553,.T.);
#11589=ORIENTED_EDGE('',*,*,#8554,.F.);
#11590=ORIENTED_EDGE('',*,*,#8555,.T.);
#11591=ORIENTED_EDGE('',*,*,#8556,.F.);
#11592=ORIENTED_EDGE('',*,*,#8557,.F.);
#11593=ORIENTED_EDGE('',*,*,#8558,.T.);
#11594=ORIENTED_EDGE('',*,*,#8559,.F.);
#11595=ORIENTED_EDGE('',*,*,#8560,.F.);
#11596=ORIENTED_EDGE('',*,*,#8561,.T.);
#11597=ORIENTED_EDGE('',*,*,#8562,.T.);
#11598=ORIENTED_EDGE('',*,*,#8563,.T.);
#11599=ORIENTED_EDGE('',*,*,#8564,.T.);
#11600=ORIENTED_EDGE('',*,*,#8565,.F.);
#11601=ORIENTED_EDGE('',*,*,#8564,.F.);
#11602=ORIENTED_EDGE('',*,*,#8566,.F.);
#11603=ORIENTED_EDGE('',*,*,#8567,.F.);
#11604=ORIENTED_EDGE('',*,*,#8568,.F.);
#11605=ORIENTED_EDGE('',*,*,#8569,.T.);
#11606=ORIENTED_EDGE('',*,*,#8570,.T.);
#11607=ORIENTED_EDGE('',*,*,#8571,.F.);
#11608=ORIENTED_EDGE('',*,*,#8548,.F.);
#11609=ORIENTED_EDGE('',*,*,#8572,.F.);
#11610=ORIENTED_EDGE('',*,*,#8573,.F.);
#11611=ORIENTED_EDGE('',*,*,#8574,.T.);
#11612=ORIENTED_EDGE('',*,*,#8575,.F.);
#11613=ORIENTED_EDGE('',*,*,#8576,.T.);
#11614=ORIENTED_EDGE('',*,*,#8577,.F.);
#11615=ORIENTED_EDGE('',*,*,#8578,.T.);
#11616=ORIENTED_EDGE('',*,*,#8579,.F.);
#11617=ORIENTED_EDGE('',*,*,#8580,.F.);
#11618=ORIENTED_EDGE('',*,*,#8581,.F.);
#11619=ORIENTED_EDGE('',*,*,#8582,.F.);
#11620=ORIENTED_EDGE('',*,*,#8418,.F.);
#11621=ORIENTED_EDGE('',*,*,#8583,.T.);
#11622=ORIENTED_EDGE('',*,*,#8419,.T.);
#11623=ORIENTED_EDGE('',*,*,#8422,.T.);
#11624=ORIENTED_EDGE('',*,*,#8584,.F.);
#11625=ORIENTED_EDGE('',*,*,#8415,.F.);
#11626=ORIENTED_EDGE('',*,*,#8437,.F.);
#11627=ORIENTED_EDGE('',*,*,#8585,.T.);
#11628=ORIENTED_EDGE('',*,*,#8586,.F.);
#11629=ORIENTED_EDGE('',*,*,#8587,.F.);
#11630=ORIENTED_EDGE('',*,*,#8438,.F.);
#11631=ORIENTED_EDGE('',*,*,#8430,.F.);
#11632=ORIENTED_EDGE('',*,*,#8588,.T.);
#11633=ORIENTED_EDGE('',*,*,#8589,.F.);
#11634=ORIENTED_EDGE('',*,*,#8590,.F.);
#11635=ORIENTED_EDGE('',*,*,#8427,.F.);
#11636=ORIENTED_EDGE('',*,*,#8482,.F.);
#11637=ORIENTED_EDGE('',*,*,#8440,.F.);
#11638=ORIENTED_EDGE('',*,*,#8591,.T.);
#11639=ORIENTED_EDGE('',*,*,#8433,.T.);
#11640=ORIENTED_EDGE('',*,*,#8591,.F.);
#11641=ORIENTED_EDGE('',*,*,#8434,.F.);
#11642=ORIENTED_EDGE('',*,*,#8592,.T.);
#11643=ORIENTED_EDGE('',*,*,#8443,.T.);
#11644=ORIENTED_EDGE('',*,*,#8592,.F.);
#11645=ORIENTED_EDGE('',*,*,#8586,.T.);
#11646=ORIENTED_EDGE('',*,*,#8593,.T.);
#11647=ORIENTED_EDGE('',*,*,#8588,.F.);
#11648=ORIENTED_EDGE('',*,*,#8429,.F.);
#11649=ORIENTED_EDGE('',*,*,#8428,.F.);
#11650=ORIENTED_EDGE('',*,*,#8590,.T.);
#11651=ORIENTED_EDGE('',*,*,#8594,.F.);
#11652=ORIENTED_EDGE('',*,*,#8585,.F.);
#11653=ORIENTED_EDGE('',*,*,#8436,.F.);
#11654=ORIENTED_EDGE('',*,*,#8439,.F.);
#11655=ORIENTED_EDGE('',*,*,#8587,.T.);
#11656=ORIENTED_EDGE('',*,*,#8593,.F.);
#11657=ORIENTED_EDGE('',*,*,#8589,.T.);
#11658=ORIENTED_EDGE('',*,*,#8594,.T.);
#11659=ORIENTED_EDGE('',*,*,#8583,.F.);
#11660=ORIENTED_EDGE('',*,*,#8417,.F.);
#11661=ORIENTED_EDGE('',*,*,#8416,.F.);
#11662=ORIENTED_EDGE('',*,*,#8584,.T.);
#11663=ORIENTED_EDGE('',*,*,#8421,.T.);
#11664=ORIENTED_EDGE('',*,*,#8420,.T.);
#11665=ORIENTED_EDGE('',*,*,#8595,.F.);
#11666=ORIENTED_EDGE('',*,*,#8491,.T.);
#11667=ORIENTED_EDGE('',*,*,#8596,.F.);
#11668=ORIENTED_EDGE('',*,*,#8577,.T.);
#11669=ORIENTED_EDGE('',*,*,#8530,.F.);
#11670=ORIENTED_EDGE('',*,*,#8597,.T.);
#11671=ORIENTED_EDGE('',*,*,#8598,.T.);
#11672=ORIENTED_EDGE('',*,*,#8599,.T.);
#11673=ORIENTED_EDGE('',*,*,#8596,.T.);
#11674=ORIENTED_EDGE('',*,*,#8600,.T.);
#11675=ORIENTED_EDGE('',*,*,#8601,.F.);
#11676=ORIENTED_EDGE('',*,*,#8602,.T.);
#11677=ORIENTED_EDGE('',*,*,#8603,.T.);
#11678=ORIENTED_EDGE('',*,*,#8604,.T.);
#11679=ORIENTED_EDGE('',*,*,#8595,.T.);
#11680=ORIENTED_EDGE('',*,*,#8605,.T.);
#11681=ORIENTED_EDGE('',*,*,#8606,.T.);
#11682=ORIENTED_EDGE('',*,*,#8607,.T.);
#11683=ORIENTED_EDGE('',*,*,#8608,.F.);
#11684=ORIENTED_EDGE('',*,*,#8609,.T.);
#11685=ORIENTED_EDGE('',*,*,#8610,.T.);
#11686=ORIENTED_EDGE('',*,*,#8611,.T.);
#11687=ORIENTED_EDGE('',*,*,#8612,.F.);
#11688=ORIENTED_EDGE('',*,*,#8613,.T.);
#11689=ORIENTED_EDGE('',*,*,#8614,.T.);
#11690=ORIENTED_EDGE('',*,*,#8615,.T.);
#11691=ORIENTED_EDGE('',*,*,#8616,.T.);
#11692=ORIENTED_EDGE('',*,*,#8617,.T.);
#11693=ORIENTED_EDGE('',*,*,#8473,.F.);
#11694=ORIENTED_EDGE('',*,*,#8537,.T.);
#11695=ORIENTED_EDGE('',*,*,#8618,.T.);
#11696=ORIENTED_EDGE('',*,*,#8582,.T.);
#11697=ORIENTED_EDGE('',*,*,#8619,.F.);
#11698=ORIENTED_EDGE('',*,*,#8578,.F.);
#11699=ORIENTED_EDGE('',*,*,#8602,.F.);
#11700=ORIENTED_EDGE('',*,*,#8580,.T.);
#11701=ORIENTED_EDGE('',*,*,#8605,.F.);
#11702=ORIENTED_EDGE('',*,*,#8576,.F.);
#11703=ORIENTED_EDGE('',*,*,#8620,.F.);
#11704=ORIENTED_EDGE('',*,*,#8621,.F.);
#11705=ORIENTED_EDGE('',*,*,#8622,.F.);
#11706=ORIENTED_EDGE('',*,*,#8623,.F.);
#11707=ORIENTED_EDGE('',*,*,#8624,.F.);
#11708=ORIENTED_EDGE('',*,*,#8623,.T.);
#11709=ORIENTED_EDGE('',*,*,#8625,.F.);
#11710=ORIENTED_EDGE('',*,*,#8626,.F.);
#11711=ORIENTED_EDGE('',*,*,#8609,.F.);
#11712=ORIENTED_EDGE('',*,*,#8621,.T.);
#11713=ORIENTED_EDGE('',*,*,#8617,.F.);
#11714=ORIENTED_EDGE('',*,*,#8627,.F.);
#11715=ORIENTED_EDGE('',*,*,#8628,.F.);
#11716=ORIENTED_EDGE('',*,*,#8490,.T.);
#11717=ORIENTED_EDGE('',*,*,#8629,.F.);
#11718=ORIENTED_EDGE('',*,*,#8486,.F.);
#11719=ORIENTED_EDGE('',*,*,#8600,.F.);
#11720=ORIENTED_EDGE('',*,*,#8492,.T.);
#11721=ORIENTED_EDGE('',*,*,#8604,.F.);
#11722=ORIENTED_EDGE('',*,*,#8488,.F.);
#11723=ORIENTED_EDGE('',*,*,#8630,.F.);
#11724=ORIENTED_EDGE('',*,*,#8631,.T.);
#11725=ORIENTED_EDGE('',*,*,#8632,.F.);
#11726=ORIENTED_EDGE('',*,*,#8633,.F.);
#11727=ORIENTED_EDGE('',*,*,#8634,.F.);
#11728=ORIENTED_EDGE('',*,*,#8635,.T.);
#11729=ORIENTED_EDGE('',*,*,#8636,.F.);
#11730=ORIENTED_EDGE('',*,*,#8637,.F.);
#11731=ORIENTED_EDGE('',*,*,#8638,.F.);
#11732=ORIENTED_EDGE('',*,*,#8479,.F.);
#11733=ORIENTED_EDGE('',*,*,#8639,.F.);
#11734=ORIENTED_EDGE('',*,*,#8635,.F.);
#11735=ORIENTED_EDGE('',*,*,#8640,.F.);
#11736=ORIENTED_EDGE('',*,*,#8641,.T.);
#11737=ORIENTED_EDGE('',*,*,#8642,.T.);
#11738=ORIENTED_EDGE('',*,*,#8643,.T.);
#11739=ORIENTED_EDGE('',*,*,#8644,.T.);
#11740=ORIENTED_EDGE('',*,*,#8645,.F.);
#11741=ORIENTED_EDGE('',*,*,#8646,.T.);
#11742=ORIENTED_EDGE('',*,*,#8647,.F.);
#11743=ORIENTED_EDGE('',*,*,#8648,.F.);
#11744=ORIENTED_EDGE('',*,*,#8647,.T.);
#11745=ORIENTED_EDGE('',*,*,#8649,.F.);
#11746=ORIENTED_EDGE('',*,*,#8650,.F.);
#11747=ORIENTED_EDGE('',*,*,#8651,.F.);
#11748=ORIENTED_EDGE('',*,*,#8501,.F.);
#11749=ORIENTED_EDGE('',*,*,#8652,.F.);
#11750=ORIENTED_EDGE('',*,*,#8650,.T.);
#11751=ORIENTED_EDGE('',*,*,#8653,.F.);
#11752=ORIENTED_EDGE('',*,*,#8502,.F.);
#11753=ORIENTED_EDGE('',*,*,#8653,.T.);
#11754=ORIENTED_EDGE('',*,*,#8649,.T.);
#11755=ORIENTED_EDGE('',*,*,#8654,.T.);
#11756=ORIENTED_EDGE('',*,*,#8655,.F.);
#11757=ORIENTED_EDGE('',*,*,#8656,.T.);
#11758=ORIENTED_EDGE('',*,*,#8645,.T.);
#11759=ORIENTED_EDGE('',*,*,#8657,.T.);
#11760=ORIENTED_EDGE('',*,*,#8658,.F.);
#11761=ORIENTED_EDGE('',*,*,#8659,.T.);
#11762=ORIENTED_EDGE('',*,*,#8660,.T.);
#11763=ORIENTED_EDGE('',*,*,#8661,.T.);
#11764=ORIENTED_EDGE('',*,*,#8534,.T.);
#11765=ORIENTED_EDGE('',*,*,#8471,.F.);
#11766=ORIENTED_EDGE('',*,*,#8662,.F.);
#11767=ORIENTED_EDGE('',*,*,#8562,.F.);
#11768=ORIENTED_EDGE('',*,*,#8663,.F.);
#11769=ORIENTED_EDGE('',*,*,#8664,.F.);
#11770=ORIENTED_EDGE('',*,*,#8559,.T.);
#11771=ORIENTED_EDGE('',*,*,#8665,.T.);
#11772=ORIENTED_EDGE('',*,*,#8666,.T.);
#11773=ORIENTED_EDGE('',*,*,#8667,.T.);
#11774=ORIENTED_EDGE('',*,*,#8557,.T.);
#11775=ORIENTED_EDGE('',*,*,#8668,.F.);
#11776=ORIENTED_EDGE('',*,*,#8565,.T.);
#11777=ORIENTED_EDGE('',*,*,#8571,.T.);
#11778=ORIENTED_EDGE('',*,*,#8669,.T.);
#11779=ORIENTED_EDGE('',*,*,#8563,.F.);
#11780=ORIENTED_EDGE('',*,*,#8670,.T.);
#11781=ORIENTED_EDGE('',*,*,#8566,.T.);
#11782=ORIENTED_EDGE('',*,*,#8671,.T.);
#11783=ORIENTED_EDGE('',*,*,#8672,.T.);
#11784=ORIENTED_EDGE('',*,*,#8554,.T.);
#11785=ORIENTED_EDGE('',*,*,#8673,.T.);
#11786=ORIENTED_EDGE('',*,*,#8674,.F.);
#11787=ORIENTED_EDGE('',*,*,#8675,.F.);
#11788=ORIENTED_EDGE('',*,*,#8553,.F.);
#11789=ORIENTED_EDGE('',*,*,#8675,.T.);
#11790=ORIENTED_EDGE('',*,*,#8676,.F.);
#11791=ORIENTED_EDGE('',*,*,#8677,.F.);
#11792=ORIENTED_EDGE('',*,*,#8671,.F.);
#11793=ORIENTED_EDGE('',*,*,#8678,.F.);
#11794=ORIENTED_EDGE('',*,*,#8679,.F.);
#11795=ORIENTED_EDGE('',*,*,#8680,.F.);
#11796=ORIENTED_EDGE('',*,*,#8677,.T.);
#11797=ORIENTED_EDGE('',*,*,#8681,.F.);
#11798=ORIENTED_EDGE('',*,*,#8680,.T.);
#11799=ORIENTED_EDGE('',*,*,#8682,.F.);
#11800=ORIENTED_EDGE('',*,*,#8555,.F.);
#11801=ORIENTED_EDGE('',*,*,#8672,.F.);
#11802=ORIENTED_EDGE('',*,*,#8683,.F.);
#11803=ORIENTED_EDGE('',*,*,#8684,.F.);
#11804=ORIENTED_EDGE('',*,*,#8572,.T.);
#11805=ORIENTED_EDGE('',*,*,#8669,.F.);
#11806=ORIENTED_EDGE('',*,*,#8568,.T.);
#11807=ORIENTED_EDGE('',*,*,#8685,.T.);
#11808=ORIENTED_EDGE('',*,*,#8686,.F.);
#11809=ORIENTED_EDGE('',*,*,#8683,.T.);
#11810=ORIENTED_EDGE('',*,*,#8570,.F.);
#11811=ORIENTED_EDGE('',*,*,#8569,.F.);
#11812=ORIENTED_EDGE('',*,*,#8670,.F.);
#11813=ORIENTED_EDGE('',*,*,#8662,.T.);
#11814=ORIENTED_EDGE('',*,*,#8687,.F.);
#11815=ORIENTED_EDGE('',*,*,#8685,.F.);
#11816=ORIENTED_EDGE('',*,*,#8567,.T.);
#11817=ORIENTED_EDGE('',*,*,#8688,.F.);
#11818=ORIENTED_EDGE('',*,*,#8549,.F.);
#11819=ORIENTED_EDGE('',*,*,#8574,.F.);
#11820=ORIENTED_EDGE('',*,*,#8689,.F.);
#11821=ORIENTED_EDGE('',*,*,#8521,.T.);
#11822=ORIENTED_EDGE('',*,*,#8666,.F.);
#11823=ORIENTED_EDGE('',*,*,#8690,.T.);
#11824=ORIENTED_EDGE('',*,*,#8691,.F.);
#11825=ORIENTED_EDGE('',*,*,#8692,.F.);
#11826=ORIENTED_EDGE('',*,*,#8673,.F.);
#11827=ORIENTED_EDGE('',*,*,#8552,.F.);
#11828=ORIENTED_EDGE('',*,*,#8693,.F.);
#11829=ORIENTED_EDGE('',*,*,#8652,.T.);
#11830=ORIENTED_EDGE('',*,*,#8500,.F.);
#11831=ORIENTED_EDGE('',*,*,#8694,.T.);
#11832=ORIENTED_EDGE('',*,*,#8689,.T.);
#11833=ORIENTED_EDGE('',*,*,#8497,.F.);
#11834=ORIENTED_EDGE('',*,*,#8695,.T.);
#11835=ORIENTED_EDGE('',*,*,#8696,.F.);
#11836=ORIENTED_EDGE('',*,*,#8692,.T.);
#11837=ORIENTED_EDGE('',*,*,#8697,.F.);
#11838=ORIENTED_EDGE('',*,*,#8698,.T.);
#11839=ORIENTED_EDGE('',*,*,#8699,.F.);
#11840=ORIENTED_EDGE('',*,*,#8700,.F.);
#11841=ORIENTED_EDGE('',*,*,#8474,.F.);
#11842=ORIENTED_EDGE('',*,*,#8700,.T.);
#11843=ORIENTED_EDGE('',*,*,#8695,.F.);
#11844=ORIENTED_EDGE('',*,*,#8476,.F.);
#11845=ORIENTED_EDGE('',*,*,#8475,.F.);
#11846=ORIENTED_EDGE('',*,*,#8701,.F.);
#11847=ORIENTED_EDGE('',*,*,#8702,.T.);
#11848=ORIENTED_EDGE('',*,*,#8661,.F.);
#11849=ORIENTED_EDGE('',*,*,#8547,.T.);
#11850=ORIENTED_EDGE('',*,*,#8703,.F.);
#11851=ORIENTED_EDGE('',*,*,#8704,.T.);
#11852=ORIENTED_EDGE('',*,*,#8705,.T.);
#11853=ORIENTED_EDGE('',*,*,#8459,.F.);
#11854=ORIENTED_EDGE('',*,*,#8706,.T.);
#11855=ORIENTED_EDGE('',*,*,#8707,.T.);
#11856=ORIENTED_EDGE('',*,*,#8708,.T.);
#11857=ORIENTED_EDGE('',*,*,#8709,.T.);
#11858=ORIENTED_EDGE('',*,*,#8710,.T.);
#11859=ORIENTED_EDGE('',*,*,#8711,.T.);
#11860=ORIENTED_EDGE('',*,*,#8712,.T.);
#11861=ORIENTED_EDGE('',*,*,#8527,.F.);
#11862=ORIENTED_EDGE('',*,*,#8713,.T.);
#11863=ORIENTED_EDGE('',*,*,#8637,.T.);
#11864=ORIENTED_EDGE('',*,*,#8714,.F.);
#11865=ORIENTED_EDGE('',*,*,#8715,.F.);
#11866=ORIENTED_EDGE('',*,*,#8707,.F.);
#11867=ORIENTED_EDGE('',*,*,#8708,.F.);
#11868=ORIENTED_EDGE('',*,*,#8716,.T.);
#11869=ORIENTED_EDGE('',*,*,#8710,.F.);
#11870=ORIENTED_EDGE('',*,*,#8717,.F.);
#11871=ORIENTED_EDGE('',*,*,#8718,.F.);
#11872=ORIENTED_EDGE('',*,*,#8719,.T.);
#11873=ORIENTED_EDGE('',*,*,#8494,.F.);
#11874=ORIENTED_EDGE('',*,*,#8720,.F.);
#11875=ORIENTED_EDGE('',*,*,#8721,.F.);
#11876=ORIENTED_EDGE('',*,*,#8638,.T.);
#11877=ORIENTED_EDGE('',*,*,#8706,.F.);
#11878=ORIENTED_EDGE('',*,*,#8722,.F.);
#11879=ORIENTED_EDGE('',*,*,#8510,.T.);
#11880=ORIENTED_EDGE('',*,*,#8465,.F.);
#11881=ORIENTED_EDGE('',*,*,#8723,.T.);
#11882=ORIENTED_EDGE('',*,*,#8724,.T.);
#11883=ORIENTED_EDGE('',*,*,#8531,.T.);
#11884=ORIENTED_EDGE('',*,*,#8723,.F.);
#11885=ORIENTED_EDGE('',*,*,#8464,.F.);
#11886=ORIENTED_EDGE('',*,*,#8725,.F.);
#11887=ORIENTED_EDGE('',*,*,#8726,.T.);
#11888=ORIENTED_EDGE('',*,*,#8727,.T.);
#11889=ORIENTED_EDGE('',*,*,#8728,.T.);
#11890=ORIENTED_EDGE('',*,*,#8729,.T.);
#11891=ORIENTED_EDGE('',*,*,#8730,.T.);
#11892=ORIENTED_EDGE('',*,*,#8731,.T.);
#11893=ORIENTED_EDGE('',*,*,#8732,.F.);
#11894=ORIENTED_EDGE('',*,*,#8733,.F.);
#11895=ORIENTED_EDGE('',*,*,#8704,.F.);
#11896=ORIENTED_EDGE('',*,*,#8734,.F.);
#11897=ORIENTED_EDGE('',*,*,#8735,.T.);
#11898=ORIENTED_EDGE('',*,*,#8736,.T.);
#11899=ORIENTED_EDGE('',*,*,#8618,.F.);
#11900=ORIENTED_EDGE('',*,*,#8737,.T.);
#11901=ORIENTED_EDGE('',*,*,#8738,.F.);
#11902=ORIENTED_EDGE('',*,*,#8698,.F.);
#11903=ORIENTED_EDGE('',*,*,#8535,.T.);
#11904=ORIENTED_EDGE('',*,*,#8702,.F.);
#11905=ORIENTED_EDGE('',*,*,#8739,.F.);
#11906=ORIENTED_EDGE('',*,*,#8740,.F.);
#11907=ORIENTED_EDGE('',*,*,#8741,.F.);
#11908=ORIENTED_EDGE('',*,*,#8737,.F.);
#11909=ORIENTED_EDGE('',*,*,#8536,.T.);
#11910=ORIENTED_EDGE('',*,*,#8742,.F.);
#11911=ORIENTED_EDGE('',*,*,#8597,.F.);
#11912=ORIENTED_EDGE('',*,*,#8743,.T.);
#11913=ORIENTED_EDGE('',*,*,#8744,.F.);
#11914=ORIENTED_EDGE('',*,*,#8745,.T.);
#11915=ORIENTED_EDGE('',*,*,#8746,.F.);
#11916=ORIENTED_EDGE('',*,*,#8747,.T.);
#11917=ORIENTED_EDGE('',*,*,#8716,.F.);
#11918=ORIENTED_EDGE('',*,*,#8715,.T.);
#11919=ORIENTED_EDGE('',*,*,#8743,.F.);
#11920=ORIENTED_EDGE('',*,*,#8529,.F.);
#11921=ORIENTED_EDGE('',*,*,#8748,.F.);
#11922=ORIENTED_EDGE('',*,*,#8749,.F.);
#11923=ORIENTED_EDGE('',*,*,#8750,.T.);
#11924=ORIENTED_EDGE('',*,*,#8711,.F.);
#11925=ORIENTED_EDGE('',*,*,#8747,.F.);
#11926=ORIENTED_EDGE('',*,*,#8751,.F.);
#11927=ORIENTED_EDGE('',*,*,#8528,.F.);
#11928=ORIENTED_EDGE('',*,*,#8712,.F.);
#11929=ORIENTED_EDGE('',*,*,#8750,.F.);
#11930=ORIENTED_EDGE('',*,*,#8748,.T.);
#11931=ORIENTED_EDGE('',*,*,#8752,.T.);
#11932=ORIENTED_EDGE('',*,*,#8753,.T.);
#11933=ORIENTED_EDGE('',*,*,#8718,.T.);
#11934=ORIENTED_EDGE('',*,*,#8754,.T.);
#11935=ORIENTED_EDGE('',*,*,#8540,.T.);
#11936=ORIENTED_EDGE('',*,*,#8544,.T.);
#11937=ORIENTED_EDGE('',*,*,#8719,.F.);
#11938=ORIENTED_EDGE('',*,*,#8753,.F.);
#11939=ORIENTED_EDGE('',*,*,#8755,.F.);
#11940=ORIENTED_EDGE('',*,*,#8756,.F.);
#11941=ORIENTED_EDGE('',*,*,#8458,.F.);
#11942=ORIENTED_EDGE('',*,*,#8538,.T.);
#11943=ORIENTED_EDGE('',*,*,#8754,.F.);
#11944=ORIENTED_EDGE('',*,*,#8720,.T.);
#11945=ORIENTED_EDGE('',*,*,#8493,.F.);
#11946=ORIENTED_EDGE('',*,*,#8757,.T.);
#11947=ORIENTED_EDGE('',*,*,#8734,.T.);
#11948=ORIENTED_EDGE('',*,*,#8703,.T.);
#11949=ORIENTED_EDGE('',*,*,#8532,.F.);
#11950=ORIENTED_EDGE('',*,*,#8724,.F.);
#11951=ORIENTED_EDGE('',*,*,#8758,.F.);
#11952=ORIENTED_EDGE('',*,*,#8756,.T.);
#11953=ORIENTED_EDGE('',*,*,#8513,.T.);
#11954=ORIENTED_EDGE('',*,*,#8759,.T.);
#11955=ORIENTED_EDGE('',*,*,#8760,.T.);
#11956=ORIENTED_EDGE('',*,*,#8761,.T.);
#11957=ORIENTED_EDGE('',*,*,#8541,.T.);
#11958=ORIENTED_EDGE('',*,*,#8762,.T.);
#11959=ORIENTED_EDGE('',*,*,#8763,.F.);
#11960=ORIENTED_EDGE('',*,*,#8764,.T.);
#11961=ORIENTED_EDGE('',*,*,#8765,.T.);
#11962=ORIENTED_EDGE('',*,*,#8620,.T.);
#11963=ORIENTED_EDGE('',*,*,#8575,.T.);
#11964=ORIENTED_EDGE('',*,*,#8619,.T.);
#11965=ORIENTED_EDGE('',*,*,#8581,.T.);
#11966=ORIENTED_EDGE('',*,*,#8628,.T.);
#11967=ORIENTED_EDGE('',*,*,#8766,.T.);
#11968=ORIENTED_EDGE('',*,*,#8625,.T.);
#11969=ORIENTED_EDGE('',*,*,#8622,.T.);
#11970=ORIENTED_EDGE('',*,*,#8483,.T.);
#11971=ORIENTED_EDGE('',*,*,#8644,.F.);
#11972=ORIENTED_EDGE('',*,*,#8767,.T.);
#11973=ORIENTED_EDGE('',*,*,#8729,.F.);
#11974=ORIENTED_EDGE('',*,*,#8768,.T.);
#11975=ORIENTED_EDGE('',*,*,#8658,.T.);
#11976=ORIENTED_EDGE('',*,*,#8769,.T.);
#11977=ORIENTED_EDGE('',*,*,#8506,.F.);
#11978=ORIENTED_EDGE('',*,*,#8770,.T.);
#11979=ORIENTED_EDGE('',*,*,#8524,.F.);
#11980=ORIENTED_EDGE('',*,*,#8630,.T.);
#11981=ORIENTED_EDGE('',*,*,#8487,.T.);
#11982=ORIENTED_EDGE('',*,*,#8629,.T.);
#11983=ORIENTED_EDGE('',*,*,#8489,.T.);
#11984=ORIENTED_EDGE('',*,*,#8608,.T.);
#11985=ORIENTED_EDGE('',*,*,#8771,.T.);
#11986=ORIENTED_EDGE('',*,*,#8614,.F.);
#11987=ORIENTED_EDGE('',*,*,#8624,.T.);
#11988=ORIENTED_EDGE('',*,*,#8612,.T.);
#11989=ORIENTED_EDGE('',*,*,#8772,.T.);
#11990=ORIENTED_EDGE('',*,*,#8773,.F.);
#11991=ORIENTED_EDGE('',*,*,#8774,.T.);
#11992=ORIENTED_EDGE('',*,*,#8749,.T.);
#11993=ORIENTED_EDGE('',*,*,#8751,.T.);
#11994=ORIENTED_EDGE('',*,*,#8746,.T.);
#11995=ORIENTED_EDGE('',*,*,#8714,.T.);
#11996=ORIENTED_EDGE('',*,*,#8636,.T.);
#11997=ORIENTED_EDGE('',*,*,#8639,.T.);
#11998=ORIENTED_EDGE('',*,*,#8478,.T.);
#11999=ORIENTED_EDGE('',*,*,#8509,.T.);
#12000=ORIENTED_EDGE('',*,*,#8525,.F.);
#12001=ORIENTED_EDGE('',*,*,#8775,.F.);
#12002=ORIENTED_EDGE('',*,*,#8462,.F.);
#12003=ORIENTED_EDGE('',*,*,#8776,.F.);
#12004=ORIENTED_EDGE('',*,*,#8777,.T.);
#12005=ORIENTED_EDGE('',*,*,#8778,.T.);
#12006=ORIENTED_EDGE('',*,*,#8744,.T.);
#12007=ORIENTED_EDGE('',*,*,#8779,.T.);
#12008=ORIENTED_EDGE('',*,*,#8780,.T.);
#12009=ORIENTED_EDGE('',*,*,#8781,.T.);
#12010=ORIENTED_EDGE('',*,*,#8782,.T.);
#12011=ORIENTED_EDGE('',*,*,#8634,.T.);
#12012=ORIENTED_EDGE('',*,*,#8783,.T.);
#12013=ORIENTED_EDGE('',*,*,#8784,.T.);
#12014=ORIENTED_EDGE('',*,*,#8785,.T.);
#12015=ORIENTED_EDGE('',*,*,#8773,.T.);
#12016=ORIENTED_EDGE('',*,*,#8786,.T.);
#12017=ORIENTED_EDGE('',*,*,#8787,.T.);
#12018=ORIENTED_EDGE('',*,*,#8788,.T.);
#12019=ORIENTED_EDGE('',*,*,#8598,.F.);
#12020=ORIENTED_EDGE('',*,*,#8789,.T.);
#12021=ORIENTED_EDGE('',*,*,#8730,.F.);
#12022=ORIENTED_EDGE('',*,*,#8790,.T.);
#12023=ORIENTED_EDGE('',*,*,#8601,.T.);
#12024=ORIENTED_EDGE('',*,*,#8485,.T.);
#12025=ORIENTED_EDGE('',*,*,#8603,.F.);
#12026=ORIENTED_EDGE('',*,*,#8579,.T.);
#12027=ORIENTED_EDGE('',*,*,#8616,.F.);
#12028=ORIENTED_EDGE('',*,*,#8791,.T.);
#12029=ORIENTED_EDGE('',*,*,#8606,.F.);
#12030=ORIENTED_EDGE('',*,*,#8792,.T.);
#12031=ORIENTED_EDGE('',*,*,#8787,.F.);
#12032=ORIENTED_EDGE('',*,*,#8632,.T.);
#12033=ORIENTED_EDGE('',*,*,#8610,.F.);
#12034=ORIENTED_EDGE('',*,*,#8793,.T.);
#12035=ORIENTED_EDGE('',*,*,#8763,.T.);
#12036=ORIENTED_EDGE('',*,*,#8794,.T.);
#12037=ORIENTED_EDGE('',*,*,#8626,.T.);
#12038=ORIENTED_EDGE('',*,*,#8766,.F.);
#12039=ORIENTED_EDGE('',*,*,#8627,.T.);
#12040=ORIENTED_EDGE('',*,*,#8792,.F.);
#12041=ORIENTED_EDGE('',*,*,#8795,.T.);
#12042=ORIENTED_EDGE('',*,*,#8774,.F.);
#12043=ORIENTED_EDGE('',*,*,#8796,.F.);
#12044=ORIENTED_EDGE('',*,*,#8765,.F.);
#12045=ORIENTED_EDGE('',*,*,#8793,.F.);
#12046=ORIENTED_EDGE('',*,*,#8613,.F.);
#12047=ORIENTED_EDGE('',*,*,#8795,.F.);
#12048=ORIENTED_EDGE('',*,*,#8764,.F.);
#12049=ORIENTED_EDGE('',*,*,#8759,.F.);
#12050=ORIENTED_EDGE('',*,*,#8512,.T.);
#12051=ORIENTED_EDGE('',*,*,#8599,.F.);
#12052=ORIENTED_EDGE('',*,*,#8797,.T.);
#12053=ORIENTED_EDGE('',*,*,#8796,.T.);
#12054=ORIENTED_EDGE('',*,*,#8788,.F.);
#12055=ORIENTED_EDGE('',*,*,#8794,.F.);
#12056=ORIENTED_EDGE('',*,*,#8762,.F.);
#12057=ORIENTED_EDGE('',*,*,#8798,.T.);
#12058=ORIENTED_EDGE('',*,*,#8760,.F.);
#12059=ORIENTED_EDGE('',*,*,#8797,.F.);
#12060=ORIENTED_EDGE('',*,*,#8790,.F.);
#12061=ORIENTED_EDGE('',*,*,#8542,.F.);
#12062=ORIENTED_EDGE('',*,*,#8761,.F.);
#12063=ORIENTED_EDGE('',*,*,#8798,.F.);
#12064=ORIENTED_EDGE('',*,*,#8736,.F.);
#12065=ORIENTED_EDGE('',*,*,#8799,.F.);
#12066=ORIENTED_EDGE('',*,*,#8800,.F.);
#12067=ORIENTED_EDGE('',*,*,#8742,.T.);
#12068=ORIENTED_EDGE('',*,*,#8740,.T.);
#12069=ORIENTED_EDGE('',*,*,#8543,.T.);
#12070=ORIENTED_EDGE('',*,*,#8799,.T.);
#12071=ORIENTED_EDGE('',*,*,#8735,.F.);
#12072=ORIENTED_EDGE('',*,*,#8757,.F.);
#12073=ORIENTED_EDGE('',*,*,#8496,.F.);
#12074=ORIENTED_EDGE('',*,*,#8667,.F.);
#12075=ORIENTED_EDGE('',*,*,#8690,.F.);
#12076=ORIENTED_EDGE('',*,*,#8665,.F.);
#12077=ORIENTED_EDGE('',*,*,#8558,.F.);
#12078=ORIENTED_EDGE('',*,*,#8801,.T.);
#12079=ORIENTED_EDGE('',*,*,#8802,.T.);
#12080=ORIENTED_EDGE('',*,*,#8726,.F.);
#12081=ORIENTED_EDGE('',*,*,#8767,.F.);
#12082=ORIENTED_EDGE('',*,*,#8643,.F.);
#12083=ORIENTED_EDGE('',*,*,#8517,.T.);
#12084=ORIENTED_EDGE('',*,*,#8803,.F.);
#12085=ORIENTED_EDGE('',*,*,#8804,.T.);
#12086=ORIENTED_EDGE('',*,*,#8660,.F.);
#12087=ORIENTED_EDGE('',*,*,#8505,.F.);
#12088=ORIENTED_EDGE('',*,*,#8805,.T.);
#12089=ORIENTED_EDGE('',*,*,#8641,.F.);
#12090=ORIENTED_EDGE('',*,*,#8770,.F.);
#12091=ORIENTED_EDGE('',*,*,#8655,.T.);
#12092=ORIENTED_EDGE('',*,*,#8803,.T.);
#12093=ORIENTED_EDGE('',*,*,#8516,.T.);
#12094=ORIENTED_EDGE('',*,*,#8806,.T.);
#12095=ORIENTED_EDGE('',*,*,#8807,.T.);
#12096=ORIENTED_EDGE('',*,*,#8808,.T.);
#12097=ORIENTED_EDGE('',*,*,#8503,.F.);
#12098=ORIENTED_EDGE('',*,*,#8522,.T.);
#12099=ORIENTED_EDGE('',*,*,#8807,.F.);
#12100=ORIENTED_EDGE('',*,*,#8809,.T.);
#12101=ORIENTED_EDGE('',*,*,#8801,.F.);
#12102=ORIENTED_EDGE('',*,*,#8642,.F.);
#12103=ORIENTED_EDGE('',*,*,#8810,.F.);
#12104=ORIENTED_EDGE('',*,*,#8809,.F.);
#12105=ORIENTED_EDGE('',*,*,#8806,.F.);
#12106=ORIENTED_EDGE('',*,*,#8519,.F.);
#12107=ORIENTED_EDGE('',*,*,#8727,.F.);
#12108=ORIENTED_EDGE('',*,*,#8802,.F.);
#12109=ORIENTED_EDGE('',*,*,#8810,.T.);
#12110=ORIENTED_EDGE('',*,*,#8805,.F.);
#12111=ORIENTED_EDGE('',*,*,#8504,.F.);
#12112=ORIENTED_EDGE('',*,*,#8808,.F.);
#12113=ORIENTED_EDGE('',*,*,#8697,.T.);
#12114=ORIENTED_EDGE('',*,*,#8691,.T.);
#12115=ORIENTED_EDGE('',*,*,#8551,.T.);
#12116=ORIENTED_EDGE('',*,*,#8498,.F.);
#12117=ORIENTED_EDGE('',*,*,#8728,.F.);
#12118=ORIENTED_EDGE('',*,*,#8518,.T.);
#12119=ORIENTED_EDGE('',*,*,#8659,.F.);
#12120=ORIENTED_EDGE('',*,*,#8768,.F.);
#12121=ORIENTED_EDGE('',*,*,#8738,.T.);
#12122=ORIENTED_EDGE('',*,*,#8741,.T.);
#12123=ORIENTED_EDGE('',*,*,#8800,.T.);
#12124=ORIENTED_EDGE('',*,*,#8739,.T.);
#12125=ORIENTED_EDGE('',*,*,#8701,.T.);
#12126=ORIENTED_EDGE('',*,*,#8546,.T.);
#12127=ORIENTED_EDGE('',*,*,#8811,.F.);
#12128=ORIENTED_EDGE('',*,*,#8722,.T.);
#12129=ORIENTED_EDGE('',*,*,#8709,.F.);
#12130=ORIENTED_EDGE('',*,*,#8717,.T.);
#12131=ORIENTED_EDGE('',*,*,#8713,.F.);
#12132=ORIENTED_EDGE('',*,*,#8526,.T.);
#12133=ORIENTED_EDGE('',*,*,#8507,.T.);
#12134=ORIENTED_EDGE('',*,*,#8769,.F.);
#12135=ORIENTED_EDGE('',*,*,#8467,.F.);
#12136=ORIENTED_EDGE('',*,*,#8454,.F.);
#12137=ORIENTED_EDGE('',*,*,#8657,.F.);
#12138=ORIENTED_EDGE('',*,*,#8648,.T.);
#12139=ORIENTED_EDGE('',*,*,#8651,.T.);
#12140=ORIENTED_EDGE('',*,*,#8693,.T.);
#12141=ORIENTED_EDGE('',*,*,#8573,.T.);
#12142=ORIENTED_EDGE('',*,*,#8684,.T.);
#12143=ORIENTED_EDGE('',*,*,#8686,.T.);
#12144=ORIENTED_EDGE('',*,*,#8687,.T.);
#12145=ORIENTED_EDGE('',*,*,#8664,.T.);
#12146=ORIENTED_EDGE('',*,*,#8812,.T.);
#12147=ORIENTED_EDGE('',*,*,#8681,.T.);
#12148=ORIENTED_EDGE('',*,*,#8676,.T.);
#12149=ORIENTED_EDGE('',*,*,#8674,.T.);
#12150=ORIENTED_EDGE('',*,*,#8696,.T.);
#12151=ORIENTED_EDGE('',*,*,#8699,.T.);
#12152=ORIENTED_EDGE('',*,*,#8446,.F.);
#12153=ORIENTED_EDGE('',*,*,#8480,.T.);
#12154=ORIENTED_EDGE('',*,*,#8640,.T.);
#12155=ORIENTED_EDGE('',*,*,#8721,.T.);
#12156=ORIENTED_EDGE('',*,*,#8811,.T.);
#12157=ORIENTED_EDGE('',*,*,#8545,.T.);
#12158=ORIENTED_EDGE('',*,*,#8813,.T.);
#12159=ORIENTED_EDGE('',*,*,#8781,.F.);
#12160=ORIENTED_EDGE('',*,*,#8814,.F.);
#12161=ORIENTED_EDGE('',*,*,#8615,.F.);
#12162=ORIENTED_EDGE('',*,*,#8815,.T.);
#12163=ORIENTED_EDGE('',*,*,#8607,.F.);
#12164=ORIENTED_EDGE('',*,*,#8816,.F.);
#12165=ORIENTED_EDGE('',*,*,#8779,.F.);
#12166=ORIENTED_EDGE('',*,*,#8550,.T.);
#12167=ORIENTED_EDGE('',*,*,#8688,.T.);
#12168=ORIENTED_EDGE('',*,*,#8694,.F.);
#12169=ORIENTED_EDGE('',*,*,#8499,.F.);
#12170=ORIENTED_EDGE('',*,*,#8814,.T.);
#12171=ORIENTED_EDGE('',*,*,#8780,.F.);
#12172=ORIENTED_EDGE('',*,*,#8816,.T.);
#12173=ORIENTED_EDGE('',*,*,#8791,.F.);
#12174=ORIENTED_EDGE('',*,*,#8815,.F.);
#12175=ORIENTED_EDGE('',*,*,#8782,.F.);
#12176=ORIENTED_EDGE('',*,*,#8813,.F.);
#12177=ORIENTED_EDGE('',*,*,#8771,.F.);
#12178=ORIENTED_EDGE('',*,*,#8784,.F.);
#12179=ORIENTED_EDGE('',*,*,#8817,.T.);
#12180=ORIENTED_EDGE('',*,*,#8772,.F.);
#12181=ORIENTED_EDGE('',*,*,#8818,.T.);
#12182=ORIENTED_EDGE('',*,*,#8818,.F.);
#12183=ORIENTED_EDGE('',*,*,#8611,.F.);
#12184=ORIENTED_EDGE('',*,*,#8631,.F.);
#12185=ORIENTED_EDGE('',*,*,#8785,.F.);
#12186=ORIENTED_EDGE('',*,*,#8817,.F.);
#12187=ORIENTED_EDGE('',*,*,#8783,.F.);
#12188=ORIENTED_EDGE('',*,*,#8633,.T.);
#12189=ORIENTED_EDGE('',*,*,#8786,.F.);
#12190=ORIENTED_EDGE('',*,*,#8819,.T.);
#12191=ORIENTED_EDGE('',*,*,#8789,.F.);
#12192=ORIENTED_EDGE('',*,*,#8745,.F.);
#12193=ORIENTED_EDGE('',*,*,#8778,.F.);
#12194=ORIENTED_EDGE('',*,*,#8820,.F.);
#12195=ORIENTED_EDGE('',*,*,#8731,.F.);
#12196=ORIENTED_EDGE('',*,*,#8819,.F.);
#12197=ORIENTED_EDGE('',*,*,#8777,.F.);
#12198=ORIENTED_EDGE('',*,*,#8705,.F.);
#12199=ORIENTED_EDGE('',*,*,#8733,.T.);
#12200=ORIENTED_EDGE('',*,*,#8821,.T.);
#12201=ORIENTED_EDGE('',*,*,#8460,.F.);
#12202=ORIENTED_EDGE('',*,*,#8821,.F.);
#12203=ORIENTED_EDGE('',*,*,#8732,.T.);
#12204=ORIENTED_EDGE('',*,*,#8820,.T.);
#12205=ORIENTED_EDGE('',*,*,#8776,.T.);
#12206=ORIENTED_EDGE('',*,*,#8461,.F.);
#12207=ORIENTED_EDGE('',*,*,#8533,.T.);
#12208=ORIENTED_EDGE('',*,*,#8758,.T.);
#12209=ORIENTED_EDGE('',*,*,#8725,.T.);
#12210=ORIENTED_EDGE('',*,*,#8463,.T.);
#12211=ORIENTED_EDGE('',*,*,#8775,.T.);
#12212=ORIENTED_EDGE('',*,*,#8812,.F.);
#12213=ORIENTED_EDGE('',*,*,#8663,.T.);
#12214=ORIENTED_EDGE('',*,*,#8561,.F.);
#12215=ORIENTED_EDGE('',*,*,#8822,.F.);
#12216=ORIENTED_EDGE('',*,*,#8823,.F.);
#12217=ORIENTED_EDGE('',*,*,#8678,.T.);
#12218=ORIENTED_EDGE('',*,*,#8556,.T.);
#12219=ORIENTED_EDGE('',*,*,#8824,.T.);
#12220=ORIENTED_EDGE('',*,*,#8822,.T.);
#12221=ORIENTED_EDGE('',*,*,#8560,.T.);
#12222=ORIENTED_EDGE('',*,*,#8668,.T.);
#12223=ORIENTED_EDGE('',*,*,#8824,.F.);
#12224=ORIENTED_EDGE('',*,*,#8682,.T.);
#12225=ORIENTED_EDGE('',*,*,#8679,.T.);
#12226=ORIENTED_EDGE('',*,*,#8823,.T.);
#12227=ORIENTED_EDGE('',*,*,#8646,.F.);
#12228=ORIENTED_EDGE('',*,*,#8656,.F.);
#12229=ORIENTED_EDGE('',*,*,#8804,.F.);
#12230=ORIENTED_EDGE('',*,*,#8654,.F.);
#12231=ORIENTED_EDGE('',*,*,#8539,.T.);
#12232=ORIENTED_EDGE('',*,*,#8514,.T.);
#12233=ORIENTED_EDGE('',*,*,#8755,.T.);
#12234=ORIENTED_EDGE('',*,*,#8752,.F.);
#12235=ORIENTED_EDGE('',*,*,#8450,.T.);
#12236=ORIENTED_EDGE('',*,*,#8444,.T.);
#14256=TOROIDAL_SURFACE('',#15859,9.,0.8);
#14257=TOROIDAL_SURFACE('',#15867,9.,0.8);
#14258=TOROIDAL_SURFACE('',#15875,3.5,0.8);
#14259=TOROIDAL_SURFACE('',#15878,4.,0.8);
#14260=TOROIDAL_SURFACE('',#15881,2.,0.8);
#14261=TOROIDAL_SURFACE('',#15884,15.,0.8);
#14262=TOROIDAL_SURFACE('',#15911,4.5,0.5);
#14263=TOROIDAL_SURFACE('',#15914,10.,0.5);
#14264=TOROIDAL_SURFACE('',#15917,6.5,0.5);
#14265=TOROIDAL_SURFACE('',#15930,3.3,0.5);
#14266=TOROIDAL_SURFACE('',#15934,4.,0.5);
#14267=TOROIDAL_SURFACE('',#15939,1.5,1.);
#14268=TOROIDAL_SURFACE('',#15956,16.5,0.5);
#14269=TOROIDAL_SURFACE('',#15959,3.,0.5);
#14270=TOROIDAL_SURFACE('',#15971,3.,0.5);
#14271=TOROIDAL_SURFACE('',#15974,5.5,0.5);
#14272=TOROIDAL_SURFACE('',#15977,11.,0.5);
#14273=TOROIDAL_SURFACE('',#15998,11.,0.5);
#14274=TOROIDAL_SURFACE('',#16005,6.5,0.5);
#14275=TOROIDAL_SURFACE('',#16008,1.5,0.5);
#14276=TOROIDAL_SURFACE('',#16025,3.,0.5);
#14277=TOROIDAL_SURFACE('',#16033,3.,0.5);
#14278=TOROIDAL_SURFACE('',#16048,16.5,0.5);
#14279=TOROIDAL_SURFACE('',#16051,16.5,0.5);
#14280=TOROIDAL_SURFACE('',#16054,3.,0.5);
#14281=TOROIDAL_SURFACE('',#16059,14.5,1.);
#14282=TOROIDAL_SURFACE('',#16066,10.,0.5);
#14283=TOROIDAL_SURFACE('',#16086,1.5,0.5);
#14284=TOROIDAL_SURFACE('',#16089,4.3,0.5);
#14285=TOROIDAL_SURFACE('',#16096,1.5,0.5);
#14286=TOROIDAL_SURFACE('',#16133,5.5,0.5);
#14287=TOROIDAL_SURFACE('',#16134,11.,0.5);
#14288=TOROIDAL_SURFACE('',#16138,5.5,0.5);
#14289=TOROIDAL_SURFACE('',#16142,1.5,1.);
#14290=TOROIDAL_SURFACE('',#16146,18.,1.);
#14291=TOROIDAL_SURFACE('',#16158,6.5,0.5);
#14292=TOROIDAL_SURFACE('',#16159,10.,0.5);
#14293=TOROIDAL_SURFACE('',#16160,10.,0.5);
#14294=TOROIDAL_SURFACE('',#16163,6.5,0.5);
#14295=TOROIDAL_SURFACE('',#16167,14.5,1.);
#14639=ADVANCED_FACE('',(#4004),#14256,.T.);
#14640=ADVANCED_FACE('',(#4005),#14257,.T.);
#14641=ADVANCED_FACE('',(#4006),#14258,.T.);
#14642=ADVANCED_FACE('',(#4007),#14259,.T.);
#14643=ADVANCED_FACE('',(#4008),#14260,.T.);
#14644=ADVANCED_FACE('',(#4009),#14261,.T.);
#14645=ADVANCED_FACE('',(#4010),#3486,.T.);
#14646=ADVANCED_FACE('',(#4011),#1041,.T.);
#14647=ADVANCED_FACE('',(#4012),#3487,.T.);
#14648=ADVANCED_FACE('',(#4013),#3488,.F.);
#14649=ADVANCED_FACE('',(#4014,#224),#3489,.T.);
#14650=ADVANCED_FACE('',(#4015),#14262,.T.);
#14651=ADVANCED_FACE('',(#4016),#14263,.F.);
#14652=ADVANCED_FACE('',(#4017),#14264,.F.);
#14653=ADVANCED_FACE('',(#4018),#3490,.T.);
#14654=ADVANCED_FACE('',(#4019),#3491,.T.);
#14655=ADVANCED_FACE('',(#4020),#14265,.T.);
#14656=ADVANCED_FACE('',(#4021),#14266,.T.);
#14657=ADVANCED_FACE('',(#4022),#14267,.T.);
#14658=ADVANCED_FACE('',(#4023),#3492,.F.);
#14659=ADVANCED_FACE('',(#4024),#3493,.T.);
#14660=ADVANCED_FACE('',(#4025),#3494,.T.);
#14661=ADVANCED_FACE('',(#4026),#3495,.T.);
#14662=ADVANCED_FACE('',(#4027),#14268,.T.);
#14663=ADVANCED_FACE('',(#4028),#14269,.F.);
#14664=ADVANCED_FACE('',(#4029),#3496,.T.);
#14665=ADVANCED_FACE('',(#4030),#3497,.T.);
#14666=ADVANCED_FACE('',(#4031),#14270,.F.);
#14667=ADVANCED_FACE('',(#4032),#14271,.T.);
#14668=ADVANCED_FACE('',(#4033),#14272,.T.);
#14669=ADVANCED_FACE('',(#4034),#149,.F.);
#14670=ADVANCED_FACE('',(#4035),#150,.T.);
#14671=ADVANCED_FACE('',(#4036),#151,.T.);
#14672=ADVANCED_FACE('',(#4037),#3498,.T.);
#14673=ADVANCED_FACE('',(#4038),#3499,.T.);
#14674=ADVANCED_FACE('',(#4039),#530,.F.);
#14675=ADVANCED_FACE('',(#4040),#152,.T.);
#14676=ADVANCED_FACE('',(#4041),#153,.T.);
#14677=ADVANCED_FACE('',(#4042),#531,.T.);
#14678=ADVANCED_FACE('',(#4043),#154,.F.);
#14679=ADVANCED_FACE('',(#4044),#3500,.T.);
#14680=ADVANCED_FACE('',(#4045),#532,.F.);
#14681=ADVANCED_FACE('',(#4046),#533,.F.);
#14682=ADVANCED_FACE('',(#4047),#534,.F.);
#14683=ADVANCED_FACE('',(#4048),#535,.F.);
#14684=ADVANCED_FACE('',(#4049),#536,.F.);
#14685=ADVANCED_FACE('',(#4050),#537,.F.);
#14686=ADVANCED_FACE('',(#4051),#538,.T.);
#14687=ADVANCED_FACE('',(#4052),#3501,.T.);
#14688=ADVANCED_FACE('',(#4053),#3502,.T.);
#14689=ADVANCED_FACE('',(#4054),#14273,.T.);
#14690=ADVANCED_FACE('',(#4055),#3503,.T.);
#14691=ADVANCED_FACE('',(#4056),#3504,.T.);
#14692=ADVANCED_FACE('',(#4057),#3505,.F.);
#14693=ADVANCED_FACE('',(#4058),#3506,.F.);
#14694=ADVANCED_FACE('',(#4059),#14274,.F.);
#14695=ADVANCED_FACE('',(#4060),#14275,.T.);
#14696=ADVANCED_FACE('',(#4061),#3507,.T.);
#14697=ADVANCED_FACE('',(#4062),#539,.T.);
#14698=ADVANCED_FACE('',(#4063),#155,.F.);
#14699=ADVANCED_FACE('',(#4064),#3508,.F.);
#14700=ADVANCED_FACE('',(#4065),#156,.F.);
#14701=ADVANCED_FACE('',(#4066),#540,.F.);
#14702=ADVANCED_FACE('',(#4067),#541,.F.);
#14703=ADVANCED_FACE('',(#4068),#542,.T.);
#14704=ADVANCED_FACE('',(#4069),#14276,.F.);
#14705=ADVANCED_FACE('',(#4070),#543,.F.);
#14706=ADVANCED_FACE('',(#4071),#544,.T.);
#14707=ADVANCED_FACE('',(#4072),#545,.F.);
#14708=ADVANCED_FACE('',(#4073),#546,.T.);
#14709=ADVANCED_FACE('',(#4074),#14277,.F.);
#14710=ADVANCED_FACE('',(#4075),#3509,.F.);
#14711=ADVANCED_FACE('',(#4076),#157,.F.);
#14712=ADVANCED_FACE('',(#4077),#3510,.T.);
#14713=ADVANCED_FACE('',(#4078),#3511,.F.);
#14714=ADVANCED_FACE('',(#4079),#158,.F.);
#14715=ADVANCED_FACE('',(#4080),#3512,.F.);
#14716=ADVANCED_FACE('',(#4081),#159,.F.);
#14717=ADVANCED_FACE('',(#4082),#547,.F.);
#14718=ADVANCED_FACE('',(#4083),#548,.F.);
#14719=ADVANCED_FACE('',(#4084),#160,.F.);
#14720=ADVANCED_FACE('',(#4085),#14278,.T.);
#14721=ADVANCED_FACE('',(#4086),#14279,.T.);
#14722=ADVANCED_FACE('',(#4087),#14280,.F.);
#14723=ADVANCED_FACE('',(#4088),#161,.F.);
#14724=ADVANCED_FACE('',(#4089),#3513,.F.);
#14725=ADVANCED_FACE('',(#4090),#14281,.F.);
#14726=ADVANCED_FACE('',(#4091),#3514,.T.);
#14727=ADVANCED_FACE('',(#4092),#549,.F.);
#14728=ADVANCED_FACE('',(#4093),#14282,.T.);
#14729=ADVANCED_FACE('',(#4094),#3515,.F.);
#14730=ADVANCED_FACE('',(#4095),#3516,.F.);
#14731=ADVANCED_FACE('',(#4096),#3517,.F.);
#14732=ADVANCED_FACE('',(#4097),#550,.T.);
#14733=ADVANCED_FACE('',(#4098),#551,.T.);
#14734=ADVANCED_FACE('',(#4099),#552,.F.);
#14735=ADVANCED_FACE('',(#4100),#553,.F.);
#14736=ADVANCED_FACE('',(#4101),#3518,.F.);
#14737=ADVANCED_FACE('',(#4102),#162,.T.);
#14738=ADVANCED_FACE('',(#4103),#163,.T.);
#14739=ADVANCED_FACE('',(#4104),#3519,.F.);
#14740=ADVANCED_FACE('',(#4105),#14283,.T.);
#14741=ADVANCED_FACE('',(#4106),#14284,.F.);
#14742=ADVANCED_FACE('',(#4107),#3520,.T.);
#14743=ADVANCED_FACE('',(#4108),#164,.F.);
#14744=ADVANCED_FACE('',(#4109),#3521,.T.);
#14745=ADVANCED_FACE('',(#4110),#14285,.T.);
#14746=ADVANCED_FACE('',(#4111),#554,.T.);
#14747=ADVANCED_FACE('',(#4112),#555,.T.);
#14748=ADVANCED_FACE('',(#4113,#225,#226,#227,#228),#556,.F.);
#14749=ADVANCED_FACE('',(#4114,#229),#557,.F.);
#14750=ADVANCED_FACE('',(#4115),#558,.F.);
#14751=ADVANCED_FACE('',(#4116),#3522,.F.);
#14752=ADVANCED_FACE('',(#4117),#3523,.F.);
#14753=ADVANCED_FACE('',(#4118),#559,.F.);
#14754=ADVANCED_FACE('',(#4119),#560,.F.);
#14755=ADVANCED_FACE('',(#4120),#561,.F.);
#14756=ADVANCED_FACE('',(#4121),#562,.F.);
#14757=ADVANCED_FACE('',(#4122),#3524,.T.);
#14758=ADVANCED_FACE('',(#4123),#3525,.F.);
#14759=ADVANCED_FACE('',(#4124),#3526,.T.);
#14760=ADVANCED_FACE('',(#4125),#3527,.T.);
#14761=ADVANCED_FACE('',(#4126),#14286,.T.);
#14762=ADVANCED_FACE('',(#4127),#14287,.T.);
#14763=ADVANCED_FACE('',(#4128),#3528,.T.);
#14764=ADVANCED_FACE('',(#4129),#3529,.T.);
#14765=ADVANCED_FACE('',(#4130),#3530,.T.);
#14766=ADVANCED_FACE('',(#4131),#14288,.T.);
#14767=ADVANCED_FACE('',(#4132),#3531,.T.);
#14768=ADVANCED_FACE('',(#4133),#563,.T.);
#14769=ADVANCED_FACE('',(#4134),#3532,.T.);
#14770=ADVANCED_FACE('',(#4135),#14289,.T.);
#14771=ADVANCED_FACE('',(#4136),#3533,.T.);
#14772=ADVANCED_FACE('',(#4137),#3534,.T.);
#14773=ADVANCED_FACE('',(#4138),#14290,.F.);
#14774=ADVANCED_FACE('',(#4139,#230),#564,.F.);
#14775=ADVANCED_FACE('',(#4140),#3535,.T.);
#14776=ADVANCED_FACE('',(#4141),#3536,.T.);
#14777=ADVANCED_FACE('',(#4142),#165,.T.);
#14778=ADVANCED_FACE('',(#4143),#166,.T.);
#14779=ADVANCED_FACE('',(#4144),#3537,.T.);
#14780=ADVANCED_FACE('',(#4145,#231),#565,.T.);
#14781=ADVANCED_FACE('',(#4146),#566,.F.);
#14782=ADVANCED_FACE('',(#4147),#3538,.F.);
#14783=ADVANCED_FACE('',(#4148),#3539,.F.);
#14784=ADVANCED_FACE('',(#4149),#167,.T.);
#14785=ADVANCED_FACE('',(#4150),#14291,.F.);
#14786=ADVANCED_FACE('',(#4151),#14292,.F.);
#14787=ADVANCED_FACE('',(#4152),#14293,.F.);
#14788=ADVANCED_FACE('',(#4153),#3540,.F.);
#14789=ADVANCED_FACE('',(#4154),#3541,.F.);
#14790=ADVANCED_FACE('',(#4155),#14294,.F.);
#14791=ADVANCED_FACE('',(#4156),#3542,.F.);
#14792=ADVANCED_FACE('',(#4157),#3543,.T.);
#14793=ADVANCED_FACE('',(#4158),#14295,.F.);
#14794=ADVANCED_FACE('',(#4159),#567,.T.);
#14795=ADVANCED_FACE('',(#4160),#568,.F.);
#14796=ADVANCED_FACE('',(#4161),#569,.F.);
#14797=ADVANCED_FACE('',(#4162),#570,.F.);
#14798=ADVANCED_FACE('',(#4163),#3544,.T.);
#14799=ADVANCED_FACE('',(#4164),#571,.F.);
#14800=ADVANCED_FACE('',(#4165),#572,.F.);
#14801=ADVANCED_FACE('',(#4166),#573,.T.);
#15196=CLOSED_SHELL('',(#14639,#14640,#14641,#14642,#14643,#14644,#14645,
#14646,#14647,#14648,#14649,#14650,#14651,#14652,#14653,#14654,#14655,#14656,
#14657,#14658,#14659,#14660,#14661,#14662,#14663,#14664,#14665,#14666,#14667,
#14668,#14669,#14670,#14671,#14672,#14673,#14674,#14675,#14676,#14677,#14678,
#14679,#14680,#14681,#14682,#14683,#14684,#14685,#14686,#14687,#14688,#14689,
#14690,#14691,#14692,#14693,#14694,#14695,#14696,#14697,#14698,#14699,#14700,
#14701,#14702,#14703,#14704,#14705,#14706,#14707,#14708,#14709,#14710,#14711,
#14712,#14713,#14714,#14715,#14716,#14717,#14718,#14719,#14720,#14721,#14722,
#14723,#14724,#14725,#14726,#14727,#14728,#14729,#14730,#14731,#14732,#14733,
#14734,#14735,#14736,#14737,#14738,#14739,#14740,#14741,#14742,#14743,#14744,
#14745,#14746,#14747,#14748,#14749,#14750,#14751,#14752,#14753,#14754,#14755,
#14756,#14757,#14758,#14759,#14760,#14761,#14762,#14763,#14764,#14765,#14766,
#14767,#14768,#14769,#14770,#14771,#14772,#14773,#14774,#14775,#14776,#14777,
#14778,#14779,#14780,#14781,#14782,#14783,#14784,#14785,#14786,#14787,#14788,
#14789,#14790,#14791,#14792,#14793,#14794,#14795,#14796,#14797,#14798,#14799,
#14800,#14801));
#15858=AXIS2_PLACEMENT_3D('',#35149,#18577,#18578);
#15859=AXIS2_PLACEMENT_3D('',#35150,#18579,#18580);
#15860=AXIS2_PLACEMENT_3D('',#35153,#18581,#18582);
#15861=AXIS2_PLACEMENT_3D('',#35154,#18583,#18584);
#15862=AXIS2_PLACEMENT_3D('',#35156,#18585,#18586);
#15863=AXIS2_PLACEMENT_3D('',#35158,#18587,#18588);
#15864=AXIS2_PLACEMENT_3D('',#35160,#18589,#18590);
#15865=AXIS2_PLACEMENT_3D('',#35162,#18591,#18592);
#15866=AXIS2_PLACEMENT_3D('',#35163,#18593,#18594);
#15867=AXIS2_PLACEMENT_3D('',#35164,#18595,#18596);
#15868=AXIS2_PLACEMENT_3D('',#35167,#18597,#18598);
#15869=AXIS2_PLACEMENT_3D('',#35169,#18599,#18600);
#15870=AXIS2_PLACEMENT_3D('',#35171,#18601,#18602);
#15871=AXIS2_PLACEMENT_3D('',#35172,#18603,#18604);
#15872=AXIS2_PLACEMENT_3D('',#35174,#18605,#18606);
#15873=AXIS2_PLACEMENT_3D('',#35176,#18607,#18608);
#15874=AXIS2_PLACEMENT_3D('',#35177,#18609,#18610);
#15875=AXIS2_PLACEMENT_3D('',#35178,#18611,#18612);
#15876=AXIS2_PLACEMENT_3D('',#35362,#18613,#18614);
#15877=AXIS2_PLACEMENT_3D('',#35363,#18615,#18616);
#15878=AXIS2_PLACEMENT_3D('',#35364,#18617,#18618);
#15879=AXIS2_PLACEMENT_3D('',#35366,#18619,#18620);
#15880=AXIS2_PLACEMENT_3D('',#35368,#18621,#18622);
#15881=AXIS2_PLACEMENT_3D('',#35538,#18623,#18624);
#15882=AXIS2_PLACEMENT_3D('',#35540,#18625,#18626);
#15883=AXIS2_PLACEMENT_3D('',#35541,#18627,#18628);
#15884=AXIS2_PLACEMENT_3D('',#35542,#18629,#18630);
#15885=AXIS2_PLACEMENT_3D('',#35544,#18631,#18632);
#15886=AXIS2_PLACEMENT_3D('',#35545,#18633,#18634);
#15887=AXIS2_PLACEMENT_3D('',#35546,#18635,#18636);
#15888=AXIS2_PLACEMENT_3D('',#35548,#18637,#18638);
#15889=AXIS2_PLACEMENT_3D('',#35551,#18640,#18641);
#15890=AXIS2_PLACEMENT_3D('',#35552,#18642,#18643);
#15891=AXIS2_PLACEMENT_3D('',#35555,#18644,#18645);
#15892=AXIS2_PLACEMENT_3D('',#35556,#18646,#18647);
#15893=AXIS2_PLACEMENT_3D('',#35559,#18649,#18650);
#15894=AXIS2_PLACEMENT_3D('',#35560,#18651,#18652);
#15895=AXIS2_PLACEMENT_3D('',#35563,#18653,#18654);
#15896=AXIS2_PLACEMENT_3D('',#35564,#18655,#18656);
#15897=AXIS2_PLACEMENT_3D('',#35566,#18658,#18659);
#15898=AXIS2_PLACEMENT_3D('',#35569,#18660,#18661);
#15899=AXIS2_PLACEMENT_3D('',#35573,#18663,#18664);
#15900=AXIS2_PLACEMENT_3D('',#35577,#18666,#18667);
#15901=AXIS2_PLACEMENT_3D('',#35607,#18669,#18670);
#15902=AXIS2_PLACEMENT_3D('',#35611,#18672,#18673);
#15903=AXIS2_PLACEMENT_3D('',#35614,#18675,#18676);
#15904=AXIS2_PLACEMENT_3D('',#35615,#18677,#18678);
#15905=AXIS2_PLACEMENT_3D('',#35616,#18679,#18680);
#15906=AXIS2_PLACEMENT_3D('',#35618,#18681,#18682);
#15907=AXIS2_PLACEMENT_3D('',#35622,#18684,#18685);
#15908=AXIS2_PLACEMENT_3D('',#35647,#18688,#18689);
#15909=AXIS2_PLACEMENT_3D('',#35719,#18691,#18692);
#15910=AXIS2_PLACEMENT_3D('',#35729,#18694,#18695);
#15911=AXIS2_PLACEMENT_3D('',#35762,#18696,#18697);
#15912=AXIS2_PLACEMENT_3D('',#35764,#18698,#18699);
#15913=AXIS2_PLACEMENT_3D('',#35765,#18700,#18701);
#15914=AXIS2_PLACEMENT_3D('',#35766,#18702,#18703);
#15915=AXIS2_PLACEMENT_3D('',#35769,#18704,#18705);
#15916=AXIS2_PLACEMENT_3D('',#35786,#18706,#18707);
#15917=AXIS2_PLACEMENT_3D('',#35801,#18708,#18709);
#15918=AXIS2_PLACEMENT_3D('',#35804,#18710,#18711);
#15919=AXIS2_PLACEMENT_3D('',#35821,#18712,#18713);
#15920=AXIS2_PLACEMENT_3D('',#35836,#18714,#18715);
#15921=AXIS2_PLACEMENT_3D('',#35839,#18716,#18717);
#15922=AXIS2_PLACEMENT_3D('',#35843,#18719,#18720);
#15923=AXIS2_PLACEMENT_3D('',#35845,#18722,#18723);
#15924=AXIS2_PLACEMENT_3D('',#35847,#18724,#18725);
#15925=AXIS2_PLACEMENT_3D('',#36015,#18726,#18727);
#15926=AXIS2_PLACEMENT_3D('',#36058,#18728,#18729);
#15927=AXIS2_PLACEMENT_3D('',#36073,#18731,#18732);
#15928=AXIS2_PLACEMENT_3D('',#36077,#18734,#18735);
#15929=AXIS2_PLACEMENT_3D('',#36080,#18737,#18738);
#15930=AXIS2_PLACEMENT_3D('',#36081,#18739,#18740);
#15931=AXIS2_PLACEMENT_3D('',#36102,#18741,#18742);
#15932=AXIS2_PLACEMENT_3D('',#36119,#18743,#18744);
#15933=AXIS2_PLACEMENT_3D('',#36121,#18745,#18746);
#15934=AXIS2_PLACEMENT_3D('',#36134,#18747,#18748);
#15935=AXIS2_PLACEMENT_3D('',#36137,#18749,#18750);
#15936=AXIS2_PLACEMENT_3D('',#36139,#18751,#18752);
#15937=AXIS2_PLACEMENT_3D('',#36141,#18753,#18754);
#15938=AXIS2_PLACEMENT_3D('',#36142,#18755,#18756);
#15939=AXIS2_PLACEMENT_3D('',#36143,#18757,#18758);
#15940=AXIS2_PLACEMENT_3D('',#36145,#18759,#18760);
#15941=AXIS2_PLACEMENT_3D('',#36146,#18761,#18762);
#15942=AXIS2_PLACEMENT_3D('',#36147,#18763,#18764);
#15943=AXIS2_PLACEMENT_3D('',#36149,#18765,#18766);
#15944=AXIS2_PLACEMENT_3D('',#36152,#18768,#18769);
#15945=AXIS2_PLACEMENT_3D('',#36153,#18770,#18771);
#15946=AXIS2_PLACEMENT_3D('',#36155,#18772,#18773);
#15947=AXIS2_PLACEMENT_3D('',#36157,#18774,#18775);
#15948=AXIS2_PLACEMENT_3D('',#36346,#18777,#18778);
#15949=AXIS2_PLACEMENT_3D('',#36351,#18781,#18782);
#15950=AXIS2_PLACEMENT_3D('',#36353,#18784,#18785);
#15951=AXIS2_PLACEMENT_3D('',#36357,#18787,#18788);
#15952=AXIS2_PLACEMENT_3D('',#36359,#18789,#18790);
#15953=AXIS2_PLACEMENT_3D('',#36361,#18792,#18793);
#15954=AXIS2_PLACEMENT_3D('',#36363,#18794,#18795);
#15955=AXIS2_PLACEMENT_3D('',#36365,#18796,#18797);
#15956=AXIS2_PLACEMENT_3D('',#36367,#18799,#18800);
#15957=AXIS2_PLACEMENT_3D('',#36370,#18801,#18802);
#15958=AXIS2_PLACEMENT_3D('',#36390,#18803,#18804);
#15959=AXIS2_PLACEMENT_3D('',#36391,#18805,#18806);
#15960=AXIS2_PLACEMENT_3D('',#36398,#18807,#18808);
#15961=AXIS2_PLACEMENT_3D('',#36413,#18809,#18810);
#15962=AXIS2_PLACEMENT_3D('',#36416,#18811,#18812);
#15963=AXIS2_PLACEMENT_3D('',#36582,#18813,#18814);
#15964=AXIS2_PLACEMENT_3D('',#36597,#18816,#18817);
#15965=AXIS2_PLACEMENT_3D('',#36601,#18819,#18820);
#15966=AXIS2_PLACEMENT_3D('',#36605,#18822,#18823);
#15967=AXIS2_PLACEMENT_3D('',#36609,#18825,#18826);
#15968=AXIS2_PLACEMENT_3D('',#36632,#18829,#18830);
#15969=AXIS2_PLACEMENT_3D('',#36675,#18832,#18833);
#15970=AXIS2_PLACEMENT_3D('',#36677,#18834,#18835);
#15971=AXIS2_PLACEMENT_3D('',#36679,#18837,#18838);
#15972=AXIS2_PLACEMENT_3D('',#36696,#18839,#18840);
#15973=AXIS2_PLACEMENT_3D('',#36697,#18841,#18842);
#15974=AXIS2_PLACEMENT_3D('',#36698,#18843,#18844);
#15975=AXIS2_PLACEMENT_3D('',#36701,#18845,#18846);
#15976=AXIS2_PLACEMENT_3D('',#36718,#18847,#18848);
#15977=AXIS2_PLACEMENT_3D('',#36733,#18849,#18850);
#15978=AXIS2_PLACEMENT_3D('',#36736,#18851,#18852);
#15979=AXIS2_PLACEMENT_3D('',#36751,#18853,#18854);
#15980=AXIS2_PLACEMENT_3D('',#38298,#18855,#18856);
#15981=AXIS2_PLACEMENT_3D('',#38514,#18857,#18858);
#15982=AXIS2_PLACEMENT_3D('',#38960,#18859,#18860);
#15983=AXIS2_PLACEMENT_3D('',#39176,#18861,#18862);
#15984=AXIS2_PLACEMENT_3D('',#39177,#18863,#18864);
#15985=AXIS2_PLACEMENT_3D('',#39179,#18866,#18867);
#15986=AXIS2_PLACEMENT_3D('',#39181,#18869,#18870);
#15987=AXIS2_PLACEMENT_3D('',#40483,#18871,#18872);
#15988=AXIS2_PLACEMENT_3D('',#41331,#18873,#18874);
#15989=AXIS2_PLACEMENT_3D('',#41334,#18877,#18878);
#15990=AXIS2_PLACEMENT_3D('',#41340,#18882,#18883);
#15991=AXIS2_PLACEMENT_3D('',#41344,#18887,#18888);
#15992=AXIS2_PLACEMENT_3D('',#41348,#18892,#18893);
#15993=AXIS2_PLACEMENT_3D('',#41357,#18898,#18899);
#15994=AXIS2_PLACEMENT_3D('',#41366,#18904,#18905);
#15995=AXIS2_PLACEMENT_3D('',#41375,#18910,#18911);
#15996=AXIS2_PLACEMENT_3D('',#41377,#18913,#18914);
#15997=AXIS2_PLACEMENT_3D('',#41379,#18916,#18917);
#15998=AXIS2_PLACEMENT_3D('',#41381,#18919,#18920);
#15999=AXIS2_PLACEMENT_3D('',#41400,#18921,#18922);
#16000=AXIS2_PLACEMENT_3D('',#41413,#18923,#18924);
#16001=AXIS2_PLACEMENT_3D('',#41414,#18925,#18926);
#16002=AXIS2_PLACEMENT_3D('',#41431,#18928,#18929);
#16003=AXIS2_PLACEMENT_3D('',#41448,#18931,#18932);
#16004=AXIS2_PLACEMENT_3D('',#41450,#18934,#18935);
#16005=AXIS2_PLACEMENT_3D('',#41452,#18937,#18938);
#16006=AXIS2_PLACEMENT_3D('',#41469,#18939,#18940);
#16007=AXIS2_PLACEMENT_3D('',#41485,#18941,#18942);
#16008=AXIS2_PLACEMENT_3D('',#41486,#18943,#18944);
#16009=AXIS2_PLACEMENT_3D('',#41489,#18945,#18946);
#16010=AXIS2_PLACEMENT_3D('',#41491,#18947,#18948);
#16011=AXIS2_PLACEMENT_3D('',#41493,#18949,#18950);
#16012=AXIS2_PLACEMENT_3D('',#41494,#18951,#18952);
#16013=AXIS2_PLACEMENT_3D('',#41495,#18953,#18954);
#16014=AXIS2_PLACEMENT_3D('',#41498,#18957,#18958);
#16015=AXIS2_PLACEMENT_3D('',#41501,#18959,#18960);
#16016=AXIS2_PLACEMENT_3D('',#41646,#18964,#18965);
#16017=AXIS2_PLACEMENT_3D('',#41648,#18966,#18967);
#16018=AXIS2_PLACEMENT_3D('',#41649,#18968,#18969);
#16019=AXIS2_PLACEMENT_3D('',#41650,#18970,#18971);
#16020=AXIS2_PLACEMENT_3D('',#41654,#18973,#18974);
#16021=AXIS2_PLACEMENT_3D('',#41954,#18976,#18977);
#16022=AXIS2_PLACEMENT_3D('',#41955,#18978,#18979);
#16023=AXIS2_PLACEMENT_3D('',#41959,#18982,#18983);
#16024=AXIS2_PLACEMENT_3D('',#41967,#18989,#18990);
#16025=AXIS2_PLACEMENT_3D('',#41969,#18992,#18993);
#16026=AXIS2_PLACEMENT_3D('',#41996,#18994,#18995);
#16027=AXIS2_PLACEMENT_3D('',#41997,#18996,#18997);
#16028=AXIS2_PLACEMENT_3D('',#41999,#18998,#18999);
#16029=AXIS2_PLACEMENT_3D('',#42002,#19001,#19002);
#16030=AXIS2_PLACEMENT_3D('',#42004,#19004,#19005);
#16031=AXIS2_PLACEMENT_3D('',#42006,#19007,#19008);
#16032=AXIS2_PLACEMENT_3D('',#42008,#19010,#19011);
#16033=AXIS2_PLACEMENT_3D('',#42012,#19014,#19015);
#16034=AXIS2_PLACEMENT_3D('',#42014,#19016,#19017);
#16035=AXIS2_PLACEMENT_3D('',#42016,#19018,#19019);
#16036=AXIS2_PLACEMENT_3D('',#42031,#19020,#19021);
#16037=AXIS2_PLACEMENT_3D('',#42034,#19023,#19024);
#16038=AXIS2_PLACEMENT_3D('',#42407,#19025,#19026);
#16039=AXIS2_PLACEMENT_3D('',#42408,#19027,#19028);
#16040=AXIS2_PLACEMENT_3D('',#42409,#19029,#19030);
#16041=AXIS2_PLACEMENT_3D('',#42411,#19032,#19033);
#16042=AXIS2_PLACEMENT_3D('',#42413,#19034,#19035);
#16043=AXIS2_PLACEMENT_3D('',#42561,#19037,#19038);
#16044=AXIS2_PLACEMENT_3D('',#42562,#19039,#19040);
#16045=AXIS2_PLACEMENT_3D('',#42682,#19042,#19043);
#16046=AXIS2_PLACEMENT_3D('',#42683,#19044,#19045);
#16047=AXIS2_PLACEMENT_3D('',#42684,#19046,#19047);
#16048=AXIS2_PLACEMENT_3D('',#42864,#19048,#19049);
#16049=AXIS2_PLACEMENT_3D('',#42865,#19050,#19051);
#16050=AXIS2_PLACEMENT_3D('',#42866,#19052,#19053);
#16051=AXIS2_PLACEMENT_3D('',#42867,#19054,#19055);
#16052=AXIS2_PLACEMENT_3D('',#42969,#19056,#19057);
#16053=AXIS2_PLACEMENT_3D('',#42970,#19058,#19059);
#16054=AXIS2_PLACEMENT_3D('',#42971,#19060,#19061);
#16055=AXIS2_PLACEMENT_3D('',#42987,#19062,#19063);
#16056=AXIS2_PLACEMENT_3D('',#42988,#19064,#19065);
#16057=AXIS2_PLACEMENT_3D('',#43115,#19066,#19067);
#16058=AXIS2_PLACEMENT_3D('',#43118,#19069,#19070);
#16059=AXIS2_PLACEMENT_3D('',#43119,#19071,#19072);
#16060=AXIS2_PLACEMENT_3D('',#43121,#19073,#19074);
#16061=AXIS2_PLACEMENT_3D('',#43133,#19075,#19076);
#16062=AXIS2_PLACEMENT_3D('',#43134,#19077,#19078);
#16063=AXIS2_PLACEMENT_3D('',#43138,#19080,#19081);
#16064=AXIS2_PLACEMENT_3D('',#43141,#19083,#19084);
#16065=AXIS2_PLACEMENT_3D('',#43142,#19085,#19086);
#16066=AXIS2_PLACEMENT_3D('',#43177,#19090,#19091);
#16067=AXIS2_PLACEMENT_3D('',#43179,#19092,#19093);
#16068=AXIS2_PLACEMENT_3D('',#43180,#19094,#19095);
#16069=AXIS2_PLACEMENT_3D('',#43181,#19096,#19097);
#16070=AXIS2_PLACEMENT_3D('',#43182,#19098,#19099);
#16071=AXIS2_PLACEMENT_3D('',#43183,#19100,#19101);
#16072=AXIS2_PLACEMENT_3D('',#43184,#19102,#19103);
#16073=AXIS2_PLACEMENT_3D('',#43188,#19105,#19106);
#16074=AXIS2_PLACEMENT_3D('',#43189,#19107,#19108);
#16075=AXIS2_PLACEMENT_3D('',#43190,#19109,#19110);
#16076=AXIS2_PLACEMENT_3D('',#43193,#19112,#19113);
#16077=AXIS2_PLACEMENT_3D('',#43194,#19114,#19115);
#16078=AXIS2_PLACEMENT_3D('',#43198,#19118,#19119);
#16079=AXIS2_PLACEMENT_3D('',#43200,#19121,#19122);
#16080=AXIS2_PLACEMENT_3D('',#43208,#19127,#19128);
#16081=AXIS2_PLACEMENT_3D('',#43227,#19135,#19136);
#16082=AXIS2_PLACEMENT_3D('',#43229,#19137,#19138);
#16083=AXIS2_PLACEMENT_3D('',#43296,#19140,#19141);
#16084=AXIS2_PLACEMENT_3D('',#43362,#19142,#19143);
#16085=AXIS2_PLACEMENT_3D('',#43363,#19144,#19145);
#16086=AXIS2_PLACEMENT_3D('',#43395,#19147,#19148);
#16087=AXIS2_PLACEMENT_3D('',#43397,#19149,#19150);
#16088=AXIS2_PLACEMENT_3D('',#43398,#19151,#19152);
#16089=AXIS2_PLACEMENT_3D('',#43399,#19153,#19154);
#16090=AXIS2_PLACEMENT_3D('',#43401,#19155,#19156);
#16091=AXIS2_PLACEMENT_3D('',#43402,#19157,#19158);
#16092=AXIS2_PLACEMENT_3D('',#43403,#19159,#19160);
#16093=AXIS2_PLACEMENT_3D('',#43730,#19162,#19163);
#16094=AXIS2_PLACEMENT_3D('',#43732,#19164,#19165);
#16095=AXIS2_PLACEMENT_3D('',#43743,#19166,#19167);
#16096=AXIS2_PLACEMENT_3D('',#43744,#19168,#19169);
#16097=AXIS2_PLACEMENT_3D('',#43745,#19170,#19171);
#16098=AXIS2_PLACEMENT_3D('',#43746,#19172,#19173);
#16099=AXIS2_PLACEMENT_3D('',#43747,#19174,#19175);
#16100=AXIS2_PLACEMENT_3D('',#43748,#19176,#19177);
#16101=AXIS2_PLACEMENT_3D('',#43749,#19178,#19179);
#16102=AXIS2_PLACEMENT_3D('',#43751,#19181,#19182);
#16103=AXIS2_PLACEMENT_3D('',#43755,#19184,#19185);
#16104=AXIS2_PLACEMENT_3D('',#43761,#19188,#19189);
#16105=AXIS2_PLACEMENT_3D('',#43764,#19191,#19192);
#16106=AXIS2_PLACEMENT_3D('',#43765,#19193,#19194);
#16107=AXIS2_PLACEMENT_3D('',#43766,#19195,#19196);
#16108=AXIS2_PLACEMENT_3D('',#43767,#19197,#19198);
#16109=AXIS2_PLACEMENT_3D('',#43768,#19199,#19200);
#16110=AXIS2_PLACEMENT_3D('',#43780,#19202,#19203);
#16111=AXIS2_PLACEMENT_3D('',#43781,#19204,#19205);
#16112=AXIS2_PLACEMENT_3D('',#43782,#19206,#19207);
#16113=AXIS2_PLACEMENT_3D('',#43783,#19208,#19209);
#16114=AXIS2_PLACEMENT_3D('',#43785,#19210,#19211);
#16115=AXIS2_PLACEMENT_3D('',#43788,#19213,#19214);
#16116=AXIS2_PLACEMENT_3D('',#43789,#19215,#19216);
#16117=AXIS2_PLACEMENT_3D('',#43792,#19218,#19219);
#16118=AXIS2_PLACEMENT_3D('',#43795,#19221,#19222);
#16119=AXIS2_PLACEMENT_3D('',#43796,#19223,#19224);
#16120=AXIS2_PLACEMENT_3D('',#43801,#19226,#19227);
#16121=AXIS2_PLACEMENT_3D('',#43804,#19229,#19230);
#16122=AXIS2_PLACEMENT_3D('',#43805,#19231,#19232);
#16123=AXIS2_PLACEMENT_3D('',#43809,#19234,#19235);
#16124=AXIS2_PLACEMENT_3D('',#43811,#19237,#19238);
#16125=AXIS2_PLACEMENT_3D('',#43816,#19242,#19243);
#16126=AXIS2_PLACEMENT_3D('',#43817,#19244,#19245);
#16127=AXIS2_PLACEMENT_3D('',#43818,#19246,#19247);
#16128=AXIS2_PLACEMENT_3D('',#43819,#19248,#19249);
#16129=AXIS2_PLACEMENT_3D('',#43820,#19250,#19251);
#16130=AXIS2_PLACEMENT_3D('',#43821,#19252,#19253);
#16131=AXIS2_PLACEMENT_3D('',#43822,#19254,#19255);
#16132=AXIS2_PLACEMENT_3D('',#43823,#19256,#19257);
#16133=AXIS2_PLACEMENT_3D('',#43844,#19258,#19259);
#16134=AXIS2_PLACEMENT_3D('',#43845,#19260,#19261);
#16135=AXIS2_PLACEMENT_3D('',#43874,#19262,#19263);
#16136=AXIS2_PLACEMENT_3D('',#43875,#19264,#19265);
#16137=AXIS2_PLACEMENT_3D('',#43890,#19266,#19267);
#16138=AXIS2_PLACEMENT_3D('',#43891,#19268,#19269);
#16139=AXIS2_PLACEMENT_3D('',#43906,#19270,#19271);
#16140=AXIS2_PLACEMENT_3D('',#43913,#19272,#19273);
#16141=AXIS2_PLACEMENT_3D('',#43915,#19275,#19276);
#16142=AXIS2_PLACEMENT_3D('',#43916,#19277,#19278);
#16143=AXIS2_PLACEMENT_3D('',#43917,#19279,#19280);
#16144=AXIS2_PLACEMENT_3D('',#43935,#19281,#19282);
#16145=AXIS2_PLACEMENT_3D('',#43937,#19284,#19285);
#16146=AXIS2_PLACEMENT_3D('',#43938,#19286,#19287);
#16147=AXIS2_PLACEMENT_3D('',#43975,#19288,#19289);
#16148=AXIS2_PLACEMENT_3D('',#43980,#19292,#19293);
#16149=AXIS2_PLACEMENT_3D('',#43981,#19294,#19295);
#16150=AXIS2_PLACEMENT_3D('',#43982,#19296,#19297);
#16151=AXIS2_PLACEMENT_3D('',#43983,#19298,#19299);
#16152=AXIS2_PLACEMENT_3D('',#43984,#19300,#19301);
#16153=AXIS2_PLACEMENT_3D('',#44213,#19302,#19303);
#16154=AXIS2_PLACEMENT_3D('',#44214,#19304,#19305);
#16155=AXIS2_PLACEMENT_3D('',#44217,#19308,#19309);
#16156=AXIS2_PLACEMENT_3D('',#44218,#19310,#19311);
#16157=AXIS2_PLACEMENT_3D('',#44247,#19312,#19313);
#16158=AXIS2_PLACEMENT_3D('',#44360,#19314,#19315);
#16159=AXIS2_PLACEMENT_3D('',#44361,#19316,#19317);
#16160=AXIS2_PLACEMENT_3D('',#44362,#19318,#19319);
#16161=AXIS2_PLACEMENT_3D('',#44391,#19320,#19321);
#16162=AXIS2_PLACEMENT_3D('',#44392,#19322,#19323);
#16163=AXIS2_PLACEMENT_3D('',#44393,#19324,#19325);
#16164=AXIS2_PLACEMENT_3D('',#44408,#19326,#19327);
#16165=AXIS2_PLACEMENT_3D('',#44421,#19328,#19329);
#16166=AXIS2_PLACEMENT_3D('',#44422,#19330,#19331);
#16167=AXIS2_PLACEMENT_3D('',#44423,#19332,#19333);
#16168=AXIS2_PLACEMENT_3D('',#44424,#19334,#19335);
#16169=AXIS2_PLACEMENT_3D('',#44425,#19336,#19337);
#16170=AXIS2_PLACEMENT_3D('',#44429,#19340,#19341);
#16171=AXIS2_PLACEMENT_3D('',#44431,#19343,#19344);
#16172=AXIS2_PLACEMENT_3D('',#44432,#19345,#19346);
#16173=AXIS2_PLACEMENT_3D('',#44433,#19347,#19348);
#16174=AXIS2_PLACEMENT_3D('',#44434,#19349,#19350);
#16175=AXIS2_PLACEMENT_3D('',#44435,#19351,#19352);
#18577=DIRECTION('axis',(0.,0.,1.));
#18578=DIRECTION('refdir',(1.,0.,0.));
#18579=DIRECTION('center_axis',(1.,-6.12303176911189E-17,0.));
#18580=DIRECTION('ref_axis',(0.,1.,0.));
#18581=DIRECTION('center_axis',(-1.0241047919602E-18,-0.0167254528569715,
0.999860119830134));
#18582=DIRECTION('ref_axis',(1.,-1.71286164185289E-20,1.02396154000794E-18));
#18583=DIRECTION('center_axis',(-1.0241047919602E-18,-0.0167254528569715,
0.999860119830134));
#18584=DIRECTION('ref_axis',(1.,-1.71286164185289E-20,1.02396154000794E-18));
#18585=DIRECTION('center_axis',(-1.,6.12303176911189E-17,0.));
#18586=DIRECTION('ref_axis',(6.12303176911189E-17,1.,0.));
#18587=DIRECTION('center_axis',(0.,0.,-1.));
#18588=DIRECTION('ref_axis',(1.,0.,0.));
#18589=DIRECTION('center_axis',(0.,0.,-1.));
#18590=DIRECTION('ref_axis',(1.,0.,0.));
#18591=DIRECTION('center_axis',(0.,0.,-1.));
#18592=DIRECTION('ref_axis',(1.,0.,0.));
#18593=DIRECTION('center_axis',(0.,0.,-1.));
#18594=DIRECTION('ref_axis',(1.,0.,0.));
#18595=DIRECTION('center_axis',(1.,-6.12303176911189E-17,0.));
#18596=DIRECTION('ref_axis',(0.,1.,0.));
#18597=DIRECTION('center_axis',(-3.05385885637485E-31,2.44929359829471E-15,
-1.));
#18598=DIRECTION('ref_axis',(1.,7.47979694701453E-46,-3.05385885637485E-31));
#18599=DIRECTION('center_axis',(-3.05385885637485E-31,2.44929359829471E-15,
-1.));
#18600=DIRECTION('ref_axis',(1.,7.47979694701453E-46,-3.05385885637485E-31));
#18601=DIRECTION('center_axis',(-3.05385885637485E-31,2.44929359829471E-15,
-1.));
#18602=DIRECTION('ref_axis',(1.,7.47979694701453E-46,-3.05385885637485E-31));
#18603=DIRECTION('center_axis',(-3.05385885637485E-31,2.44929359829471E-15,
-1.));
#18604=DIRECTION('ref_axis',(1.,7.47979694701453E-46,-3.05385885637485E-31));
#18605=DIRECTION('center_axis',(-1.,6.12303176911189E-17,0.));
#18606=DIRECTION('ref_axis',(6.12303176911189E-17,1.,0.));
#18607=DIRECTION('center_axis',(2.02350164340122E-18,0.0330473810965473,
0.999453786126532));
#18608=DIRECTION('ref_axis',(1.,-6.68714299589699E-20,-2.02239637873061E-18));
#18609=DIRECTION('center_axis',(2.02350164340122E-18,0.0330473810965473,
0.999453786126532));
#18610=DIRECTION('ref_axis',(1.,-6.68714299589699E-20,-2.02239637873061E-18));
#18611=DIRECTION('center_axis',(-1.,6.12303176911189E-17,0.));
#18612=DIRECTION('ref_axis',(0.,-1.,0.));
#18613=DIRECTION('center_axis',(1.,-6.12303176911189E-17,0.));
#18614=DIRECTION('ref_axis',(-6.12303176911189E-17,-1.,0.));
#18615=DIRECTION('center_axis',(2.97215916777767E-17,0.485406458736823,
0.874288607850163));
#18616=DIRECTION('ref_axis',(1.,-1.44270525643314E-17,-2.59852490110544E-17));
#18617=DIRECTION('center_axis',(-1.,6.12303176911189E-17,0.));
#18618=DIRECTION('ref_axis',(0.,-1.,0.));
#18619=DIRECTION('center_axis',(-1.18600730662684E-17,-0.193696089020763,
0.981061580685973));
#18620=DIRECTION('ref_axis',(1.,-2.29724976843668E-18,1.16354620294444E-17));
#18621=DIRECTION('center_axis',(1.,-6.12303176911189E-17,0.));
#18622=DIRECTION('ref_axis',(-6.12303176911189E-17,-1.,0.));
#18623=DIRECTION('center_axis',(-1.,6.12303176911189E-17,0.));
#18624=DIRECTION('ref_axis',(0.,0.970124980364195,-0.242605693406751));
#18625=DIRECTION('center_axis',(2.97215916777766E-17,0.485406458736823,
0.874288607850164));
#18626=DIRECTION('ref_axis',(1.,-1.44270525643314E-17,-2.59852490110543E-17));
#18627=DIRECTION('center_axis',(1.,-6.12303176911189E-17,0.));
#18628=DIRECTION('ref_axis',(5.94010607477901E-17,0.970124980364195,-0.242605693406751));
#18629=DIRECTION('center_axis',(-1.,6.12303176911189E-17,0.));
#18630=DIRECTION('ref_axis',(0.,0.996726356556968,0.0808490577846839));
#18631=DIRECTION('center_axis',(1.,-6.12303176911189E-17,0.));
#18632=DIRECTION('ref_axis',(6.10298714630946E-17,0.996726356556968,0.0808490577846839));
#18633=DIRECTION('center_axis',(-1.18600730662684E-17,-0.193696089020763,
0.981061580685973));
#18634=DIRECTION('ref_axis',(1.,-2.29724976843668E-18,1.16354620294444E-17));
#18635=DIRECTION('center_axis',(1.,0.,0.));
#18636=DIRECTION('ref_axis',(0.,0.,-1.));
#18637=DIRECTION('center_axis',(1.,-6.12303176911189E-17,0.));
#18638=DIRECTION('ref_axis',(-6.12303176911189E-17,-1.,0.));
#18639=DIRECTION('',(-1.,0.,0.));
#18640=DIRECTION('center_axis',(1.,-6.12303176911189E-17,0.));
#18641=DIRECTION('ref_axis',(6.12303176911189E-17,1.,0.));
#18642=DIRECTION('center_axis',(1.,0.,0.));
#18643=DIRECTION('ref_axis',(0.,0.,1.));
#18644=DIRECTION('center_axis',(1.,0.,0.));
#18645=DIRECTION('ref_axis',(0.,0.,1.));
#18646=DIRECTION('center_axis',(1.,0.,0.));
#18647=DIRECTION('ref_axis',(0.,0.,1.));
#18648=DIRECTION('',(-0.707106781186548,-8.65956056235493E-17,0.707106781186547));
#18649=DIRECTION('center_axis',(-1.,6.12303176911189E-17,0.));
#18650=DIRECTION('ref_axis',(6.12303176911189E-17,1.,0.));
#18651=DIRECTION('center_axis',(1.,0.,0.));
#18652=DIRECTION('ref_axis',(0.,0.,-1.));
#18653=DIRECTION('center_axis',(-1.,6.12303176911189E-17,0.));
#18654=DIRECTION('ref_axis',(6.12303176911189E-17,1.,0.));
#18655=DIRECTION('center_axis',(-1.,6.12303176911189E-17,0.));
#18656=DIRECTION('ref_axis',(6.12303176911189E-17,1.,0.));
#18657=DIRECTION('',(-1.,0.,0.));
#18658=DIRECTION('center_axis',(-1.,6.12303176911189E-17,0.));
#18659=DIRECTION('ref_axis',(6.12303176911189E-17,1.,0.));
#18660=DIRECTION('center_axis',(1.,-6.12303176911189E-17,0.));
#18661=DIRECTION('ref_axis',(6.12303176911189E-17,1.,0.));
#18662=DIRECTION('',(-1.,6.12303176911189E-17,0.));
#18663=DIRECTION('center_axis',(-1.,6.12303176911189E-17,0.));
#18664=DIRECTION('ref_axis',(6.12303176911189E-17,1.,0.));
#18665=DIRECTION('',(-1.,3.93558242098606E-17,0.));
#18666=DIRECTION('center_axis',(1.,0.,0.));
#18667=DIRECTION('ref_axis',(0.,0.,-1.));
#18668=DIRECTION('',(1.,0.,0.));
#18669=DIRECTION('center_axis',(-1.,0.,0.));
#18670=DIRECTION('ref_axis',(0.,0.,1.));
#18671=DIRECTION('',(1.,-6.12303176911189E-17,0.));
#18672=DIRECTION('center_axis',(-1.,3.78429896776521E-17,0.));
#18673=DIRECTION('ref_axis',(-3.78429896776521E-17,-1.,0.));
#18674=DIRECTION('',(-1.,3.93558242098606E-17,0.));
#18675=DIRECTION('center_axis',(-1.,6.12303176911189E-17,0.));
#18676=DIRECTION('ref_axis',(6.12303176911189E-17,1.,0.));
#18677=DIRECTION('center_axis',(1.,-6.12303176911189E-17,0.));
#18678=DIRECTION('ref_axis',(6.12303176911189E-17,1.,0.));
#18679=DIRECTION('center_axis',(1.,-6.12303176911189E-17,0.));
#18680=DIRECTION('ref_axis',(-6.12303176911189E-17,-1.,0.));
#18681=DIRECTION('center_axis',(-1.,6.12303176911189E-17,0.));
#18682=DIRECTION('ref_axis',(-6.12303176911189E-17,-1.,0.));
#18683=DIRECTION('',(-1.,6.12303176911189E-17,0.));
#18684=DIRECTION('center_axis',(1.,-6.12303176911189E-17,0.));
#18685=DIRECTION('ref_axis',(6.12303176911189E-17,1.,0.));
#18686=DIRECTION('',(1.,-6.12303176911189E-17,0.));
#18687=DIRECTION('',(-1.,6.12303176911189E-17,0.));
#18688=DIRECTION('center_axis',(1.,-6.12303176911189E-17,0.));
#18689=DIRECTION('ref_axis',(6.12303176911189E-17,1.,0.));
#18690=DIRECTION('',(-1.,6.12303176911189E-17,0.));
#18691=DIRECTION('center_axis',(-1.,0.,0.));
#18692=DIRECTION('ref_axis',(0.,0.,-1.));
#18693=DIRECTION('',(-1.,6.12303176911189E-17,0.));
#18694=DIRECTION('center_axis',(1.,-6.12303176911189E-17,0.));
#18695=DIRECTION('ref_axis',(6.12303176911189E-17,1.,0.));
#18696=DIRECTION('center_axis',(1.,-6.12303176911189E-17,0.));
#18697=DIRECTION('ref_axis',(0.,1.,0.));
#18698=DIRECTION('center_axis',(1.,-6.12303176911189E-17,0.));
#18699=DIRECTION('ref_axis',(6.12303176911189E-17,1.,0.));
#18700=DIRECTION('center_axis',(7.49855125668918E-33,1.22464679907692E-16,
-1.));
#18701=DIRECTION('ref_axis',(0.,-1.,-1.22464679907692E-16));
#18702=DIRECTION('center_axis',(1.,-6.305873043676E-17,0.));
#18703=DIRECTION('ref_axis',(0.,1.,0.));
#18704=DIRECTION('center_axis',(1.,-6.305873043676E-17,0.));
#18705=DIRECTION('ref_axis',(6.305873043676E-17,1.,0.));
#18706=DIRECTION('center_axis',(-1.,6.305873043676E-17,0.));
#18707=DIRECTION('ref_axis',(6.305873043676E-17,1.,0.));
#18708=DIRECTION('center_axis',(1.,-6.305873043676E-17,0.));
#18709=DIRECTION('ref_axis',(0.,1.,0.));
#18710=DIRECTION('center_axis',(1.,-6.305873043676E-17,0.));
#18711=DIRECTION('ref_axis',(6.305873043676E-17,1.,0.));
#18712=DIRECTION('center_axis',(-1.,6.305873043676E-17,0.));
#18713=DIRECTION('ref_axis',(6.305873043676E-17,1.,0.));
#18714=DIRECTION('center_axis',(-1.,0.,0.));
#18715=DIRECTION('ref_axis',(0.,0.,1.));
#18716=DIRECTION('center_axis',(-1.,0.,0.));
#18717=DIRECTION('ref_axis',(0.,0.,-1.));
#18718=DIRECTION('',(-1.,0.,0.));
#18719=DIRECTION('center_axis',(1.,-6.12303176911189E-17,0.));
#18720=DIRECTION('ref_axis',(6.12303176911189E-17,1.,0.));
#18721=DIRECTION('',(1.,0.,0.));
#18722=DIRECTION('center_axis',(-1.,0.,0.));
#18723=DIRECTION('ref_axis',(0.,0.,1.));
#18724=DIRECTION('center_axis',(-1.,6.12303176911189E-17,0.));
#18725=DIRECTION('ref_axis',(6.12303176911189E-17,1.,0.));
#18726=DIRECTION('center_axis',(-1.,6.12303176911189E-17,0.));
#18727=DIRECTION('ref_axis',(6.12303176911189E-17,1.,0.));
#18728=DIRECTION('center_axis',(-0.707106781186543,-8.6003326957104E-14,
-0.707106781186552));
#18729=DIRECTION('ref_axis',(0.707106781186552,1.48735968909061E-10,-0.707106781186543));
#18730=DIRECTION('',(-1.,0.,0.));
#18731=DIRECTION('center_axis',(-1.,8.82754440022857E-17,0.));
#18732=DIRECTION('ref_axis',(-8.82754440022857E-17,-1.,0.));
#18733=DIRECTION('',(1.,0.,0.));
#18734=DIRECTION('center_axis',(1.,-6.12303176911189E-17,0.));
#18735=DIRECTION('ref_axis',(-6.12303176911189E-17,-1.,0.));
#18736=DIRECTION('',(-1.,6.12303176911189E-17,0.));
#18737=DIRECTION('center_axis',(-1.,0.,0.));
#18738=DIRECTION('ref_axis',(0.,0.,-1.));
#18739=DIRECTION('center_axis',(1.,-6.12303176911189E-17,0.));
#18740=DIRECTION('ref_axis',(0.,-0.933406972407284,0.358819486457282));
#18741=DIRECTION('center_axis',(1.,-6.12303176911189E-17,0.));
#18742=DIRECTION('ref_axis',(6.12303176911189E-17,1.,0.));
#18743=DIRECTION('center_axis',(1.,-6.12303176911189E-17,0.));
#18744=DIRECTION('ref_axis',(6.12303176911189E-17,1.,0.));
#18745=DIRECTION('center_axis',(1.,-6.12303176911189E-17,0.));
#18746=DIRECTION('ref_axis',(6.12303176911189E-17,1.,0.));
#18747=DIRECTION('center_axis',(0.,0.,-1.));
#18748=DIRECTION('ref_axis',(1.,0.,0.));
#18749=DIRECTION('center_axis',(0.,0.,1.));
#18750=DIRECTION('ref_axis',(1.,0.,0.));
#18751=DIRECTION('center_axis',(-1.,0.,0.));
#18752=DIRECTION('ref_axis',(0.,0.,-1.));
#18753=DIRECTION('center_axis',(0.,0.,-1.));
#18754=DIRECTION('ref_axis',(1.,0.,0.));
#18755=DIRECTION('center_axis',(1.,0.,0.));
#18756=DIRECTION('ref_axis',(0.,0.,1.));
#18757=DIRECTION('center_axis',(-1.,6.12303176911189E-17,0.));
#18758=DIRECTION('ref_axis',(0.,-1.,0.));
#18759=DIRECTION('center_axis',(-1.35958617011586E-32,-2.22044604925031E-16,
-1.));
#18760=DIRECTION('ref_axis',(0.,1.,-2.22044604925031E-16));
#18761=DIRECTION('center_axis',(1.,-6.12303176911189E-17,0.));
#18762=DIRECTION('ref_axis',(-6.12303176911189E-17,-1.,0.));
#18763=DIRECTION('center_axis',(0.,0.,-1.));
#18764=DIRECTION('ref_axis',(-1.,0.,0.));
#18765=DIRECTION('center_axis',(0.,0.,-1.));
#18766=DIRECTION('ref_axis',(1.,0.,0.));
#18767=DIRECTION('',(0.,0.,-1.));
#18768=DIRECTION('center_axis',(0.,0.,-1.));
#18769=DIRECTION('ref_axis',(-1.,0.,0.));
#18770=DIRECTION('center_axis',(1.,-6.12303176911189E-17,0.));
#18771=DIRECTION('ref_axis',(1.24734901031854E-17,0.20371428033591,-0.979030383587364));
#18772=DIRECTION('center_axis',(1.,0.,0.));
#18773=DIRECTION('ref_axis',(0.,0.,1.));
#18774=DIRECTION('center_axis',(1.,-6.37765983815004E-17,0.));
#18775=DIRECTION('ref_axis',(-6.37765983815004E-17,-1.,0.));
#18776=DIRECTION('',(-1.,6.12303176911189E-17,0.));
#18777=DIRECTION('center_axis',(-1.,6.305873043676E-17,0.));
#18778=DIRECTION('ref_axis',(6.305873043676E-17,1.,0.));
#18779=DIRECTION('',(-1.,3.93558242098606E-17,0.));
#18780=DIRECTION('',(-1.,3.93558242098606E-17,0.));
#18781=DIRECTION('center_axis',(-1.,0.,0.));
#18782=DIRECTION('ref_axis',(0.,0.,-1.));
#18783=DIRECTION('',(-1.,6.12303176911189E-17,0.));
#18784=DIRECTION('center_axis',(-0.707106781186548,-3.48206089692902E-16,
0.707106781186548));
#18785=DIRECTION('ref_axis',(0.707106781186547,7.42019951680791E-31,0.707106781186547));
#18786=DIRECTION('',(0.707106781186547,3.48206089692903E-16,-0.707106781186547));
#18787=DIRECTION('center_axis',(-0.707106781186547,-6.13317366673352E-16,
0.707106781186548));
#18788=DIRECTION('ref_axis',(-0.707106781186548,-1.21863909340796E-30,-0.707106781186547));
#18789=DIRECTION('center_axis',(-0.707106781186548,-6.13317366673348E-16,
0.707106781186548));
#18790=DIRECTION('ref_axis',(-0.707106781186548,-1.52186717178597E-30,-0.707106781186548));
#18791=DIRECTION('',(-0.707106781186547,-3.48206089692903E-16,0.707106781186547));
#18792=DIRECTION('center_axis',(-1.,6.12303176911189E-17,0.));
#18793=DIRECTION('ref_axis',(6.12303176911189E-17,1.,0.));
#18794=DIRECTION('center_axis',(1.,0.,0.));
#18795=DIRECTION('ref_axis',(0.,0.,1.));
#18796=DIRECTION('center_axis',(-1.,6.12303176911189E-17,0.));
#18797=DIRECTION('ref_axis',(6.12303176911189E-17,1.,0.));
#18798=DIRECTION('',(-1.,6.12303176911189E-17,0.));
#18799=DIRECTION('center_axis',(1.,-6.12303176911189E-17,0.));
#18800=DIRECTION('ref_axis',(0.,0.0945993501281125,0.995515425774678));
#18801=DIRECTION('center_axis',(-1.,6.12303176911189E-17,0.));
#18802=DIRECTION('ref_axis',(6.12303176911189E-17,1.,0.));
#18803=DIRECTION('center_axis',(0.,-0.206307963004919,-0.978487109981915));
#18804=DIRECTION('ref_axis',(0.,-0.978487109981915,0.206307963004919));
#18805=DIRECTION('center_axis',(1.,-6.12303176911189E-17,0.));
#18806=DIRECTION('ref_axis',(0.,1.,0.));
#18807=DIRECTION('center_axis',(-1.,6.12303176911189E-17,0.));
#18808=DIRECTION('ref_axis',(6.12303176911189E-17,1.,0.));
#18809=DIRECTION('center_axis',(1.,-8.55850097257312E-17,0.));
#18810=DIRECTION('ref_axis',(8.29584272353424E-17,0.969310250722573,-0.245840675731543));
#18811=DIRECTION('center_axis',(1.,-6.12303176911189E-17,0.));
#18812=DIRECTION('ref_axis',(6.12303176911189E-17,1.,0.));
#18813=DIRECTION('center_axis',(1.,-6.12303176911189E-17,0.));
#18814=DIRECTION('ref_axis',(6.12303176911189E-17,1.,0.));
#18815=DIRECTION('',(-1.,8.55850097257312E-17,0.));
#18816=DIRECTION('center_axis',(1.,0.,0.));
#18817=DIRECTION('ref_axis',(0.,0.,-1.));
#18818=DIRECTION('',(-1.,0.,0.));
#18819=DIRECTION('center_axis',(-1.,8.82766640598215E-17,0.));
#18820=DIRECTION('ref_axis',(-8.82766640598215E-17,-1.,0.));
#18821=DIRECTION('',(1.,-8.55850097257312E-17,0.));
#18822=DIRECTION('center_axis',(1.,0.,0.));
#18823=DIRECTION('ref_axis',(0.,0.,-1.));
#18824=DIRECTION('',(-1.,8.55850097257312E-17,0.));
#18825=DIRECTION('center_axis',(1.,-6.12303176911189E-17,0.));
#18826=DIRECTION('ref_axis',(6.12303176911189E-17,1.,0.));
#18827=DIRECTION('',(1.,-8.55850097257312E-17,0.));
#18828=DIRECTION('',(1.,-8.55850097257312E-17,0.));
#18829=DIRECTION('center_axis',(-0.894427190999916,0.420243315606445,-0.152956058030083));
#18830=DIRECTION('ref_axis',(0.425247203315731,0.90507724315229,5.35984724282349E-16));
#18831=DIRECTION('',(0.894427190999916,-0.420243315606445,0.152956058030083));
#18832=DIRECTION('center_axis',(0.948683298050566,0.297156898213485,-0.108156265856593));
#18833=DIRECTION('ref_axis',(0.316227766016682,-0.89147069465054,0.324468797543589));
#18834=DIRECTION('center_axis',(0.948683298050506,0.297156898213675,-0.108156265856598));
#18835=DIRECTION('ref_axis',(0.316227766016862,-0.89147069464147,0.324468797568334));
#18836=DIRECTION('',(-0.894427190999916,0.420243315606445,-0.152956058030083));
#18837=DIRECTION('center_axis',(1.,-6.12303176911189E-17,0.));
#18838=DIRECTION('ref_axis',(0.,1.,0.));
#18839=DIRECTION('center_axis',(-1.,6.12303176911189E-17,0.));
#18840=DIRECTION('ref_axis',(6.12303176911189E-17,1.,0.));
#18841=DIRECTION('center_axis',(0.,-0.301227558036465,0.953552283977857));
#18842=DIRECTION('ref_axis',(0.,0.953552283977857,0.301227558036465));
#18843=DIRECTION('center_axis',(1.,-6.12303176911189E-17,0.));
#18844=DIRECTION('ref_axis',(0.,1.,0.));
#18845=DIRECTION('center_axis',(-1.,6.12303176911189E-17,0.));
#18846=DIRECTION('ref_axis',(6.12303176911189E-17,1.,0.));
#18847=DIRECTION('center_axis',(1.,-6.12303176911189E-17,0.));
#18848=DIRECTION('ref_axis',(6.12303176911189E-17,1.,0.));
#18849=DIRECTION('center_axis',(1.,-6.12303176911189E-17,0.));
#18850=DIRECTION('ref_axis',(0.,1.,0.));
#18851=DIRECTION('center_axis',(-1.,6.12303176911189E-17,0.));
#18852=DIRECTION('ref_axis',(6.12303176911189E-17,1.,0.));
#18853=DIRECTION('center_axis',(1.,-6.12303176911189E-17,0.));
#18854=DIRECTION('ref_axis',(6.12303176911189E-17,1.,0.));
#18855=DIRECTION('center_axis',(0.191261891041587,-0.962950243082436,-0.190120273465704));
#18856=DIRECTION('ref_axis',(-6.86713994557681E-6,0.193694776232803,-0.98106183985158));
#18857=DIRECTION('center_axis',(-0.191881081657469,0.962831674217306,0.190096863798062));
#18858=DIRECTION('ref_axis',(3.99680288865059E-14,0.193696089020735,-0.981061580685979));
#18859=DIRECTION('center_axis',(0.00786589508707537,0.999969063368702,-1.88252157794132E-14));
#18860=DIRECTION('ref_axis',(-3.94970882666714E-7,3.10691472549253E-9,0.999999999999922));
#18861=DIRECTION('center_axis',(-0.00663612315024062,-0.999977980692342,
1.83917848476882E-13));
#18862=DIRECTION('ref_axis',(4.13457446057927E-8,-2.74198441729828E-10,
0.999999999999999));
#18863=DIRECTION('center_axis',(2.97215916777767E-17,0.485406458736824,
0.874288607850163));
#18864=DIRECTION('ref_axis',(1.08239046981355E-32,0.874288607850163,-0.485406458736824));
#18865=DIRECTION('',(-2.97215916777767E-17,-0.485406458736824,-0.874288607850163));
#18866=DIRECTION('center_axis',(-1.18600730662684E-17,-0.19369608902076,
0.981061580685974));
#18867=DIRECTION('ref_axis',(-2.11938170784821E-33,0.981061580685974,0.19369608902076));
#18868=DIRECTION('',(1.18600730662684E-17,0.19369608902076,-0.981061580685974));
#18869=DIRECTION('center_axis',(-1.18600730662687E-17,-0.193696089020763,
0.981061580685973));
#18870=DIRECTION('ref_axis',(-1.,6.12303176911196E-17,3.04400344543169E-34));
#18871=DIRECTION('center_axis',(-1.50855276528563E-32,-2.46373499627365E-16,
1.));
#18872=DIRECTION('ref_axis',(0.,-1.,-2.46373499627365E-16));
#18873=DIRECTION('center_axis',(1.,-6.12303176911189E-17,0.));
#18874=DIRECTION('ref_axis',(5.75556361012452E-17,0.939985913376917,0.341213250992636));
#18875=DIRECTION('',(-1.,6.12303176911189E-17,0.));
#18876=DIRECTION('',(1.,-6.12303176911189E-17,0.));
#18877=DIRECTION('center_axis',(2.64577897101399E-17,0.419573777126289,
0.907721237797144));
#18878=DIRECTION('ref_axis',(1.,-6.30587304367601E-17,-1.7798463758201E-33));
#18879=DIRECTION('',(-5.72397488459722E-17,-0.907721237797144,0.419573777126289));
#18880=DIRECTION('',(-1.,6.12303176911189E-17,0.));
#18881=DIRECTION('',(5.55800597652948E-17,0.907721237797144,-0.419573777126289));
#18882=DIRECTION('center_axis',(-2.64577897101398E-17,-0.419573777126288,
-0.907721237797145));
#18883=DIRECTION('ref_axis',(1.,-1.6659881145224E-34,-2.91474833995815E-17));
#18884=DIRECTION('',(5.72397488459722E-17,0.907721237797144,-0.419573777126288));
#18885=DIRECTION('',(1.,-6.305873043676E-17,0.));
#18886=DIRECTION('',(-5.55800597652948E-17,-0.907721237797144,0.419573777126288));
#18887=DIRECTION('center_axis',(-5.72397488459722E-17,-0.907721237797144,
0.419573777126289));
#18888=DIRECTION('ref_axis',(-1.,6.06873725410465E-33,-1.36423561162507E-16));
#18889=DIRECTION('',(1.,-6.305873043676E-17,0.));
#18890=DIRECTION('',(-2.64577897101398E-17,-0.419573777126289,-0.907721237797144));
#18891=DIRECTION('',(2.56906356683054E-17,0.419573777126289,0.907721237797144));
#18892=DIRECTION('center_axis',(5.72397488459722E-17,0.907721237797144,
-0.419573777126289));
#18893=DIRECTION('ref_axis',(-5.56772127245432E-34,-0.419573777126289,-0.907721237797144));
#18894=DIRECTION('',(1.,-6.12303176911189E-17,0.));
#18895=DIRECTION('',(2.64577897101398E-17,0.419573777126289,0.907721237797144));
#18896=DIRECTION('',(1.,-6.305873043676E-17,0.));
#18897=DIRECTION('',(-2.56906356683054E-17,-0.419573777126289,-0.907721237797144));
#18898=DIRECTION('center_axis',(2.64577897101398E-17,0.419573777126289,
0.907721237797144));
#18899=DIRECTION('ref_axis',(1.,-6.30587304367598E-17,4.62196821834101E-33));
#18900=DIRECTION('',(1.,-6.12303176911189E-17,0.));
#18901=DIRECTION('',(-5.72397488459722E-17,-0.907721237797144,0.419573777126289));
#18902=DIRECTION('',(1.,-6.305873043676E-17,0.));
#18903=DIRECTION('',(5.55800597652948E-17,0.907721237797144,-0.419573777126289));
#18904=DIRECTION('center_axis',(-2.64577897101398E-17,-0.419573777126289,
-0.907721237797144));
#18905=DIRECTION('ref_axis',(1.,7.16552847671617E-35,-2.91474833995815E-17));
#18906=DIRECTION('',(1.,-6.305873043676E-17,0.));
#18907=DIRECTION('',(5.72397488459722E-17,0.907721237797144,-0.419573777126289));
#18908=DIRECTION('',(-1.,6.12303176911189E-17,0.));
#18909=DIRECTION('',(-5.55800597652948E-17,-0.907721237797144,0.419573777126289));
#18910=DIRECTION('center_axis',(-7.16258653671378E-18,-1.,-4.9960036108132E-16));
#18911=DIRECTION('ref_axis',(-1.73759657126474E-49,4.9960036108132E-16,
-1.));
#18912=DIRECTION('',(3.05906888276069E-32,4.9960036108132E-16,-1.));
#18913=DIRECTION('center_axis',(-5.55800597652948E-17,-0.907721237797145,
0.419573777126288));
#18914=DIRECTION('ref_axis',(-8.12311769207607E-32,-0.419573777126288,-0.907721237797145));
#18915=DIRECTION('',(5.55800597652948E-17,0.907721237797144,-0.419573777126288));
#18916=DIRECTION('center_axis',(2.56906356683053E-17,0.419573777126289,
0.907721237797144));
#18917=DIRECTION('ref_axis',(-7.58956401293417E-33,-0.907721237797144,0.419573777126289));
#18918=DIRECTION('',(-2.56906356683053E-17,-0.419573777126289,-0.907721237797144));
#18919=DIRECTION('center_axis',(1.,-6.12303176911189E-17,0.));
#18920=DIRECTION('ref_axis',(0.,1.,0.));
#18921=DIRECTION('center_axis',(1.,-6.12303176911189E-17,0.));
#18922=DIRECTION('ref_axis',(6.12303176911189E-17,1.,0.));
#18923=DIRECTION('center_axis',(-1.,6.12303176911189E-17,0.));
#18924=DIRECTION('ref_axis',(6.12303176911189E-17,1.,0.));
#18925=DIRECTION('center_axis',(-2.56906356683053E-17,-0.419573777126289,
-0.907721237797144));
#18926=DIRECTION('ref_axis',(7.58956401293417E-33,0.907721237797144,-0.419573777126289));
#18927=DIRECTION('',(2.56906356683053E-17,0.419573777126289,0.907721237797144));
#18928=DIRECTION('center_axis',(-5.55800597652948E-17,-0.907721237797144,
0.419573777126289));
#18929=DIRECTION('ref_axis',(-1.29808072260833E-31,-0.419573777126289,-0.907721237797144));
#18930=DIRECTION('',(5.55800597652948E-17,0.907721237797144,-0.419573777126289));
#18931=DIRECTION('center_axis',(5.72397488459722E-17,0.907721237797145,
-0.419573777126288));
#18932=DIRECTION('ref_axis',(8.70154526560722E-32,0.419573777126288,0.907721237797145));
#18933=DIRECTION('',(-5.72397488459722E-17,-0.907721237797144,0.419573777126288));
#18934=DIRECTION('center_axis',(-2.64577897101398E-17,-0.419573777126289,
-0.907721237797144));
#18935=DIRECTION('ref_axis',(9.2001233786812E-33,0.907721237797144,-0.419573777126289));
#18936=DIRECTION('',(2.64577897101398E-17,0.419573777126289,0.907721237797144));
#18937=DIRECTION('center_axis',(1.,-6.305873043676E-17,0.));
#18938=DIRECTION('ref_axis',(0.,1.,0.));
#18939=DIRECTION('center_axis',(-1.,6.305873043676E-17,0.));
#18940=DIRECTION('ref_axis',(6.305873043676E-17,1.,0.));
#18941=DIRECTION('center_axis',(1.,-6.305873043676E-17,0.));
#18942=DIRECTION('ref_axis',(6.305873043676E-17,1.,0.));
#18943=DIRECTION('center_axis',(1.,-6.305873043676E-17,0.));
#18944=DIRECTION('ref_axis',(0.,1.,0.));
#18945=DIRECTION('center_axis',(0.,1.,0.));
#18946=DIRECTION('ref_axis',(0.,0.,-1.));
#18947=DIRECTION('center_axis',(1.,-6.305873043676E-17,0.));
#18948=DIRECTION('ref_axis',(6.305873043676E-17,1.,0.));
#18949=DIRECTION('center_axis',(0.,0.525870255519711,-0.85056479727275));
#18950=DIRECTION('ref_axis',(0.,-0.85056479727275,-0.525870255519711));
#18951=DIRECTION('center_axis',(-1.,6.305873043676E-17,0.));
#18952=DIRECTION('ref_axis',(6.305873043676E-17,1.,0.));
#18953=DIRECTION('center_axis',(6.305873043676E-17,1.,-1.71170019451462E-16));
#18954=DIRECTION('ref_axis',(1.07937641154447E-32,1.71170019451462E-16,
1.));
#18955=DIRECTION('',(-6.305873043676E-17,-1.,1.71170019451462E-16));
#18956=DIRECTION('',(6.305873043676E-17,1.,-1.71170019451462E-16));
#18957=DIRECTION('center_axis',(-1.,8.82754440022857E-17,0.));
#18958=DIRECTION('ref_axis',(8.82754440022857E-17,1.,0.));
#18959=DIRECTION('center_axis',(1.,-8.82754440022857E-17,0.));
#18960=DIRECTION('ref_axis',(-8.82754440022857E-17,-1.,0.));
#18961=DIRECTION('',(8.82754440022857E-17,1.,0.));
#18962=DIRECTION('',(-1.3611865338937E-31,-1.5419764230905E-15,-1.));
#18963=DIRECTION('',(-8.82754440022857E-17,-1.,0.));
#18964=DIRECTION('center_axis',(-0.948683298050517,3.48666447216684E-15,
-0.316227766016828));
#18965=DIRECTION('ref_axis',(0.316227766016828,3.38856734140111E-13,-0.948683298050517));
#18966=DIRECTION('center_axis',(0.,-1.,0.));
#18967=DIRECTION('ref_axis',(0.,0.,1.));
#18968=DIRECTION('center_axis',(-1.,0.,0.));
#18969=DIRECTION('ref_axis',(0.,1.96105308347356E-6,-0.999999999998077));
#18970=DIRECTION('center_axis',(-6.12303176911189E-17,-1.,-6.16297582203916E-33));
#18971=DIRECTION('ref_axis',(-1.,6.12303176911189E-17,3.77360967506142E-49));
#18972=DIRECTION('',(-6.12303176911189E-17,-1.,-5.89862595156241E-33));
#18973=DIRECTION('center_axis',(0.,-1.,0.));
#18974=DIRECTION('ref_axis',(0.,0.,1.));
#18975=DIRECTION('',(6.12303176911189E-17,1.,6.16297582203916E-33));
#18976=DIRECTION('center_axis',(-0.707106781204563,-5.65566764166261E-12,
-0.707106781168532));
#18977=DIRECTION('ref_axis',(0.673256666820156,0.305697433935813,-0.673256666856907));
#18978=DIRECTION('center_axis',(-0.707106781186548,4.32963728535968E-17,
-0.707106781186548));
#18979=DIRECTION('ref_axis',(2.30001377051388E-33,1.,6.12303176911189E-17));
#18980=DIRECTION('',(0.707106781186547,-6.05177407449811E-17,-0.707106781186547));
#18981=DIRECTION('',(-6.12303176911189E-17,-1.,0.));
#18982=DIRECTION('center_axis',(8.55850097257312E-17,1.,0.));
#18983=DIRECTION('ref_axis',(1.,-8.55850097257312E-17,0.));
#18984=DIRECTION('',(-0.707106781186547,6.05177407449811E-17,0.707106781186547));
#18985=DIRECTION('',(0.,0.,-1.));
#18986=DIRECTION('',(-1.,8.55850097257312E-17,0.));
#18987=DIRECTION('',(0.,0.,1.));
#18988=DIRECTION('',(-1.,8.55850097257312E-17,0.));
#18989=DIRECTION('center_axis',(7.16258653671378E-18,1.,4.9960036108132E-16));
#18990=DIRECTION('ref_axis',(1.,-7.16258653671378E-18,0.));
#18991=DIRECTION('',(-3.05906888276069E-32,-4.9960036108132E-16,1.));
#18992=DIRECTION('center_axis',(1.,-6.12303176911189E-17,0.));
#18993=DIRECTION('ref_axis',(0.,-0.357902634963279,-0.93375891100773));
#18994=DIRECTION('center_axis',(-1.,6.12303176911189E-17,0.));
#18995=DIRECTION('ref_axis',(6.12303176911189E-17,1.,0.));
#18996=DIRECTION('center_axis',(0.,0.939692620785909,-0.342020143325668));
#18997=DIRECTION('ref_axis',(0.,-0.342020143325668,-0.939692620785909));
#18998=DIRECTION('center_axis',(0.,-0.939692620785909,0.342020143325668));
#18999=DIRECTION('ref_axis',(0.,-0.342020143325668,-0.939692620785909));
#19000=DIRECTION('',(0.,0.342020143325668,0.939692620785909));
#19001=DIRECTION('center_axis',(0.,-0.939692620785909,0.342020143325668));
#19002=DIRECTION('ref_axis',(0.,-0.342020143325668,-0.939692620785909));
#19003=DIRECTION('',(0.,0.342020143325668,0.939692620785909));
#19004=DIRECTION('center_axis',(0.,0.342020143325668,0.939692620785909));
#19005=DIRECTION('ref_axis',(1.,0.,0.));
#19006=DIRECTION('',(-5.75376777027213E-17,-0.939692620785909,0.342020143325668));
#19007=DIRECTION('center_axis',(0.,0.342020143325668,0.939692620785909));
#19008=DIRECTION('ref_axis',(1.,0.,0.));
#19009=DIRECTION('',(5.75376777027213E-17,0.939692620785909,-0.342020143325668));
#19010=DIRECTION('center_axis',(0.,0.342020143325668,0.939692620785909));
#19011=DIRECTION('ref_axis',(1.,0.,0.));
#19012=DIRECTION('',(-5.75376777027213E-17,-0.939692620785909,0.342020143325668));
#19013=DIRECTION('',(0.894427190999916,0.420243315606445,-0.152956058030083));
#19014=DIRECTION('center_axis',(1.,-6.12303176911189E-17,0.));
#19015=DIRECTION('ref_axis',(0.,1.,0.));
#19016=DIRECTION('center_axis',(-6.6521838836082E-15,0.843685290277401,
0.536838086362674));
#19017=DIRECTION('ref_axis',(1.87310260347094E-29,0.536838086362674,-0.843685290277401));
#19018=DIRECTION('center_axis',(-1.,6.12303176911189E-17,0.));
#19019=DIRECTION('ref_axis',(6.12303176911189E-17,1.,0.));
#19020=DIRECTION('center_axis',(-5.75376777027213E-17,-0.939692620785909,
0.342020143325668));
#19021=DIRECTION('ref_axis',(8.8935491616808E-32,-0.342020143325668,-0.939692620785909));
#19022=DIRECTION('',(5.75376777027213E-17,0.939692620785909,-0.342020143325668));
#19023=DIRECTION('center_axis',(7.4313463805646E-16,0.939692620785909,-0.342020143325667));
#19024=DIRECTION('ref_axis',(1.85564127880603E-30,-0.342020143325667,-0.939692620785909));
#19025=DIRECTION('center_axis',(0.948683298050523,-0.297156898213624,0.108156265856586));
#19026=DIRECTION('ref_axis',(0.316227766016811,0.891470694640734,-0.324468797570405));
#19027=DIRECTION('center_axis',(-1.,-2.35521515975489E-13,-5.36913090858677E-14));
#19028=DIRECTION('ref_axis',(-2.02953649309067E-13,0.939690866223616,-0.342024963907476));
#19029=DIRECTION('center_axis',(0.894427190999916,0.420243315606445,-0.152956058030083));
#19030=DIRECTION('ref_axis',(0.425247203315731,-0.90507724315229,-5.35984724282349E-16));
#19031=DIRECTION('',(-0.894427190999916,-0.420243315606445,0.152956058030083));
#19032=DIRECTION('center_axis',(5.75376777027213E-17,0.939692620785909,
-0.342020143325668));
#19033=DIRECTION('ref_axis',(-8.8935491616808E-32,0.342020143325668,0.939692620785909));
#19034=DIRECTION('center_axis',(0.,-0.939692620785909,0.342020143325668));
#19035=DIRECTION('ref_axis',(0.,0.342020143325668,0.939692620785909));
#19036=DIRECTION('',(5.75376777027213E-17,0.939692620785909,-0.342020143325668));
#19037=DIRECTION('center_axis',(-1.,-1.10682065829975E-15,2.76579965799101E-15));
#19038=DIRECTION('ref_axis',(-1.98603300901544E-15,0.9396922190012,-0.342021247218065));
#19039=DIRECTION('center_axis',(-5.75376777027213E-17,-0.939692620785909,
0.342020143325668));
#19040=DIRECTION('ref_axis',(8.8935491616808E-32,-0.342020143325668,-0.939692620785909));
#19041=DIRECTION('',(-5.75376777027213E-17,-0.939692620785909,0.342020143325668));
#19042=DIRECTION('center_axis',(-1.,6.12303176911189E-17,0.));
#19043=DIRECTION('ref_axis',(6.12303176911189E-17,1.,0.));
#19044=DIRECTION('center_axis',(-1.,8.82766640598215E-17,0.));
#19045=DIRECTION('ref_axis',(8.82766640598215E-17,1.,0.));
#19046=DIRECTION('center_axis',(1.,-8.82766640598215E-17,0.));
#19047=DIRECTION('ref_axis',(-8.82766640598215E-17,-1.,0.));
#19048=DIRECTION('center_axis',(1.,-6.12303176911189E-17,0.));
#19049=DIRECTION('ref_axis',(0.,1.,0.));
#19050=DIRECTION('center_axis',(1.,-6.12303176911189E-17,0.));
#19051=DIRECTION('ref_axis',(6.12303176911189E-17,1.,0.));
#19052=DIRECTION('center_axis',(-3.98057119674385E-15,0.902145193524675,
-0.431432555332032));
#19053=DIRECTION('ref_axis',(2.30883845873134E-29,-0.431432555332032,-0.902145193524675));
#19054=DIRECTION('center_axis',(1.,-6.12303176911189E-17,0.));
#19055=DIRECTION('ref_axis',(0.,-0.679936320676586,0.733271163911951));
#19056=DIRECTION('center_axis',(1.,-6.12303176911189E-17,0.));
#19057=DIRECTION('ref_axis',(6.12303176911189E-17,1.,0.));
#19058=DIRECTION('center_axis',(0.,0.968402813368906,-0.249391240943199));
#19059=DIRECTION('ref_axis',(0.,-0.249391240943199,-0.968402813368906));
#19060=DIRECTION('center_axis',(1.,-6.12303176911189E-17,0.));
#19061=DIRECTION('ref_axis',(0.,1.,0.));
#19062=DIRECTION('center_axis',(-1.,6.12303176911189E-17,0.));
#19063=DIRECTION('ref_axis',(6.12303176911189E-17,1.,0.));
#19064=DIRECTION('center_axis',(-5.63595351442503E-15,0.673655460688034,
0.739045546827253));
#19065=DIRECTION('ref_axis',(-8.67000511622114E-30,0.739045546827253,-0.673655460688034));
#19066=DIRECTION('center_axis',(3.05906888276069E-32,4.9960036108132E-16,
-1.));
#19067=DIRECTION('ref_axis',(-3.06415924378128E-57,1.,4.9960036108132E-16));
#19068=DIRECTION('',(3.05906888276069E-32,4.9960036108132E-16,-1.));
#19069=DIRECTION('center_axis',(0.894427190999906,-4.00966414299127E-14,
0.447213595499978));
#19070=DIRECTION('ref_axis',(0.447213595499978,4.85406311470918E-13,-0.894427190999906));
#19071=DIRECTION('center_axis',(-1.,0.,0.));
#19072=DIRECTION('ref_axis',(0.,0.112528245522859,0.993648526371145));
#19073=DIRECTION('center_axis',(-1.,0.,0.));
#19074=DIRECTION('ref_axis',(0.,0.,-1.));
#19075=DIRECTION('center_axis',(-1.,0.,0.));
#19076=DIRECTION('ref_axis',(0.,0.,-1.));
#19077=DIRECTION('center_axis',(1.,-6.12303176911189E-17,0.));
#19078=DIRECTION('ref_axis',(-6.12303176911189E-17,-1.,0.));
#19079=DIRECTION('',(-1.,6.12303176911189E-17,0.));
#19080=DIRECTION('center_axis',(1.,-6.305873043676E-17,0.));
#19081=DIRECTION('ref_axis',(6.305873043676E-17,1.,0.));
#19082=DIRECTION('',(1.,-6.12303176911189E-17,0.));
#19083=DIRECTION('center_axis',(-1.,6.12303176911189E-17,0.));
#19084=DIRECTION('ref_axis',(6.12303176911189E-17,1.,0.));
#19085=DIRECTION('center_axis',(1.89956701267235E-32,3.10233081307019E-16,
1.));
#19086=DIRECTION('ref_axis',(0.,1.,-3.10233081307019E-16));
#19087=DIRECTION('',(-1.,6.12303176911189E-17,0.));
#19088=DIRECTION('',(6.305873043676E-17,1.,-3.10233081307019E-16));
#19089=DIRECTION('',(-6.12303176911189E-17,-1.,3.10233081307019E-16));
#19090=DIRECTION('center_axis',(1.,-6.305873043676E-17,0.));
#19091=DIRECTION('ref_axis',(0.,1.,0.));
#19092=DIRECTION('center_axis',(-1.,6.305873043676E-17,0.));
#19093=DIRECTION('ref_axis',(6.305873043676E-17,1.,0.));
#19094=DIRECTION('center_axis',(0.,0.873412217959863,0.486981619281912));
#19095=DIRECTION('ref_axis',(0.,0.486981619281912,-0.873412217959863));
#19096=DIRECTION('center_axis',(1.,-6.12303176911189E-17,0.));
#19097=DIRECTION('ref_axis',(-6.12303176911189E-17,-1.,0.));
#19098=DIRECTION('center_axis',(-1.,6.305873043676E-17,0.));
#19099=DIRECTION('ref_axis',(6.305873043676E-17,1.,0.));
#19100=DIRECTION('center_axis',(-1.,6.12303176911189E-17,0.));
#19101=DIRECTION('ref_axis',(6.12303176911189E-17,1.,0.));
#19102=DIRECTION('center_axis',(-1.,0.,0.));
#19103=DIRECTION('ref_axis',(0.,0.,1.));
#19104=DIRECTION('',(1.,-6.12303176911189E-17,0.));
#19105=DIRECTION('center_axis',(-1.,6.12303176911189E-17,0.));
#19106=DIRECTION('ref_axis',(6.12303176911189E-17,1.,0.));
#19107=DIRECTION('center_axis',(-1.,0.,0.));
#19108=DIRECTION('ref_axis',(0.,0.,1.));
#19109=DIRECTION('center_axis',(1.,-6.12303176911189E-17,0.));
#19110=DIRECTION('ref_axis',(-6.12303176911189E-17,-1.,0.));
#19111=DIRECTION('',(1.,-6.12303176911189E-17,0.));
#19112=DIRECTION('center_axis',(-1.,6.12303176911189E-17,0.));
#19113=DIRECTION('ref_axis',(6.12303176911189E-17,1.,0.));
#19114=DIRECTION('center_axis',(1.65126718156494E-17,0.419573777126287,
0.907721237797145));
#19115=DIRECTION('ref_axis',(1.,-3.93558242098606E-17,1.53156320849217E-33));
#19116=DIRECTION('',(3.4350885432143E-17,0.907721237797145,-0.419573777126287));
#19117=DIRECTION('',(3.4350885432143E-17,0.907721237797145,-0.419573777126287));
#19118=DIRECTION('center_axis',(-1.,3.78429896776521E-17,0.));
#19119=DIRECTION('ref_axis',(3.78429896776521E-17,1.,0.));
#19120=DIRECTION('',(0.,-0.882947592858927,0.469471562785891));
#19121=DIRECTION('center_axis',(-8.55850097257312E-17,-1.,1.54197642309049E-15));
#19122=DIRECTION('ref_axis',(9.35280776177934E-48,-1.54197642309049E-15,
-1.));
#19123=DIRECTION('',(1.3611865338937E-31,1.5419764230905E-15,1.));
#19124=DIRECTION('',(1.,-8.55850097257312E-17,0.));
#19125=DIRECTION('',(-1.3611865338937E-31,-1.5419764230905E-15,-1.));
#19126=DIRECTION('',(-1.,8.55850097257312E-17,0.));
#19127=DIRECTION('center_axis',(8.68731872386614E-33,1.37765518964554E-16,
1.));
#19128=DIRECTION('ref_axis',(0.,1.,-1.37765518964554E-16));
#19129=DIRECTION('',(1.,-6.12303176911189E-17,0.));
#19130=DIRECTION('',(-6.305873043676E-17,-1.,1.37765518964554E-16));
#19131=DIRECTION('',(1.,0.,0.));
#19132=DIRECTION('',(0.,1.,-1.33305621742574E-16));
#19133=DIRECTION('',(-1.,1.1968129724039E-48,8.68731872386614E-33));
#19134=DIRECTION('',(6.12303176911189E-17,1.,-1.37765518964554E-16));
#19135=DIRECTION('center_axis',(-3.05906888276069E-32,-4.9960036108132E-16,
1.));
#19136=DIRECTION('ref_axis',(3.06415924378128E-57,-1.,-4.9960036108132E-16));
#19137=DIRECTION('center_axis',(0.894431478679542,-2.13240231356641E-5,
0.447205019529537));
#19138=DIRECTION('ref_axis',(0.447205018870395,-2.96107870526001E-5,-0.894431478773154));
#19139=DIRECTION('',(-3.05906888276069E-32,-4.9960036108132E-16,1.));
#19140=DIRECTION('center_axis',(-0.707106780946326,8.56130761774713E-10,
-0.707106781426769));
#19141=DIRECTION('ref_axis',(0.707106553895062,-0.000802219031349341,-0.707106553415591));
#19142=DIRECTION('center_axis',(-0.707106780941704,-8.72599632391827E-10,
-0.707106781431391));
#19143=DIRECTION('ref_axis',(0.707106548468998,0.000811736179642942,-0.707106547980313));
#19144=DIRECTION('center_axis',(-5.72397488459722E-17,-0.907721237797144,
0.419573777126289));
#19145=DIRECTION('ref_axis',(-1.1368799380976E-31,-0.419573777126289,-0.907721237797144));
#19146=DIRECTION('',(5.72397488459722E-17,0.907721237797144,-0.419573777126289));
#19147=DIRECTION('center_axis',(1.,-6.305873043676E-17,0.));
#19148=DIRECTION('ref_axis',(0.,1.,0.));
#19149=DIRECTION('center_axis',(1.,-6.305873043676E-17,0.));
#19150=DIRECTION('ref_axis',(6.305873043676E-17,1.,0.));
#19151=DIRECTION('center_axis',(-6.305873043676E-17,-1.,3.10233081307019E-16));
#19152=DIRECTION('ref_axis',(1.95629042467048E-32,3.10233081307019E-16,
1.));
#19153=DIRECTION('center_axis',(1.,-6.305873043676E-17,0.));
#19154=DIRECTION('ref_axis',(0.,-0.991300262557005,-0.131619867248123));
#19155=DIRECTION('center_axis',(0.,-0.512782925680917,0.858518299822502));
#19156=DIRECTION('ref_axis',(0.,0.858518299822502,0.512782925680917));
#19157=DIRECTION('center_axis',(1.,-6.305873043676E-17,0.));
#19158=DIRECTION('ref_axis',(6.305873043676E-17,1.,0.));
#19159=DIRECTION('center_axis',(6.305873043676E-17,1.,-3.10233081307019E-16));
#19160=DIRECTION('ref_axis',(1.95629042467048E-32,3.10233081307019E-16,
1.));
#19161=DIRECTION('',(-6.305873043676E-17,-1.,3.10233081307019E-16));
#19162=DIRECTION('center_axis',(1.,-6.12303176911189E-17,0.));
#19163=DIRECTION('ref_axis',(-6.12303176911189E-17,-1.,0.));
#19164=DIRECTION('center_axis',(1.,-6.37765983815004E-17,0.));
#19165=DIRECTION('ref_axis',(-6.37765983815004E-17,-1.,0.));
#19166=DIRECTION('center_axis',(-1.,0.,0.));
#19167=DIRECTION('ref_axis',(0.,0.,-1.));
#19168=DIRECTION('center_axis',(1.,-6.12303176911189E-17,0.));
#19169=DIRECTION('ref_axis',(0.,-0.855521656752581,-0.517767027559035));
#19170=DIRECTION('center_axis',(1.,-6.12303176911189E-17,0.));
#19171=DIRECTION('ref_axis',(6.12303176911189E-17,1.,0.));
#19172=DIRECTION('center_axis',(1.,-6.12303176911189E-17,0.));
#19173=DIRECTION('ref_axis',(6.12303176911189E-17,1.,0.));
#19174=DIRECTION('center_axis',(1.,0.,0.));
#19175=DIRECTION('ref_axis',(0.,0.,1.));
#19176=DIRECTION('center_axis',(1.,0.,0.));
#19177=DIRECTION('ref_axis',(0.,0.,1.));
#19178=DIRECTION('center_axis',(1.,0.,0.));
#19179=DIRECTION('ref_axis',(0.,0.,1.));
#19180=DIRECTION('',(0.,-0.882947592858927,0.469471562785891));
#19181=DIRECTION('center_axis',(1.,-6.12303176911189E-17,0.));
#19182=DIRECTION('ref_axis',(0.,0.,1.));
#19183=DIRECTION('',(-5.55800597652948E-17,-0.907721237797144,0.419573777126289));
#19184=DIRECTION('center_axis',(-1.,6.12303176911189E-17,0.));
#19185=DIRECTION('ref_axis',(6.12303176911189E-17,1.,0.));
#19186=DIRECTION('',(-6.12303176911189E-17,-1.,1.37765518964554E-16));
#19187=DIRECTION('',(6.12303176911189E-17,1.,1.13606963518701E-16));
#19188=DIRECTION('center_axis',(1.,-6.305873043676E-17,0.));
#19189=DIRECTION('ref_axis',(-6.305873043676E-17,-1.,0.));
#19190=DIRECTION('',(-5.55800597652948E-17,-0.907721237797144,0.419573777126289));
#19191=DIRECTION('center_axis',(1.,-6.12303176911189E-17,0.));
#19192=DIRECTION('ref_axis',(6.12303176911189E-17,1.,0.));
#19193=DIRECTION('center_axis',(-1.,6.12303176911189E-17,0.));
#19194=DIRECTION('ref_axis',(6.12303176911189E-17,1.,0.));
#19195=DIRECTION('center_axis',(0.,0.,1.));
#19196=DIRECTION('ref_axis',(-1.,0.,0.));
#19197=DIRECTION('center_axis',(0.,0.,-1.));
#19198=DIRECTION('ref_axis',(-1.,0.,0.));
#19199=DIRECTION('center_axis',(0.,0.,-1.));
#19200=DIRECTION('ref_axis',(-1.,0.,0.));
#19201=DIRECTION('',(8.82754440022857E-17,1.,0.));
#19202=DIRECTION('center_axis',(1.,-6.305873043676E-17,0.));
#19203=DIRECTION('ref_axis',(0.,0.,1.));
#19204=DIRECTION('center_axis',(1.,-6.12303176911189E-17,0.));
#19205=DIRECTION('ref_axis',(-6.12303176911189E-17,-1.,0.));
#19206=DIRECTION('center_axis',(1.,-6.305873043676E-17,0.));
#19207=DIRECTION('ref_axis',(6.305873043676E-17,1.,0.));
#19208=DIRECTION('center_axis',(1.,-6.12303176911189E-17,0.));
#19209=DIRECTION('ref_axis',(-6.12303176911189E-17,-1.,0.));
#19210=DIRECTION('center_axis',(1.,-6.305873043676E-17,0.));
#19211=DIRECTION('ref_axis',(6.305873043676E-17,1.,0.));
#19212=DIRECTION('',(1.,-6.305873043676E-17,0.));
#19213=DIRECTION('center_axis',(-1.,6.12303176911189E-17,0.));
#19214=DIRECTION('ref_axis',(6.12303176911189E-17,1.,0.));
#19215=DIRECTION('center_axis',(1.,-6.305873043676E-17,0.));
#19216=DIRECTION('ref_axis',(0.,0.,1.));
#19217=DIRECTION('',(6.50521303491303E-17,0.882947592858927,-0.469471562785891));
#19218=DIRECTION('center_axis',(-1.,0.,0.));
#19219=DIRECTION('ref_axis',(0.,0.,-1.));
#19220=DIRECTION('',(6.305873043676E-17,1.,-1.37765518964554E-16));
#19221=DIRECTION('center_axis',(1.,-6.305873043676E-17,0.));
#19222=DIRECTION('ref_axis',(6.305873043676E-17,1.,0.));
#19223=DIRECTION('center_axis',(1.,-6.305873043676E-17,0.));
#19224=DIRECTION('ref_axis',(0.,0.,1.));
#19225=DIRECTION('',(-2.64577897101398E-17,-0.419573777126289,-0.907721237797144));
#19226=DIRECTION('center_axis',(1.,-6.305873043676E-17,0.));
#19227=DIRECTION('ref_axis',(6.305873043676E-17,1.,0.));
#19228=DIRECTION('',(-5.72397488459722E-17,-0.907721237797144,0.419573777126289));
#19229=DIRECTION('center_axis',(-1.,6.305873043676E-17,0.));
#19230=DIRECTION('ref_axis',(6.305873043676E-17,1.,0.));
#19231=DIRECTION('center_axis',(1.,-6.305873043676E-17,0.));
#19232=DIRECTION('ref_axis',(0.,0.,1.));
#19233=DIRECTION('',(-6.305873043676E-17,-1.,-1.13606963518701E-16));
#19234=DIRECTION('center_axis',(-1.,6.305873043676E-17,0.));
#19235=DIRECTION('ref_axis',(6.305873043676E-17,1.,0.));
#19236=DIRECTION('',(5.72397488459722E-17,0.907721237797144,-0.419573777126289));
#19237=DIRECTION('center_axis',(7.16391088826457E-33,1.13606963518701E-16,
-1.));
#19238=DIRECTION('ref_axis',(0.,1.,1.13606963518701E-16));
#19239=DIRECTION('',(6.305873043676E-17,1.,1.13606963518701E-16));
#19240=DIRECTION('',(-1.,6.12303176911189E-17,0.));
#19241=DIRECTION('',(-6.12303176911189E-17,-1.,-1.13606963518701E-16));
#19242=DIRECTION('center_axis',(1.,-6.12303176911189E-17,0.));
#19243=DIRECTION('ref_axis',(-6.12303176911189E-17,-1.,0.));
#19244=DIRECTION('center_axis',(-1.,6.305873043676E-17,0.));
#19245=DIRECTION('ref_axis',(6.305873043676E-17,1.,0.));
#19246=DIRECTION('center_axis',(1.,-6.12303176911189E-17,0.));
#19247=DIRECTION('ref_axis',(6.12303176911189E-17,1.,0.));
#19248=DIRECTION('center_axis',(1.,-6.12303176911189E-17,0.));
#19249=DIRECTION('ref_axis',(5.75176428514148E-17,0.939365416027515,0.342917796521927));
#19250=DIRECTION('center_axis',(1.,-6.12303176911189E-17,0.));
#19251=DIRECTION('ref_axis',(-6.12303176911189E-17,-1.,0.));
#19252=DIRECTION('center_axis',(-1.,6.305873043676E-17,0.));
#19253=DIRECTION('ref_axis',(6.305873043676E-17,1.,0.));
#19254=DIRECTION('center_axis',(1.,-6.12303176911189E-17,0.));
#19255=DIRECTION('ref_axis',(6.12303176911189E-17,1.,0.));
#19256=DIRECTION('center_axis',(1.,-6.12303176911189E-17,0.));
#19257=DIRECTION('ref_axis',(-6.12303176911189E-17,-1.,0.));
#19258=DIRECTION('center_axis',(1.,-6.12303176911189E-17,0.));
#19259=DIRECTION('ref_axis',(0.,1.,0.));
#19260=DIRECTION('center_axis',(1.,-6.12303176911189E-17,0.));
#19261=DIRECTION('ref_axis',(0.,1.,0.));
#19262=DIRECTION('center_axis',(5.55800597652948E-17,0.907721237797144,
-0.419573777126289));
#19263=DIRECTION('ref_axis',(1.29808072260833E-31,0.419573777126289,0.907721237797144));
#19264=DIRECTION('center_axis',(5.55800597652948E-17,0.907721237797144,
-0.419573777126289));
#19265=DIRECTION('ref_axis',(1.29808072260833E-31,0.419573777126289,0.907721237797144));
#19266=DIRECTION('center_axis',(-6.12303176911189E-17,-1.,-1.13606963518701E-16));
#19267=DIRECTION('ref_axis',(6.95619046817341E-33,1.13606963518701E-16,
-1.));
#19268=DIRECTION('center_axis',(1.,-6.12303176911189E-17,0.));
#19269=DIRECTION('ref_axis',(0.,1.,0.));
#19270=DIRECTION('center_axis',(6.12303176911189E-17,1.,-1.37765518964554E-16));
#19271=DIRECTION('ref_axis',(8.43542649308151E-33,1.37765518964554E-16,
1.));
#19272=DIRECTION('center_axis',(0.707106781186548,-1.06487712312249E-15,
0.707106781186548));
#19273=DIRECTION('ref_axis',(-1.50596366978067E-15,-1.,3.33894885375682E-33));
#19274=DIRECTION('',(7.1625865367138E-18,1.,1.49880108324396E-15));
#19275=DIRECTION('center_axis',(-1.,0.,0.));
#19276=DIRECTION('ref_axis',(0.,0.,1.));
#19277=DIRECTION('center_axis',(-1.,8.82766640598215E-17,0.));
#19278=DIRECTION('ref_axis',(0.,0.93969262078591,-0.342020143325664));
#19279=DIRECTION('center_axis',(-1.3611865338937E-31,-1.5419764230905E-15,
-1.));
#19280=DIRECTION('ref_axis',(-3.05518935066593E-57,1.,-1.5419764230905E-15));
#19281=DIRECTION('center_axis',(1.,-8.55850097257312E-17,0.));
#19282=DIRECTION('ref_axis',(-8.55850097257312E-17,-1.,0.));
#19283=DIRECTION('',(1.,-8.55850097257312E-17,0.));
#19284=DIRECTION('center_axis',(0.923879532511291,2.62280693261509E-15,
-0.382683432365079));
#19285=DIRECTION('ref_axis',(0.382683432365079,-1.7921752496165E-12,0.923879532511291));
#19286=DIRECTION('center_axis',(-1.,8.82754440022857E-17,0.));
#19287=DIRECTION('ref_axis',(0.,0.995871426936473,-0.090775002128966));
#19288=DIRECTION('center_axis',(0.,0.,-1.));
#19289=DIRECTION('ref_axis',(0.,1.,0.));
#19290=DIRECTION('',(-1.,8.55850097257312E-17,0.));
#19291=DIRECTION('',(-8.82754440022857E-17,-1.,0.));
#19292=DIRECTION('center_axis',(5.49761868397523E-12,-9.20733867538014E-13,
-1.));
#19293=DIRECTION('ref_axis',(0.732793660910527,-0.680450917061141,4.65516458078155E-12));
#19294=DIRECTION('center_axis',(8.82754440022857E-17,1.,0.));
#19295=DIRECTION('ref_axis',(1.,-8.82754440022857E-17,0.));
#19296=DIRECTION('center_axis',(-0.707106781186578,-0.707106781186517,1.40152838177972E-12));
#19297=DIRECTION('ref_axis',(0.707106781186517,-0.707106781186578,-1.08700436557221E-11));
#19298=DIRECTION('center_axis',(0.,-1.,0.));
#19299=DIRECTION('ref_axis',(0.,0.,1.));
#19300=DIRECTION('center_axis',(1.,-8.55850097257312E-17,0.));
#19301=DIRECTION('ref_axis',(-8.55850097257312E-17,-1.,0.));
#19302=DIRECTION('center_axis',(1.3611865338937E-31,1.54197642309049E-15,
1.));
#19303=DIRECTION('ref_axis',(-8.16770755219275E-61,-1.,1.54197642309049E-15));
#19304=DIRECTION('center_axis',(1.,-6.12303176911189E-17,0.));
#19305=DIRECTION('ref_axis',(0.,0.,1.));
#19306=DIRECTION('',(-6.12303176911189E-17,-1.,1.71170019451462E-16));
#19307=DIRECTION('',(1.44560289664734E-16,-0.939692620785909,0.342020143325668));
#19308=DIRECTION('center_axis',(1.0480794670208E-32,1.71170019451462E-16,
1.));
#19309=DIRECTION('ref_axis',(0.,1.,-1.71170019451462E-16));
#19310=DIRECTION('center_axis',(5.72397488459722E-17,0.907721237797144,
-0.419573777126289));
#19311=DIRECTION('ref_axis',(1.37844232230888E-31,0.419573777126289,0.907721237797144));
#19312=DIRECTION('center_axis',(2.64577897101398E-17,0.419573777126289,
0.907721237797144));
#19313=DIRECTION('ref_axis',(-5.00442534740975E-33,-0.907721237797144,0.419573777126289));
#19314=DIRECTION('center_axis',(1.,-6.305873043676E-17,0.));
#19315=DIRECTION('ref_axis',(0.,1.,0.));
#19316=DIRECTION('center_axis',(1.,-6.305873043676E-17,0.));
#19317=DIRECTION('ref_axis',(0.,1.,0.));
#19318=DIRECTION('center_axis',(1.,-6.305873043676E-17,0.));
#19319=DIRECTION('ref_axis',(0.,1.,0.));
#19320=DIRECTION('center_axis',(-5.72397488459722E-17,-0.907721237797144,
0.419573777126289));
#19321=DIRECTION('ref_axis',(-1.34762744319869E-31,-0.419573777126289,-0.907721237797144));
#19322=DIRECTION('center_axis',(6.305873043676E-17,1.,1.13606963518701E-16));
#19323=DIRECTION('ref_axis',(-7.16391088826459E-33,-1.13606963518701E-16,
1.));
#19324=DIRECTION('center_axis',(1.,-6.305873043676E-17,0.));
#19325=DIRECTION('ref_axis',(0.,1.,0.));
#19326=DIRECTION('center_axis',(-6.305873043676E-17,-1.,1.37765518964554E-16));
#19327=DIRECTION('ref_axis',(-8.68731872386616E-33,-1.37765518964554E-16,
-1.));
#19328=DIRECTION('center_axis',(1.,0.,0.));
#19329=DIRECTION('ref_axis',(0.,0.112528245522859,0.993648526371145));
#19330=DIRECTION('center_axis',(-1.,0.,0.));
#19331=DIRECTION('ref_axis',(0.,0.,-1.));
#19332=DIRECTION('center_axis',(-1.,0.,0.));
#19333=DIRECTION('ref_axis',(0.,0.0968769480691947,0.995296366381792));
#19334=DIRECTION('center_axis',(0.,0.469471562785891,0.882947592858927));
#19335=DIRECTION('ref_axis',(1.,0.,0.));
#19336=DIRECTION('center_axis',(0.,0.342020143325668,0.939692620785909));
#19337=DIRECTION('ref_axis',(1.,0.,0.));
#19338=DIRECTION('',(0.,0.939692620785909,-0.342020143325668));
#19339=DIRECTION('',(0.894427190999916,0.420243315606445,-0.152956058030083));
#19340=DIRECTION('center_axis',(-1.,0.,0.));
#19341=DIRECTION('ref_axis',(0.,-1.,0.));
#19342=DIRECTION('',(0.,-0.342020143325668,-0.939692620785909));
#19343=DIRECTION('center_axis',(-0.447213595499957,0.84048663121289,-0.305912116060166));
#19344=DIRECTION('ref_axis',(-1.70074100669568E-17,-0.342020143325668,-0.939692620785909));
#19345=DIRECTION('center_axis',(0.707106781186548,-6.05177407449811E-17,
-0.707106781186548));
#19346=DIRECTION('ref_axis',(-0.707106781186548,1.46675000719695E-31,-0.707106781186548));
#19347=DIRECTION('center_axis',(1.,-6.12303176911189E-17,0.));
#19348=DIRECTION('ref_axis',(0.,0.,1.));
#19349=DIRECTION('center_axis',(1.,-6.12303176911189E-17,0.));
#19350=DIRECTION('ref_axis',(0.,0.,1.));
#19351=DIRECTION('center_axis',(1.,-6.12303176911189E-17,0.));
#19352=DIRECTION('ref_axis',(0.,0.,1.));
#35149=CARTESIAN_POINT('',(0.,0.,0.));
#35150=CARTESIAN_POINT('Origin',(-37.718924746634,35.,3.67381906146713E-15));
#35151=CARTESIAN_POINT('',(-37.718924746634,26.8011470173929,-0.137148713427167));
#35152=CARTESIAN_POINT('',(-37.718924746634,25.2013708256647,-0.163909437998321));
#35153=CARTESIAN_POINT('Origin',(-37.718924746634,26.0012589215288,-0.150529075712744));
#35154=CARTESIAN_POINT('Origin',(-37.718924746634,26.0012589215288,-0.150529075712744));
#35155=CARTESIAN_POINT('',(-37.718924746634,26.8,0.));
#35156=CARTESIAN_POINT('Origin',(-37.718924746634,35.,3.67381906146713E-15));
#35157=CARTESIAN_POINT('',(-36.918924746634,26.,0.));
#35158=CARTESIAN_POINT('Origin',(-37.718924746634,26.,0.));
#35159=CARTESIAN_POINT('',(-37.718924746634,25.2,0.));
#35160=CARTESIAN_POINT('Origin',(-37.718924746634,26.,0.));
#35161=CARTESIAN_POINT('',(-38.518924746634,26.,0.));
#35162=CARTESIAN_POINT('Origin',(-37.718924746634,26.,0.));
#35163=CARTESIAN_POINT('Origin',(-37.718924746634,26.,0.));
#35164=CARTESIAN_POINT('Origin',(-17.718924746634,35.,-1.7347234759768E-15));
#35165=CARTESIAN_POINT('',(-18.518924746634,26.,-2.20436423846523E-14));
#35166=CARTESIAN_POINT('',(-17.718924746634,26.8,-2.00842075060165E-14));
#35167=CARTESIAN_POINT('Origin',(-17.718924746634,26.,-2.20436423846523E-14));
#35168=CARTESIAN_POINT('',(-17.718924746634,25.2,-2.40030772632881E-14));
#35169=CARTESIAN_POINT('Origin',(-17.718924746634,26.,-2.20436423846523E-14));
#35170=CARTESIAN_POINT('',(-16.918924746634,26.,-2.20436423846523E-14));
#35171=CARTESIAN_POINT('Origin',(-17.718924746634,26.,-2.20436423846523E-14));
#35172=CARTESIAN_POINT('Origin',(-17.718924746634,26.,-2.20436423846523E-14));
#35173=CARTESIAN_POINT('',(-17.718924746634,26.8044789537624,0.270988524991688));
#35174=CARTESIAN_POINT('Origin',(-17.718924746634,35.,-1.7347234759768E-15));
#35175=CARTESIAN_POINT('',(-17.718924746634,25.20535289596,0.323864334746163));
#35176=CARTESIAN_POINT('Origin',(-17.718924746634,26.0049159248612,0.297426429868925));
#35177=CARTESIAN_POINT('Origin',(-17.718924746634,26.0049159248612,0.297426429868925));
#35178=CARTESIAN_POINT('Origin',(-37.718924746634,21.,-2.5));
#35179=CARTESIAN_POINT('',(-37.3733225893608,18.2550018077979,-2.93018347082097));
#35180=CARTESIAN_POINT('',(-37.718924746634,19.3314643670594,-4.62273145772317));
#35181=CARTESIAN_POINT('Ctrl Pts',(-37.3733232272543,18.2550018791746,-2.93018346215923));
#35182=CARTESIAN_POINT('Ctrl Pts',(-37.3725399318501,18.2873279411122,-3.13887925979283));
#35183=CARTESIAN_POINT('Ctrl Pts',(-37.3771862418788,18.3459461927511,-3.34221139809461));
#35184=CARTESIAN_POINT('Ctrl Pts',(-37.4055310344249,18.5636687830632,-3.84861224630963));
#35185=CARTESIAN_POINT('Ctrl Pts',(-37.4367046322635,18.7448722293728,-4.09334967078263));
#35186=CARTESIAN_POINT('Ctrl Pts',(-37.513662764176,19.0344707879862,-4.3965117730213));
#35187=CARTESIAN_POINT('Ctrl Pts',(-37.5503726296912,19.1412839689907,-4.48376923795396));
#35188=CARTESIAN_POINT('Ctrl Pts',(-37.6047598935936,19.2409031720841,-4.55916514358062));
#35189=CARTESIAN_POINT('Ctrl Pts',(-37.6248502188041,19.2739476093295,-4.58313159510348));
#35190=CARTESIAN_POINT('Ctrl Pts',(-37.6598548373438,19.3077811937435,-4.60665604839667));
#35191=CARTESIAN_POINT('Ctrl Pts',(-37.6713097435794,19.3168085985258,-4.61282433924523));
#35192=CARTESIAN_POINT('Ctrl Pts',(-37.6923292478912,19.327010715773,-4.61973825681333));
#35193=CARTESIAN_POINT('Ctrl Pts',(-37.7011201878655,19.3298589042222,-4.62165247607873));
#35194=CARTESIAN_POINT('Ctrl Pts',(-37.7132641086043,19.3312981704222,-4.62261984197903));
#35195=CARTESIAN_POINT('Ctrl Pts',(-37.7161029581537,19.3314643670594,-4.62273145772315));
#35196=CARTESIAN_POINT('Ctrl Pts',(-37.718924746634,19.3314643670594,-4.62273145772315));
#35197=CARTESIAN_POINT('',(-36.9189423546079,17.5305480470118,-3.0004786401109));
#35198=CARTESIAN_POINT('Ctrl Pts',(-37.3733226583846,18.2550016652924,-2.93018349180643));
#35199=CARTESIAN_POINT('Ctrl Pts',(-37.3516251004149,18.2446527637436,-2.9312734297924));
#35200=CARTESIAN_POINT('Ctrl Pts',(-37.3303369685924,18.2333021834777,-2.93246489517018));
#35201=CARTESIAN_POINT('Ctrl Pts',(-37.3038079847852,18.2175624224805,-2.93410932586751));
#35202=CARTESIAN_POINT('Ctrl Pts',(-37.2981695486083,18.2141223505386,-2.93446831448551));
#35203=CARTESIAN_POINT('Ctrl Pts',(-37.2869979825889,18.2071152324757,-2.93519862167771));
#35204=CARTESIAN_POINT('Ctrl Pts',(-37.2704052709352,18.1964200031032,-2.93631197089007));
#35205=CARTESIAN_POINT('Ctrl Pts',(-37.2328335594255,18.1701812873708,-2.93903307929234));
#35206=CARTESIAN_POINT('Ctrl Pts',(-37.1823616251368,18.1291072193081,-2.94325912074197));
#35207=CARTESIAN_POINT('Ctrl Pts',(-37.1453575126505,18.0924641596172,-2.94698385382838));
#35208=CARTESIAN_POINT('Ctrl Pts',(-37.1188904285929,18.063538924587,-2.94990359739459));
#35209=CARTESIAN_POINT('Ctrl Pts',(-37.1102827811923,18.053656262645,-2.95089791608696));
#35210=CARTESIAN_POINT('Ctrl Pts',(-37.097699635775,18.0384638148773,-2.95242101316685));
#35211=CARTESIAN_POINT('Ctrl Pts',(-37.0935544678788,18.0333310247829,-2.95293470286882));
#35212=CARTESIAN_POINT('Ctrl Pts',(-37.0854130228059,18.0229903050876,-2.95396774156509));
#35213=CARTESIAN_POINT('Ctrl Pts',(-37.0654228154996,17.996938824735,-2.95656569797625));
#35214=CARTESIAN_POINT('Ctrl Pts',(-37.032653758298,17.9482802891913,-2.96137533348098));
#35215=CARTESIAN_POINT('Ctrl Pts',(-36.9956436062314,17.8797286255216,-2.96804918531509));
#35216=CARTESIAN_POINT('Ctrl Pts',(-36.9754354386431,17.8315716900848,-2.97266366864207));
#35217=CARTESIAN_POINT('Ctrl Pts',(-36.9642457335021,17.8006811814676,-2.97559869592517));
#35218=CARTESIAN_POINT('Ctrl Pts',(-36.9620775415684,17.7944555471112,-2.97618899559907));
#35219=CARTESIAN_POINT('Ctrl Pts',(-36.9579096024883,17.7819924669561,-2.97736824178165));
#35220=CARTESIAN_POINT('Ctrl Pts',(-36.9519025588888,17.763262156184,-2.97913679820747));
#35221=CARTESIAN_POINT('Ctrl Pts',(-36.9395867914297,17.7193101856959,-2.98326093492252));
#35222=CARTESIAN_POINT('Ctrl Pts',(-36.9267397851585,17.655829738656,-2.98914315755744));
#35223=CARTESIAN_POINT('Ctrl Pts',(-36.9198258320865,17.5885563906065,-2.99527260942571));
#35224=CARTESIAN_POINT('Ctrl Pts',(-36.918834284911,17.5465615159496,-2.99904690933985));
#35225=CARTESIAN_POINT('Ctrl Pts',(-36.9189421675989,17.5305480457708,-3.00047864028992));
#35226=CARTESIAN_POINT('',(-37.718924746634,16.7373849369936,-3.06578952415236));
#35227=CARTESIAN_POINT('Ctrl Pts',(-36.9189421675989,17.5305480457708,-3.00047864028992));
#35228=CARTESIAN_POINT('Ctrl Pts',(-36.919010575733,17.5203939456227,-3.0013864971935));
#35229=CARTESIAN_POINT('Ctrl Pts',(-36.9192737151562,17.5102114283485,-3.00229389904805));
#35230=CARTESIAN_POINT('Ctrl Pts',(-36.9209227121865,17.4736847569009,-3.00553816871275));
#35231=CARTESIAN_POINT('Ctrl Pts',(-36.9258858078666,17.4215585073783,-3.01012817483868));
#35232=CARTESIAN_POINT('Ctrl Pts',(-36.9408692628969,17.3448391155681,-3.01677274079049));
#35233=CARTESIAN_POINT('Ctrl Pts',(-36.9558799055065,17.2946725283372,-3.02104811851266));
#35234=CARTESIAN_POINT('Ctrl Pts',(-36.96687627967,17.2636336341393,-3.02367300382162));
#35235=CARTESIAN_POINT('Ctrl Pts',(-36.9691537112077,17.257450076958,-3.02419490147982));
#35236=CARTESIAN_POINT('Ctrl Pts',(-36.9738469995823,17.2451764290858,-3.02522882019687));
#35237=CARTESIAN_POINT('Ctrl Pts',(-36.9811011279822,17.2268856044673,-3.02676662512534));
#35238=CARTESIAN_POINT('Ctrl Pts',(-36.9995186272136,17.1850400421649,-3.03026458098281));
#35239=CARTESIAN_POINT('Ctrl Pts',(-37.0300126016223,17.1275979053621,-3.0350126340462));
#35240=CARTESIAN_POINT('Ctrl Pts',(-37.0588378628576,17.084120115963,-3.03855681973285));
#35241=CARTESIAN_POINT('Ctrl Pts',(-37.0782685093995,17.0577375107066,-3.04069395282585));
#35242=CARTESIAN_POINT('Ctrl Pts',(-37.082225544559,17.0525006314761,-3.04111747216896));
#35243=CARTESIAN_POINT('Ctrl Pts',(-37.0902828595418,17.0421069646206,-3.04195670011983));
#35244=CARTESIAN_POINT('Ctrl Pts',(-37.0943866683441,17.0369458657907,-3.04237275563911));
#35245=CARTESIAN_POINT('Ctrl Pts',(-37.1068915748229,17.0216125534472,-3.04360691231197));
#35246=CARTESIAN_POINT('Ctrl Pts',(-37.1325618428275,16.9916896358098,-3.04600756947841));
#35247=CARTESIAN_POINT('Ctrl Pts',(-37.1785652046567,16.9454439267093,-3.04968393967054));
#35248=CARTESIAN_POINT('Ctrl Pts',(-37.2187381548525,16.9122436653894,-3.05229515823886));
#35249=CARTESIAN_POINT('Ctrl Pts',(-37.2501443023646,16.8887815514432,-3.05413229054577));
#35250=CARTESIAN_POINT('Ctrl Pts',(-37.2661669984714,16.8774105933781,-3.05502048390176));
#35251=CARTESIAN_POINT('Ctrl Pts',(-37.2826770037829,16.8665887086542,-3.05586302629121));
#35252=CARTESIAN_POINT('Ctrl Pts',(-37.293793158217,16.8594974852881,-3.05641453576931));
#35253=CARTESIAN_POINT('Ctrl Pts',(-37.2994118352766,16.8560102252891,-3.05668545575409));
#35254=CARTESIAN_POINT('Ctrl Pts',(-37.3276328534854,16.8389747544918,-3.05800757335247));
#35255=CARTESIAN_POINT('Ctrl Pts',(-37.3737884152845,16.8141488770453,-3.0599257099477));
#35256=CARTESIAN_POINT('Ctrl Pts',(-37.4459381546772,16.7839866864414,-3.06224049280731));
#35257=CARTESIAN_POINT('Ctrl Pts',(-37.4959782855394,16.7685872041763,-3.06341603722978));
#35258=CARTESIAN_POINT('Ctrl Pts',(-37.5342560467992,16.7588521398196,-3.06415800376904));
#35259=CARTESIAN_POINT('Ctrl Pts',(-37.5471721285017,16.7559047648012,-3.06438240114302));
#35260=CARTESIAN_POINT('Ctrl Pts',(-37.5729991097878,16.7506789220564,-3.06478000194362));
#35261=CARTESIAN_POINT('Ctrl Pts',(-37.6117937694978,16.7438261426791,-3.06530089754843));
#35262=CARTESIAN_POINT('Ctrl Pts',(-37.6647357792095,16.7384443509895,-3.06570916417531));
#35263=CARTESIAN_POINT('Ctrl Pts',(-37.704858235669,16.737384873758,-3.06578952970039));
#35264=CARTESIAN_POINT('Ctrl Pts',(-37.718924746634,16.7373849369936,-3.06578952415236));
#35265=CARTESIAN_POINT('',(-38.5188998330781,17.5422403127815,-2.99943193326247));
#35266=CARTESIAN_POINT('Ctrl Pts',(-37.718924746634,16.7373849369936,-3.06578952415236));
#35267=CARTESIAN_POINT('Ctrl Pts',(-37.7309724146918,16.7373849911536,-3.06578951940059));
#35268=CARTESIAN_POINT('Ctrl Pts',(-37.7430350373672,16.7376571699563,-3.06576887237064));
#35269=CARTESIAN_POINT('Ctrl Pts',(-37.7682023355023,16.7387953147954,-3.06568253939694));
#35270=CARTESIAN_POINT('Ctrl Pts',(-37.7813096714479,16.7397096923924,-3.0656131746316));
#35271=CARTESIAN_POINT('Ctrl Pts',(-37.8009977508883,16.741573938698,-3.06547168652142));
#35272=CARTESIAN_POINT('Ctrl Pts',(-37.8075737093973,16.7422786005527,-3.06541819715752));
#35273=CARTESIAN_POINT('Ctrl Pts',(-37.8206887979692,16.7438483559608,-3.06529901151748));
#35274=CARTESIAN_POINT('Ctrl Pts',(-37.8533606292976,16.7481717229133,-3.06497067396001));
#35275=CARTESIAN_POINT('Ctrl Pts',(-37.9111453064512,16.7594812532432,-3.06411088374695));
#35276=CARTESIAN_POINT('Ctrl Pts',(-37.9860613887302,16.7818937437651,-3.06240058626652));
#35277=CARTESIAN_POINT('Ctrl Pts',(-38.0345821581833,16.8017347263525,-3.06087864877346));
#35278=CARTESIAN_POINT('Ctrl Pts',(-38.0644485553534,16.8157154672045,-3.05980221395205));
#35279=CARTESIAN_POINT('Ctrl Pts',(-38.0704043083084,16.8185937583215,-3.05958042082917));
#35280=CARTESIAN_POINT('Ctrl Pts',(-38.0822056520277,16.8244781459628,-3.05912657441623));
#35281=CARTESIAN_POINT('Ctrl Pts',(-38.099763863601,16.8335052848071,-3.05842974112173));
#35282=CARTESIAN_POINT('Ctrl Pts',(-38.1397327587973,16.8559635822866,-3.05669137072979));
#35283=CARTESIAN_POINT('Ctrl Pts',(-38.1940302112681,16.8919528132613,-3.05388941931908));
#35284=CARTESIAN_POINT('Ctrl Pts',(-38.2345117085067,16.9248663030074,-3.05130289362264));
#35285=CARTESIAN_POINT('Ctrl Pts',(-38.2637436106773,16.9511255701933,-3.04922757687767));
#35286=CARTESIAN_POINT('Ctrl Pts',(-38.2732990393399,16.9601414846898,-3.0485131908628));
#35287=CARTESIAN_POINT('Ctrl Pts',(-38.2873435899538,16.9740676197577,-3.04740650943474));
#35288=CARTESIAN_POINT('Ctrl Pts',(-38.2919756404014,16.9787758243361,-3.04703183290515));
#35289=CARTESIAN_POINT('Ctrl Pts',(-38.3010915965788,16.9882731695345,-3.04627492659788));
#35290=CARTESIAN_POINT('Ctrl Pts',(-38.3235426877027,17.012252520247,-3.04436110678424));
#35291=CARTESIAN_POINT('Ctrl Pts',(-38.3609567050234,17.0575033826528,-3.04072350743365));
#35292=CARTESIAN_POINT('Ctrl Pts',(-38.4045936810271,17.1221885322085,-3.03545633743746));
#35293=CARTESIAN_POINT('Ctrl Pts',(-38.429500116155,17.1682250232725,-3.03165548589758));
#35294=CARTESIAN_POINT('Ctrl Pts',(-38.4437134661759,17.1979395070246,-3.02918325758975));
#35295=CARTESIAN_POINT('Ctrl Pts',(-38.4464837427162,17.2039205266858,-3.02868471815221));
#35296=CARTESIAN_POINT('Ctrl Pts',(-38.4518595478943,17.2159127295726,-3.02768323259862));
#35297=CARTESIAN_POINT('Ctrl Pts',(-38.4596864613027,17.2339662976765,-3.02617273205817));
#35298=CARTESIAN_POINT('Ctrl Pts',(-38.4763011808142,17.2765454650671,-3.02258998023486));
#35299=CARTESIAN_POINT('Ctrl Pts',(-38.4954157055941,17.3386458788027,-3.01730425152133));
#35300=CARTESIAN_POINT('Ctrl Pts',(-38.5058190053368,17.3896723095994,-3.0128910139563));
#35301=CARTESIAN_POINT('Ctrl Pts',(-38.5117501031248,17.4284572602049,-3.00950811920092));
#35302=CARTESIAN_POINT('Ctrl Pts',(-38.5134146825683,17.4414715854915,-3.00836831081549));
#35303=CARTESIAN_POINT('Ctrl Pts',(-38.5161053987673,17.4676759533342,-3.00606351257013));
#35304=CARTESIAN_POINT('Ctrl Pts',(-38.5171225993645,17.4807801627204,-3.00490606944401));
#35305=CARTESIAN_POINT('Ctrl Pts',(-38.5186672398078,17.5100035515609,-3.0023138950648));
#35306=CARTESIAN_POINT('Ctrl Pts',(-38.5190286374484,17.5261237028805,-3.00087654313128));
#35307=CARTESIAN_POINT('Ctrl Pts',(-38.5189000091045,17.5422403141662,-2.99943193309589));
#35308=CARTESIAN_POINT('',(-38.0645261134423,18.255001868818,-2.93018339529753));
#35309=CARTESIAN_POINT('Ctrl Pts',(-38.5189000091045,17.5422403141662,-2.99943193309589));
#35310=CARTESIAN_POINT('Ctrl Pts',(-38.518819629035,17.5523116117943,-2.99852919384351));
#35311=CARTESIAN_POINT('Ctrl Pts',(-38.5185478927787,17.5623815270316,-2.99762362028695));
#35312=CARTESIAN_POINT('Ctrl Pts',(-38.5174831792733,17.5855404169291,-2.9955341060631));
#35313=CARTESIAN_POINT('Ctrl Pts',(-38.5165576565204,17.5986284329933,-2.99434819030326));
#35314=CARTESIAN_POINT('Ctrl Pts',(-38.5146791299617,17.6182569082276,-2.99256197428916));
#35315=CARTESIAN_POINT('Ctrl Pts',(-38.5139702987777,17.624806343346,-2.99196468640024));
#35316=CARTESIAN_POINT('Ctrl Pts',(-38.5123929064259,17.6378655121742,-2.99077117076634));
#35317=CARTESIAN_POINT('Ctrl Pts',(-38.5080511096546,17.6703979780115,-2.98779152237676));
#35318=CARTESIAN_POINT('Ctrl Pts',(-38.4967136126686,17.727935441958,-2.98246468554883));
#35319=CARTESIAN_POINT('Ctrl Pts',(-38.4742706912444,17.8025288092669,-2.97544207174657));
#35320=CARTESIAN_POINT('Ctrl Pts',(-38.454411593118,17.8508389101167,-2.97081849908883));
#35321=CARTESIAN_POINT('Ctrl Pts',(-38.4404194899548,17.8805751295757,-2.96794982485069));
#35322=CARTESIAN_POINT('Ctrl Pts',(-38.4375384803318,17.8865058429242,-2.967376526089));
#35323=CARTESIAN_POINT('Ctrl Pts',(-38.4316473483778,17.8982598993618,-2.96623805154997));
#35324=CARTESIAN_POINT('Ctrl Pts',(-38.4226095803834,17.9157483563618,-2.96454075450265));
#35325=CARTESIAN_POINT('Ctrl Pts',(-38.40012241695,17.9555624401979,-2.96065368940274));
#35326=CARTESIAN_POINT('Ctrl Pts',(-38.3640776936724,18.0096595981727,-2.95531050337563));
#35327=CARTESIAN_POINT('Ctrl Pts',(-38.3310991261845,18.0500004283726,-2.95126832284971));
#35328=CARTESIAN_POINT('Ctrl Pts',(-38.3047809236703,18.0791333861947,-2.94833016157896));
#35329=CARTESIAN_POINT('Ctrl Pts',(-38.2957436722637,18.0886569280017,-2.94736638630857));
#35330=CARTESIAN_POINT('Ctrl Pts',(-38.2817826469739,18.1026552032221,-2.94594525661301));
#35331=CARTESIAN_POINT('Ctrl Pts',(-38.2770696331703,18.1072649271286,-2.94547649987763));
#35332=CARTESIAN_POINT('Ctrl Pts',(-38.2675578378121,18.1163414658276,-2.94455208056439));
#35333=CARTESIAN_POINT('Ctrl Pts',(-38.2435389562924,18.1386979602117,-2.94227145996936));
#35334=CARTESIAN_POINT('Ctrl Pts',(-38.198184360507,18.1759736987718,-2.93843840821149));
#35335=CARTESIAN_POINT('Ctrl Pts',(-38.1549150551439,18.2049773241328,-2.9354232729364));
#35336=CARTESIAN_POINT('Ctrl Pts',(-38.1213464392414,18.2251692867483,-2.93331492411179));
#35337=CARTESIAN_POINT('Ctrl Pts',(-38.1042825224182,18.2348744500654,-2.93229905812222));
#35338=CARTESIAN_POINT('Ctrl Pts',(-38.0867927304674,18.243984444565,-2.93134241094606));
#35339=CARTESIAN_POINT('Ctrl Pts',(-38.0754919523261,18.2496943815878,-2.93074218958385));
#35340=CARTESIAN_POINT('Ctrl Pts',(-38.0700213262657,18.252380813858,-2.93045951516175));
#35341=CARTESIAN_POINT('Ctrl Pts',(-38.0645262657606,18.2550018687314,-2.93018339473831));
#35342=CARTESIAN_POINT('Ctrl Pts',(-37.718924746634,19.3314643670594,-4.62273145772315));
#35343=CARTESIAN_POINT('Ctrl Pts',(-37.7240432796227,19.3314643670594,-4.62273145772315));
#35344=CARTESIAN_POINT('Ctrl Pts',(-37.729105675728,19.330917508136,-4.62236438057516));
#35345=CARTESIAN_POINT('Ctrl Pts',(-37.7429480950038,19.3279914277147,-4.62039543755766));
#35346=CARTESIAN_POINT('Ctrl Pts',(-37.7511301340406,19.3246331108791,-4.61813211791741));
#35347=CARTESIAN_POINT('Ctrl Pts',(-37.7709118757918,19.3136757017161,-4.6106867021804));
#35348=CARTESIAN_POINT('Ctrl Pts',(-37.7817536948118,19.3044969837231,-4.60439028856606));
#35349=CARTESIAN_POINT('Ctrl Pts',(-37.8119215619376,19.273950159203,-4.58308087636467));
#35350=CARTESIAN_POINT('Ctrl Pts',(-37.8293065757878,19.2470367921451,-4.56367620611464));
#35351=CARTESIAN_POINT('Ctrl Pts',(-37.8842261422008,19.1493119759434,-4.49018612732299));
#35352=CARTESIAN_POINT('Ctrl Pts',(-37.9205683373981,19.0452717254973,-4.40565062734794));
#35353=CARTESIAN_POINT('Ctrl Pts',(-37.9994181115573,18.7553638270197,-4.10740388440347));
#35354=CARTESIAN_POINT('Ctrl Pts',(-38.0314877466367,18.5690397639075,-3.85835872738472));
#35355=CARTESIAN_POINT('Ctrl Pts',(-38.0598088046867,18.3530721778374,-3.36031585786156));
#35356=CARTESIAN_POINT('Ctrl Pts',(-38.0646084270943,18.2960215435642,-3.16946171823003));
#35357=CARTESIAN_POINT('Ctrl Pts',(-38.0646084270943,18.2621718608173,-2.9739074883211));
#35358=CARTESIAN_POINT('Ctrl Pts',(-38.0646084270943,18.2596508721519,-2.95934339326693));
#35359=CARTESIAN_POINT('Ctrl Pts',(-38.0645810063647,18.2572609718871,-2.94476807941075));
#35360=CARTESIAN_POINT('Ctrl Pts',(-38.0645262657607,18.2550018687316,-2.93018339473923));
#35361=CARTESIAN_POINT('',(-37.718924746634,23.3605792411954,-3.81059743858941));
#35362=CARTESIAN_POINT('Origin',(-37.718924746634,21.,-2.5));
#35363=CARTESIAN_POINT('Origin',(-37.718924746634,24.0600101274756,-4.19892260557888));
#35364=CARTESIAN_POINT('Origin',(-17.718924746634,21.,7.));
#35365=CARTESIAN_POINT('',(-17.718924746634,24.1393970581951,7.61982748486642));
#35366=CARTESIAN_POINT('Origin',(-17.718924746634,24.9242463227439,7.77478435608303));
#35367=CARTESIAN_POINT('',(-17.718924746634,17.8056396357716,6.81010093219959));
#35368=CARTESIAN_POINT('Origin',(-17.718924746634,21.,7.));
#35369=CARTESIAN_POINT('',(-18.503934654988,16.8564417728896,6.70366763718318));
#35370=CARTESIAN_POINT('Ctrl Pts',(-17.718924746634,17.8056396357716,6.81010093219959));
#35371=CARTESIAN_POINT('Ctrl Pts',(-17.7437642274753,17.805639936155,6.81010096743885));
#35372=CARTESIAN_POINT('Ctrl Pts',(-17.7945806620485,17.8032736219272,6.80985504288097));
#35373=CARTESIAN_POINT('Ctrl Pts',(-17.8705625761499,17.7924930279374,6.80873329662359));
#35374=CARTESIAN_POINT('Ctrl Pts',(-17.921492828803,17.7801311535749,6.80744359855836));
#35375=CARTESIAN_POINT('Ctrl Pts',(-17.9531061110628,17.7707796265052,6.80646566831214));
#35376=CARTESIAN_POINT('Ctrl Pts',(-17.9594238791357,17.7688257129027,6.80626124067242));
#35377=CARTESIAN_POINT('Ctrl Pts',(-17.9719700525308,17.7647754194567,6.80583724177927));
#35378=CARTESIAN_POINT('Ctrl Pts',(-17.9906772709459,17.7584809008687,6.80517797306814));
#35379=CARTESIAN_POINT('Ctrl Pts',(-18.0335480566535,17.7422697905638,6.80347718720341));
#35380=CARTESIAN_POINT('Ctrl Pts',(-18.0926092393002,17.7148435014562,6.80058915066718));
#35381=CARTESIAN_POINT('Ctrl Pts',(-18.1375535774513,17.6883976114347,6.79778673808222));
#35382=CARTESIAN_POINT('Ctrl Pts',(-18.1703813397044,17.6668424494962,6.7954934838427));
#35383=CARTESIAN_POINT('Ctrl Pts',(-18.1811769170662,17.6593700941287,6.79469709774963));
#35384=CARTESIAN_POINT('Ctrl Pts',(-18.1971452253442,17.6477217806831,6.7934531112477));
#35385=CARTESIAN_POINT('Ctrl Pts',(-18.2024277795054,17.6437672898988,6.79303038089619));
#35386=CARTESIAN_POINT('Ctrl Pts',(-18.2128589038726,17.6357562610639,6.79217313373619));
#35387=CARTESIAN_POINT('Ctrl Pts',(-18.2386372906825,17.6154455326787,6.78999755925242));
#35388=CARTESIAN_POINT('Ctrl Pts',(-18.2823885839682,17.5763805902293,6.78579238930071));
#35389=CARTESIAN_POINT('Ctrl Pts',(-18.335199074135,17.5190716076668,6.77956801624083));
#35390=CARTESIAN_POINT('Ctrl Pts',(-18.3667048102232,17.4773678386001,6.77499525393865));
#35391=CARTESIAN_POINT('Ctrl Pts',(-18.3851987148915,17.4501719281585,6.77199753817605));
#35392=CARTESIAN_POINT('Ctrl Pts',(-18.3888300757025,17.4446866457309,6.77139215707454));
#35393=CARTESIAN_POINT('Ctrl Pts',(-18.3959354367756,17.4336604106349,6.77017369611277));
#35394=CARTESIAN_POINT('Ctrl Pts',(-18.4063691081392,17.4170215549816,6.76833269446205));
#35395=CARTESIAN_POINT('Ctrl Pts',(-18.4291527063757,17.3775050758205,6.76394379344769));
#35396=CARTESIAN_POINT('Ctrl Pts',(-18.4573221090362,17.3191117620688,6.7574088008242));
#35397=CARTESIAN_POINT('Ctrl Pts',(-18.4752252427967,17.2703441070257,6.75189395522156));
#35398=CARTESIAN_POINT('Ctrl Pts',(-18.4868790983566,17.2329825881833,6.74764614586732));
#35399=CARTESIAN_POINT('Ctrl Pts',(-18.4904676066854,17.2203975511552,6.74621156959817));
#35400=CARTESIAN_POINT('Ctrl Pts',(-18.4970395596012,17.1949594180543,6.74330409490759));
#35401=CARTESIAN_POINT('Ctrl Pts',(-18.4999963095876,17.1822091381994,6.74184294570588));
#35402=CARTESIAN_POINT('Ctrl Pts',(-18.5078943414964,17.1438889055983,6.73744002022504));
#35403=CARTESIAN_POINT('Ctrl Pts',(-18.5158427423235,17.0925907201539,6.7315152759013));
#35404=CARTESIAN_POINT('Ctrl Pts',(-18.5187347637249,17.0408921832155,6.72548308130679));
#35405=CARTESIAN_POINT('Ctrl Pts',(-18.5189935253682,17.001967015951,6.72091847384795));
#35406=CARTESIAN_POINT('Ctrl Pts',(-18.5187608417161,16.9889667041771,6.71939018918219));
#35407=CARTESIAN_POINT('Ctrl Pts',(-18.5176482397637,16.9629148154356,6.71632002713026));
#35408=CARTESIAN_POINT('Ctrl Pts',(-18.5167674431033,16.9498537547869,6.71477702649695));
#35409=CARTESIAN_POINT('Ctrl Pts',(-18.5131381950841,16.9106515627424,6.71013447800261));
#35410=CARTESIAN_POINT('Ctrl Pts',(-18.5093031380889,16.8838623643511,6.70694639835343));
#35411=CARTESIAN_POINT('Ctrl Pts',(-18.5041119180302,16.8573391865427,6.70377496037948));
#35412=CARTESIAN_POINT('Ctrl Pts',(-18.5039346585515,16.8564417721916,6.70366763713326));
#35413=CARTESIAN_POINT('',(-17.718924746634,16.2147387265569,6.62413484998572));
#35414=CARTESIAN_POINT('Ctrl Pts',(-18.5039346585515,16.8564417721916,6.70366763713326));
#35415=CARTESIAN_POINT('Ctrl Pts',(-18.4990520338128,16.8317224311244,6.70071141080989));
#35416=CARTESIAN_POINT('Ctrl Pts',(-18.4929900691117,16.8072344206075,6.69776969800538));
#35417=CARTESIAN_POINT('Ctrl Pts',(-18.4838530007988,16.7766971106601,6.69408581848945));
#35418=CARTESIAN_POINT('Ctrl Pts',(-18.481891446972,16.7704267103922,6.69332855080655));
#35419=CARTESIAN_POINT('Ctrl Pts',(-18.4778252926784,16.7579733179017,6.69182295030277));
#35420=CARTESIAN_POINT('Ctrl Pts',(-18.4715061772404,16.7394035120316,6.68957544372212));
#35421=CARTESIAN_POINT('Ctrl Pts',(-18.4552314545873,16.6968413309535,6.68440761131254));
#35422=CARTESIAN_POINT('Ctrl Pts',(-18.4276933217952,16.6381885851568,6.67724190315151));
#35423=CARTESIAN_POINT('Ctrl Pts',(-18.4011288767869,16.5935389735778,6.67174551679615));
#35424=CARTESIAN_POINT('Ctrl Pts',(-18.379470949919,16.5609208580899,6.66771645958401));
#35425=CARTESIAN_POINT('Ctrl Pts',(-18.371962026184,16.5501932599997,6.66638900938586));
#35426=CARTESIAN_POINT('Ctrl Pts',(-18.3563525988859,16.5290344037261,6.6637664185393));
#35427=CARTESIAN_POINT('Ctrl Pts',(-18.3483028175492,16.518672885763,6.66247991996544));
#35428=CARTESIAN_POINT('Ctrl Pts',(-18.3234959875097,16.4883125244316,6.65870444956298));
#35429=CARTESIAN_POINT('Ctrl Pts',(-18.2886161598463,16.4496856970626,6.65388502913153));
#35430=CARTESIAN_POINT('Ctrl Pts',(-18.2502021300267,16.4146892602587,6.64949372875457));
#35431=CARTESIAN_POINT('Ctrl Pts',(-18.2200556979461,16.3898138372835,6.6463649871714));
#35432=CARTESIAN_POINT('Ctrl Pts',(-18.2046479670122,16.3777196541662,6.6448418639455));
#35433=CARTESIAN_POINT('Ctrl Pts',(-18.1887307386623,16.3661486304109,6.64338209528373));
#35434=CARTESIAN_POINT('Ctrl Pts',(-18.1780048436419,16.3585520846253,6.64242320052006));
#35435=CARTESIAN_POINT('Ctrl Pts',(-18.1725777225939,16.3548079090092,6.64195030912558));
#35436=CARTESIAN_POINT('Ctrl Pts',(-18.1452408175762,16.336443365656,6.63962960324257));
#35437=CARTESIAN_POINT('Ctrl Pts',(-18.1003916816812,16.309440410321,6.63620924911408));
#35438=CARTESIAN_POINT('Ctrl Pts',(-18.0298938090306,16.2758481786742,6.63193887289174));
#35439=CARTESIAN_POINT('Ctrl Pts',(-17.9807546607501,16.2580417410788,6.62966864832929));
#35440=CARTESIAN_POINT('Ctrl Pts',(-17.9493568559871,16.2483826473291,6.62843600572121));
#35441=CARTESIAN_POINT('Ctrl Pts',(-17.9430429233677,16.2465244962757,6.62819881007824));
#35442=CARTESIAN_POINT('Ctrl Pts',(-17.9303455620517,16.2429571389029,6.62774332035942));
#35443=CARTESIAN_POINT('Ctrl Pts',(-17.9239586678768,16.2412473003856,6.62752494537815));
#35444=CARTESIAN_POINT('Ctrl Pts',(-17.9047992194454,16.2363691840864,6.62690179590072));
#35445=CARTESIAN_POINT('Ctrl Pts',(-17.8663831007668,16.2275932534501,6.62578012373376));
#35446=CARTESIAN_POINT('Ctrl Pts',(-17.8018815463507,16.2177528554165,6.62452085559388));
#35447=CARTESIAN_POINT('Ctrl Pts',(-17.7497820050364,16.2149044523123,6.62415607053616));
#35448=CARTESIAN_POINT('Ctrl Pts',(-17.7220460714532,16.2147432699944,6.62413543169615));
#35449=CARTESIAN_POINT('Ctrl Pts',(-17.7204856339758,16.2147387305049,6.62413485045537));
#35450=CARTESIAN_POINT('Ctrl Pts',(-17.718924746634,16.2147387265569,6.62413484998572));
#35451=CARTESIAN_POINT('',(-16.9340264357173,17.1635288511797,6.73969634067107));
#35452=CARTESIAN_POINT('Ctrl Pts',(-17.718924746634,16.2147387265569,6.62413484998572));
#35453=CARTESIAN_POINT('Ctrl Pts',(-17.7073901207539,16.2147386973818,6.62413484651512));
#35454=CARTESIAN_POINT('Ctrl Pts',(-17.6958309281618,16.214986349411,6.62416655835217));
#35455=CARTESIAN_POINT('Ctrl Pts',(-17.6710950665175,16.2160521816488,6.62430302504923));
#35456=CARTESIAN_POINT('Ctrl Pts',(-17.6578800967229,16.2169470871587,6.62441760265911));
#35457=CARTESIAN_POINT('Ctrl Pts',(-17.618539737525,16.2205845052797,6.62488321315798));
#35458=CARTESIAN_POINT('Ctrl Pts',(-17.5667062451157,16.2279645901634,6.62582775169573));
#35459=CARTESIAN_POINT('Ctrl Pts',(-17.4907655414855,16.2464159284195,6.62818590268485));
#35460=CARTESIAN_POINT('Ctrl Pts',(-17.4413448027588,16.2636382051738,6.63038235379587));
#35461=CARTESIAN_POINT('Ctrl Pts',(-17.4108450610503,16.275986019519,6.63195461113918));
#35462=CARTESIAN_POINT('Ctrl Pts',(-17.4047573329155,16.2785381347074,6.63227946159647));
#35463=CARTESIAN_POINT('Ctrl Pts',(-17.392656553187,16.2837875791675,6.63294738475772));
#35464=CARTESIAN_POINT('Ctrl Pts',(-17.3746406531229,16.2918680856118,6.63397514809339));
#35465=CARTESIAN_POINT('Ctrl Pts',(-17.333543938793,16.3121571257405,6.63655266849902));
#35466=CARTESIAN_POINT('Ctrl Pts',(-17.2774646495951,16.3451542416341,6.64073395855193));
#35467=CARTESIAN_POINT('Ctrl Pts',(-17.2353718106155,16.37577953871,6.64459834653782));
#35468=CARTESIAN_POINT('Ctrl Pts',(-17.2048581546413,16.4003601492348,6.64769185760752));
#35469=CARTESIAN_POINT('Ctrl Pts',(-17.1948632441005,16.4088227697541,6.64875561975649));
#35470=CARTESIAN_POINT('Ctrl Pts',(-17.1801404493712,16.4219281696642,6.65040072833764));
#35471=CARTESIAN_POINT('Ctrl Pts',(-17.1752713191261,16.4263714613955,6.65095812427235));
#35472=CARTESIAN_POINT('Ctrl Pts',(-17.1656691894842,16.4353539396767,6.65208416112202));
#35473=CARTESIAN_POINT('Ctrl Pts',(-17.1419929093713,16.4580609542231,6.65492876298833));
#35474=CARTESIAN_POINT('Ctrl Pts',(-17.102285326311,16.5011517480721,6.66030848420105));
#35475=CARTESIAN_POINT('Ctrl Pts',(-17.0553941325125,16.5632214156579,6.66800927694668));
#35476=CARTESIAN_POINT('Ctrl Pts',(-17.02817892591,16.6076872190025,6.67348812469957));
#35477=CARTESIAN_POINT('Ctrl Pts',(-17.0124748344788,16.6364744349879,6.67702127116173));
#35478=CARTESIAN_POINT('Ctrl Pts',(-17.0093968359646,16.6422873010984,6.67773402886076));
#35479=CARTESIAN_POINT('Ctrl Pts',(-17.0034052213629,16.6539503720992,6.67916272927562));
#35480=CARTESIAN_POINT('Ctrl Pts',(-16.9946522678938,16.6715209503219,6.6813130134438));
#35481=CARTESIAN_POINT('Ctrl Pts',(-16.9758596752147,16.7130474928295,6.68638011044747));
#35482=CARTESIAN_POINT('Ctrl Pts',(-16.9535805813423,16.7738516553674,6.6937548144664));
#35483=CARTESIAN_POINT('Ctrl Pts',(-16.9405788954198,16.824058627078,6.69979202793982));
#35484=CARTESIAN_POINT('Ctrl Pts',(-16.9326693696693,16.8623113652087,6.7043705098731));
#35485=CARTESIAN_POINT('Ctrl Pts',(-16.9303403635677,16.8751620394352,6.70590511847467));
#35486=CARTESIAN_POINT('Ctrl Pts',(-16.9273175517075,16.8945907808836,6.7082197633061));
#35487=CARTESIAN_POINT('Ctrl Pts',(-16.9263885149695,16.9010931471414,6.70899351049072));
#35488=CARTESIAN_POINT('Ctrl Pts',(-16.9246942153957,16.9141079987304,6.71054035440315));
#35489=CARTESIAN_POINT('Ctrl Pts',(-16.9239281128653,16.9206255601628,6.71131405642648));
#35490=CARTESIAN_POINT('Ctrl Pts',(-16.920503229783,16.9532643609428,6.71518393496801));
#35491=CARTESIAN_POINT('Ctrl Pts',(-16.9176572816504,17.0053713760446,6.72133216615983));
#35492=CARTESIAN_POINT('Ctrl Pts',(-16.9210645020192,17.0831969363472,6.73042420827673));
#35493=CARTESIAN_POINT('Ctrl Pts',(-16.9284495603501,17.1348575716213,6.73639817772183));
#35494=CARTESIAN_POINT('Ctrl Pts',(-16.933645427244,17.161596976226,6.73947417131325));
#35495=CARTESIAN_POINT('Ctrl Pts',(-16.9338350389026,17.1625631269947,6.73958529147372));
#35496=CARTESIAN_POINT('Ctrl Pts',(-16.9340264381954,17.1635288506924,6.739696340638));
#35497=CARTESIAN_POINT('Ctrl Pts',(-16.9340264381954,17.1635288506924,6.739696340638));
#35498=CARTESIAN_POINT('Ctrl Pts',(-16.9351109981369,17.1690011030818,6.74032559831906));
#35499=CARTESIAN_POINT('Ctrl Pts',(-16.9362529571807,17.1744596426592,6.74095257638505));
#35500=CARTESIAN_POINT('Ctrl Pts',(-16.9388568010243,17.186283641671,6.74230919334707));
#35501=CARTESIAN_POINT('Ctrl Pts',(-16.9433081085948,17.2053688483162,6.74449603083134));
#35502=CARTESIAN_POINT('Ctrl Pts',(-16.9552863579889,17.2492826463594,6.74950793438583));
#35503=CARTESIAN_POINT('Ctrl Pts',(-16.9768561553689,17.3102847941397,6.75641516254366));
#35504=CARTESIAN_POINT('Ctrl Pts',(-16.9988177277096,17.3572579116379,6.76167884669307));
#35505=CARTESIAN_POINT('Ctrl Pts',(-17.0170860870797,17.3917891174648,6.76552887059901));
#35506=CARTESIAN_POINT('Ctrl Pts',(-17.0234756011144,17.4031828736261,6.76679589924646));
#35507=CARTESIAN_POINT('Ctrl Pts',(-17.033519120055,17.420094939934,6.76867182765814));
#35508=CARTESIAN_POINT('Ctrl Pts',(-17.036947410201,17.4257086449722,6.76929371066084));
#35509=CARTESIAN_POINT('Ctrl Pts',(-17.0439406736216,17.4368468258563,6.77052603009099));
#35510=CARTESIAN_POINT('Ctrl Pts',(-17.0617383518508,17.464424047629,6.77357320762057));
#35511=CARTESIAN_POINT('Ctrl Pts',(-17.0965584766246,17.5116883613631,6.77876195919935));
#35512=CARTESIAN_POINT('Ctrl Pts',(-17.1313811716546,17.550398225015,6.78297104726967));
#35513=CARTESIAN_POINT('Ctrl Pts',(-17.1589589461814,17.5781840235213,6.78597933669272));
#35514=CARTESIAN_POINT('Ctrl Pts',(-17.1731136118301,17.5917647691345,6.78744629220304));
#35515=CARTESIAN_POINT('Ctrl Pts',(-17.187824895331,17.604870422577,6.78885736137875));
#35516=CARTESIAN_POINT('Ctrl Pts',(-17.197757352162,17.6135008803574,6.78978561002206));
#35517=CARTESIAN_POINT('Ctrl Pts',(-17.2027922558143,17.6177677510881,6.79024403430444));
#35518=CARTESIAN_POINT('Ctrl Pts',(-17.2281606385066,17.6387327999837,6.79249414672339));
#35519=CARTESIAN_POINT('Ctrl Pts',(-17.2700991321529,17.6700274474653,6.79583792030219));
#35520=CARTESIAN_POINT('Ctrl Pts',(-17.3369316643949,17.7104237496203,6.80012224085272));
#35521=CARTESIAN_POINT('Ctrl Pts',(-17.384096505469,17.7330010511229,6.80250132612996));
#35522=CARTESIAN_POINT('Ctrl Pts',(-17.4144120897862,17.7457144101392,6.80383778899833));
#35523=CARTESIAN_POINT('Ctrl Pts',(-17.4205171825721,17.7481870458338,6.80409753968387));
#35524=CARTESIAN_POINT('Ctrl Pts',(-17.4328122755551,17.7529906441943,6.80460184646387));
#35525=CARTESIAN_POINT('Ctrl Pts',(-17.4389911007516,17.7553170440476,6.80484592328607));
#35526=CARTESIAN_POINT('Ctrl Pts',(-17.4575584676089,17.7620489786898,6.80555181272847));
#35527=CARTESIAN_POINT('Ctrl Pts',(-17.4948927783289,17.7745487978019,6.8068607858668));
#35528=CARTESIAN_POINT('Ctrl Pts',(-17.5580921261442,17.7906693688048,6.80854332410195));
#35529=CARTESIAN_POINT('Ctrl Pts',(-17.609677577175,17.7986089778658,6.80936966339988));
#35530=CARTESIAN_POINT('Ctrl Pts',(-17.6487571126183,17.8026771607332,6.80979290243887));
#35531=CARTESIAN_POINT('Ctrl Pts',(-17.6618488145178,17.8037182435059,6.80990116365931));
#35532=CARTESIAN_POINT('Ctrl Pts',(-17.6815859652612,17.8047986328145,6.81001349995407));
#35533=CARTESIAN_POINT('Ctrl Pts',(-17.6881898144631,17.8050787312053,6.81004262041923));
#35534=CARTESIAN_POINT('Ctrl Pts',(-17.7013903129314,17.8054755893881,6.8100838811623));
#35535=CARTESIAN_POINT('Ctrl Pts',(-17.7094380700629,17.8056177510387,6.81009865616776));
#35536=CARTESIAN_POINT('Ctrl Pts',(-17.7174696864885,17.8056396181756,6.81010093013532));
#35537=CARTESIAN_POINT('Ctrl Pts',(-17.718924746634,17.8056396357716,6.81010093219959));
#35538=CARTESIAN_POINT('Origin',(-37.718924746634,24.0015386818685,-0.183979981426689));
#35539=CARTESIAN_POINT('',(-37.718924746634,25.0506850112887,-0.766467731910886));
#35540=CARTESIAN_POINT('Origin',(-37.718924746634,25.7501158975689,-1.15479289890034));
#35541=CARTESIAN_POINT('Origin',(-37.718924746634,24.0015386818685,-0.183979981426689));
#35542=CARTESIAN_POINT('Origin',(-17.718924746634,11.0131091329632,0.793137146317211));
#35543=CARTESIAN_POINT('',(-17.718924746634,24.9441835787041,3.54362161041199));
#35544=CARTESIAN_POINT('Origin',(-17.718924746634,11.0131091329632,0.793137146317211));
#35545=CARTESIAN_POINT('Origin',(-17.718924746634,25.7290328432529,3.6985784816286));
#35546=CARTESIAN_POINT('Origin',(-31.,34.999999994595,6.54998265276524E-10));
#35547=CARTESIAN_POINT('',(-31.,34.999999994595,4.000000000655));
#35548=CARTESIAN_POINT('Origin',(-31.,34.999999994595,6.54998265276524E-10));
#35549=CARTESIAN_POINT('',(-39.,34.999999994595,4.000000000655));
#35550=CARTESIAN_POINT('',(-31.,34.999999994595,4.000000000655));
#35551=CARTESIAN_POINT('Origin',(-39.,34.999999994595,6.54998265276524E-10));
#35552=CARTESIAN_POINT('Origin',(-45.7,34.999999994595,6.54998265276524E-10));
#35553=CARTESIAN_POINT('',(-45.7,34.999999994595,4.000000000655));
#35554=CARTESIAN_POINT('',(-45.7,34.999999994595,-3.999999999345));
#35555=CARTESIAN_POINT('Origin',(-45.7,34.999999994595,6.54998265276524E-10));
#35556=CARTESIAN_POINT('Origin',(-45.7,34.999999994595,6.54998265276524E-10));
#35557=CARTESIAN_POINT('',(-46.,34.999999994595,-3.699999999345));
#35558=CARTESIAN_POINT('',(-45.7,34.999999994595,-3.999999999345));
#35559=CARTESIAN_POINT('Origin',(-46.,34.999999994595,6.54998265276524E-10));
#35560=CARTESIAN_POINT('Origin',(-31.,34.999999994595,6.54998265276524E-10));
#35561=CARTESIAN_POINT('',(-45.5,34.999999994595,4.000000000655));
#35562=CARTESIAN_POINT('',(-45.5,30.999999994595,6.5499951014128E-10));
#35563=CARTESIAN_POINT('Origin',(-45.5,34.999999994595,6.55E-10));
#35564=CARTESIAN_POINT('Origin',(-45.5,34.999999994595,6.55E-10));
#35565=CARTESIAN_POINT('',(-31.,34.999999994595,4.000000000655));
#35566=CARTESIAN_POINT('Origin',(-56.6690017314647,48.5946168001447,-6.3392739254555));
#35567=CARTESIAN_POINT('',(-39.,48.5946168001447,-3.5392739254555));
#35568=CARTESIAN_POINT('',(-39.,45.7946168001447,-6.3392739254555));
#35569=CARTESIAN_POINT('Origin',(-39.,48.5946168001447,-6.3392739254555));
#35570=CARTESIAN_POINT('',(-45.5,45.7946168001447,-6.3392739254555));
#35571=CARTESIAN_POINT('',(-56.6690017314647,45.7946168001447,-6.3392739254555));
#35572=CARTESIAN_POINT('',(-45.5,51.3913318198147,-6.47486558726599));
#35573=CARTESIAN_POINT('Origin',(-45.5,48.5946168001447,-6.3392739254555));
#35574=CARTESIAN_POINT('',(-45.,51.3913318198147,-6.47486558726599));
#35575=CARTESIAN_POINT('',(-45.,51.3913318198147,-6.47486558726599));
#35576=CARTESIAN_POINT('',(-45.,49.0519043965673,-3.57686771815033));
#35577=CARTESIAN_POINT('Origin',(-45.,48.5946168001447,-6.3392739254555));
#35578=CARTESIAN_POINT('',(-44.,48.0109313132992,-3.60078688834068));
#35579=CARTESIAN_POINT('Ctrl Pts',(-45.,49.0519043965673,-3.57686771815035));
#35580=CARTESIAN_POINT('Ctrl Pts',(-45.,48.9957251357862,-3.56756782624327));
#35581=CARTESIAN_POINT('Ctrl Pts',(-44.9951745711715,48.9392147266966,-3.55998370975779));
#35582=CARTESIAN_POINT('Ctrl Pts',(-44.9630876045502,48.7514236666012,-3.5405436690203));
#35583=CARTESIAN_POINT('Ctrl Pts',(-44.9151278102305,48.6247757407979,-3.53708953016471));
#35584=CARTESIAN_POINT('Ctrl Pts',(-44.7751927091309,48.3936711000784,-3.54406290383913));
#35585=CARTESIAN_POINT('Ctrl Pts',(-44.6832058663738,48.2908272034433,-3.55457782983572));
#35586=CARTESIAN_POINT('Ctrl Pts',(-44.4781736557104,48.1357194801071,-3.57614322542986));
#35587=CARTESIAN_POINT('Ctrl Pts',(-44.3689066136297,48.0798168915966,-3.58679425502691));
#35588=CARTESIAN_POINT('Ctrl Pts',(-44.1695174787766,48.022881826187,-3.59816232312806));
#35589=CARTESIAN_POINT('Ctrl Pts',(-44.0850432793417,48.0109313132992,-3.60078688834069));
#35590=CARTESIAN_POINT('Ctrl Pts',(-44.,48.0109313132992,-3.60078688834069));
#35591=CARTESIAN_POINT('',(-43.,48.0109313132992,-3.60078688834069));
#35592=CARTESIAN_POINT('',(-43.5,48.0109313132992,-3.60078688834069));
#35593=CARTESIAN_POINT('',(-42.,49.0519043965673,-3.57686771815033));
#35594=CARTESIAN_POINT('Ctrl Pts',(-43.,48.0109313132992,-3.60078688834069));
#35595=CARTESIAN_POINT('Ctrl Pts',(-42.9691893177197,48.0109313132992,-3.60078688834069));
#35596=CARTESIAN_POINT('Ctrl Pts',(-42.9383039359468,48.0125011261107,-3.60045085699698));
#35597=CARTESIAN_POINT('Ctrl Pts',(-42.7839130068819,48.0283194174735,-3.59710789163843));
#35598=CARTESIAN_POINT('Ctrl Pts',(-42.6652177139826,48.0659731655586,-3.58898860882495));
#35599=CARTESIAN_POINT('Ctrl Pts',(-42.4345634815223,48.1900964691459,-3.56785168328553));
#35600=CARTESIAN_POINT('Ctrl Pts',(-42.3270875778571,48.2807056420326,-3.55483109731437));
#35601=CARTESIAN_POINT('Ctrl Pts',(-42.1572239135169,48.490393491272,-3.53934603484932));
#35602=CARTESIAN_POINT('Ctrl Pts',(-42.0931335275273,48.6071980157876,-3.53651307227344));
#35603=CARTESIAN_POINT('Ctrl Pts',(-42.0177600379801,48.8361031309839,-3.54776238095549));
#35604=CARTESIAN_POINT('Ctrl Pts',(-42.,48.9440345489199,-3.55901098758455));
#35605=CARTESIAN_POINT('Ctrl Pts',(-42.,49.0519043965673,-3.57686771815035));
#35606=CARTESIAN_POINT('',(-42.,50.599158431302,-8.29421966612385));
#35607=CARTESIAN_POINT('Origin',(-42.,48.5946168001447,-6.3392739254555));
#35608=CARTESIAN_POINT('',(-45.,50.599158431302,-8.29421966612386));
#35609=CARTESIAN_POINT('',(-56.6690017314647,50.599158431302,-8.29421966612386));
#35610=CARTESIAN_POINT('',(-45.,50.5871414377259,-8.30646623141651));
#35611=CARTESIAN_POINT('Origin',(-45.,48.5946168001447,-6.3392739254555));
#35612=CARTESIAN_POINT('',(-45.5,50.5871414377259,-8.30646623141651));
#35613=CARTESIAN_POINT('',(-45.,50.5871414377259,-8.30646623141651));
#35614=CARTESIAN_POINT('Origin',(-45.5,48.5946168001447,-6.3392739254555));
#35615=CARTESIAN_POINT('Origin',(-39.,48.5946168001447,-6.3392739254555));
#35616=CARTESIAN_POINT('Origin',(-35.3179607461319,20.7255401693197,-2.54750793782168));
#35617=CARTESIAN_POINT('',(-30.,23.2255401693197,-2.54750793782168));
#35618=CARTESIAN_POINT('Origin',(-30.,20.7255401693197,-2.54750793782168));
#35619=CARTESIAN_POINT('',(-38.5,23.2255401693197,-2.54750793782168));
#35620=CARTESIAN_POINT('',(-35.3179607461319,23.2255401693197,-2.54750793782168));
#35621=CARTESIAN_POINT('',(-38.5,21.2255401693197,-0.0980181950384966));
#35622=CARTESIAN_POINT('Origin',(-38.5,20.7255401693197,-2.54750793782168));
#35623=CARTESIAN_POINT('',(-35.1565965239697,21.2255401693197,-0.0980181950384966));
#35624=CARTESIAN_POINT('',(-35.3179607461319,21.2255401693197,-0.0980181950384966));
#35625=CARTESIAN_POINT('',(-35.1565965239697,20.2255401693197,-0.0980181950385001));
#35626=CARTESIAN_POINT('Ctrl Pts',(-35.1565965239697,21.2255401693197,-0.098018195038502));
#35627=CARTESIAN_POINT('Ctrl Pts',(-35.0760059557493,21.2255401693197,-0.098018195038502));
#35628=CARTESIAN_POINT('Ctrl Pts',(-34.9884055345433,21.2153179188118,-0.0958304096017428));
#35629=CARTESIAN_POINT('Ctrl Pts',(-34.8229201950239,21.1669869100577,-0.0866687028340092));
#35630=CARTESIAN_POINT('Ctrl Pts',(-34.7450786649676,21.1287241345178,-0.0797242857551705));
#35631=CARTESIAN_POINT('Ctrl Pts',(-34.6299180077935,21.0381431963904,-0.0667841517369663));
#35632=CARTESIAN_POINT('Ctrl Pts',(-34.5820250297599,20.9842926662468,-0.0601688196471046));
#35633=CARTESIAN_POINT('Ctrl Pts',(-34.5170648437554,20.8612473945026,-0.0504311897554679));
#35634=CARTESIAN_POINT('Ctrl Pts',(-34.5,20.7920357336245,-0.0475079378216808));
#35635=CARTESIAN_POINT('Ctrl Pts',(-34.5,20.6590446050149,-0.0475079378216808));
#35636=CARTESIAN_POINT('Ctrl Pts',(-34.5170648437554,20.5898329441368,-0.0504311897554679));
#35637=CARTESIAN_POINT('Ctrl Pts',(-34.5820250297599,20.4667876723926,-0.0601688196471046));
#35638=CARTESIAN_POINT('Ctrl Pts',(-34.6299180077935,20.412937142249,-0.0667841517369663));
#35639=CARTESIAN_POINT('Ctrl Pts',(-34.7450786649676,20.3223562041216,-0.0797242857551706));
#35640=CARTESIAN_POINT('Ctrl Pts',(-34.8229201950239,20.2840934285817,-0.0866687028340092));
#35641=CARTESIAN_POINT('Ctrl Pts',(-34.9884055345433,20.2357624198276,-0.0958304096017427));
#35642=CARTESIAN_POINT('Ctrl Pts',(-35.0760059557493,20.2255401693197,-0.0980181950385028));
#35643=CARTESIAN_POINT('Ctrl Pts',(-35.1565965239697,20.2255401693197,-0.0980181950385028));
#35644=CARTESIAN_POINT('',(-38.5,20.2255401693197,-0.0980181950385001));
#35645=CARTESIAN_POINT('',(-35.3179607461319,20.2255401693197,-0.0980181950385001));
#35646=CARTESIAN_POINT('',(-38.5,18.8779263022516,-0.863369286101596));
#35647=CARTESIAN_POINT('Origin',(-38.5,20.7255401693197,-2.54750793782168));
#35648=CARTESIAN_POINT('',(-39.224471181792,18.2255370962949,-2.547507937818));
#35649=CARTESIAN_POINT('Ctrl Pts',(-38.5,18.8779263022516,-0.863369286101596));
#35650=CARTESIAN_POINT('Ctrl Pts',(-38.5,18.8418134627679,-0.902987510492509));
#35651=CARTESIAN_POINT('Ctrl Pts',(-38.5029913583948,18.8074241910345,-0.943268205815897));
#35652=CARTESIAN_POINT('Ctrl Pts',(-38.513756919099,18.741792668973,-1.02517424287596));
#35653=CARTESIAN_POINT('Ctrl Pts',(-38.5215384310811,18.7105519790673,-1.06679926913165));
#35654=CARTESIAN_POINT('Ctrl Pts',(-38.5411026664266,18.651029869407,-1.15141245973054));
#35655=CARTESIAN_POINT('Ctrl Pts',(-38.5528891238843,18.6227492495679,-1.19440046494414));
#35656=CARTESIAN_POINT('Ctrl Pts',(-38.5731607994899,18.5824620218676,-1.25992360068095));
#35657=CARTESIAN_POINT('Ctrl Pts',(-38.5803546854392,18.5693838675296,-1.28194731863795));
#35658=CARTESIAN_POINT('Ctrl Pts',(-38.5955434055275,18.5439521349797,-1.3263088029536));
#35659=CARTESIAN_POINT('Ctrl Pts',(-38.6034889685688,18.5316796196784,-1.34850420543431));
#35660=CARTESIAN_POINT('Ctrl Pts',(-38.6282756681186,18.4961209979196,-1.41515357438277));
#35661=CARTESIAN_POINT('Ctrl Pts',(-38.6460625712208,18.4740906795495,-1.45967140046796));
#35662=CARTESIAN_POINT('Ctrl Pts',(-38.6837385046754,18.4330942498066,-1.54895656553476));
#35663=CARTESIAN_POINT('Ctrl Pts',(-38.7036292324255,18.4141292052936,-1.59372355142654));
#35664=CARTESIAN_POINT('Ctrl Pts',(-38.745211491781,18.3790679312211,-1.68356735179541));
#35665=CARTESIAN_POINT('Ctrl Pts',(-38.788595931521,18.3468763471817,-1.77372069830513));
#35666=CARTESIAN_POINT('Ctrl Pts',(-38.8351353172829,18.3201595782086,-1.86459367854188));
#35667=CARTESIAN_POINT('Ctrl Pts',(-38.8710944633591,18.3021126177066,-1.9330522270599));
#35668=CARTESIAN_POINT('Ctrl Pts',(-38.8832569805968,18.296429086976,-1.95592235061537));
#35669=CARTESIAN_POINT('Ctrl Pts',(-38.9079166969854,18.2857197929667,-2.00176927464294));
#35670=CARTESIAN_POINT('Ctrl Pts',(-38.920357181891,18.2807186421253,-2.0246406900419));
#35671=CARTESIAN_POINT('Ctrl Pts',(-38.9579733632456,18.2667428790988,-2.09310093948371));
#35672=CARTESIAN_POINT('Ctrl Pts',(-39.0089188989727,18.2508425791602,-2.18398462221447));
#35673=CARTESIAN_POINT('Ctrl Pts',(-39.0873223383069,18.2347459403829,-2.3193393269623));
#35674=CARTESIAN_POINT('Ctrl Pts',(-39.1407093081975,18.2289758926703,-2.40904581727342));
#35675=CARTESIAN_POINT('Ctrl Pts',(-39.186472043237,18.2261235988577,-2.48508031520527));
#35676=CARTESIAN_POINT('Ctrl Pts',(-39.2054196067492,18.2255380886718,-2.51631704202074));
#35677=CARTESIAN_POINT('Ctrl Pts',(-39.2244711817888,18.2255371663434,-2.54750793782168));
#35678=CARTESIAN_POINT('',(-39.5,18.2644264063412,-2.9867334444556));
#35679=CARTESIAN_POINT('Ctrl Pts',(-39.2244711817953,18.2255370262464,-2.54750793781432));
#35680=CARTESIAN_POINT('Ctrl Pts',(-39.2589632575303,18.2255356570879,-2.60397760789945));
#35681=CARTESIAN_POINT('Ctrl Pts',(-39.2937962530053,18.2274503724719,-2.66029706465531));
#35682=CARTESIAN_POINT('Ctrl Pts',(-39.3289017777147,18.2312588219439,-2.71650663643555));
#35683=CARTESIAN_POINT('Ctrl Pts',(-39.3298642110874,18.2313632322583,-2.71804764652428));
#35684=CARTESIAN_POINT('Ctrl Pts',(-39.3308268508299,18.2314690702069,-2.71958857350432));
#35685=CARTESIAN_POINT('Ctrl Pts',(-39.331789695751,18.2315763362011,-2.72112941814041));
#35686=CARTESIAN_POINT('Ctrl Pts',(-39.3590347419993,18.2346115778152,-2.76472977626034));
#35687=CARTESIAN_POINT('Ctrl Pts',(-39.3864439213512,18.2387901600934,-2.80826403375964));
#35688=CARTESIAN_POINT('Ctrl Pts',(-39.4139900200143,18.2441217238816,-2.85174879411711));
#35689=CARTESIAN_POINT('Ctrl Pts',(-39.4144915148842,18.2442187885121,-2.85254046282139));
#35690=CARTESIAN_POINT('Ctrl Pts',(-39.414993055187,18.2443162355879,-2.85333211510684));
#35691=CARTESIAN_POINT('Ctrl Pts',(-39.4154946407658,18.2444140652289,-2.85412375107242));
#35692=CARTESIAN_POINT('Ctrl Pts',(-39.4292658612322,18.247100014769,-2.87585841385372));
#35693=CARTESIAN_POINT('Ctrl Pts',(-39.4430712030152,18.2500743365209,-2.89758076757143));
#35694=CARTESIAN_POINT('Ctrl Pts',(-39.4569074113687,18.253339532556,-2.91929283744107));
#35695=CARTESIAN_POINT('Ctrl Pts',(-39.4571637281578,18.2534000205554,-2.91969505515071));
#35696=CARTESIAN_POINT('Ctrl Pts',(-39.4574200555418,18.2534606083965,-2.92009726933075));
#35697=CARTESIAN_POINT('Ctrl Pts',(-39.4576763935003,18.2535212960994,-2.9204994799941));
#35698=CARTESIAN_POINT('Ctrl Pts',(-39.4645930575922,18.2551588079922,-2.9313521686462));
#35699=CARTESIAN_POINT('Ctrl Pts',(-39.4715174189979,18.2568690247549,-2.9422022947352));
#35700=CARTESIAN_POINT('Ctrl Pts',(-39.4784490768014,18.2586523436986,-2.95305011294296));
#35701=CARTESIAN_POINT('Ctrl Pts',(-39.4785795394355,18.2586859080339,-2.95325428270692));
#35702=CARTESIAN_POINT('Ctrl Pts',(-39.4787100046545,18.2587194982663,-2.95345845165321));
#35703=CARTESIAN_POINT('Ctrl Pts',(-39.4788404724558,18.2587531143986,-2.95366261978354));
#35704=CARTESIAN_POINT('Ctrl Pts',(-39.4823049708794,18.2596457717164,-2.95908418861828));
#35705=CARTESIAN_POINT('Ctrl Pts',(-39.4857712218867,18.2605566737303,-2.96450507496648));
#35706=CARTESIAN_POINT('Ctrl Pts',(-39.489239377884,18.2614859299042,-2.96992562828773));
#35707=CARTESIAN_POINT('Ctrl Pts',(-39.4893061499531,18.2615038207827,-2.97002998967213));
#35708=CARTESIAN_POINT('Ctrl Pts',(-39.4893729221599,18.2615217183572,-2.97013435003213));
#35709=CARTESIAN_POINT('Ctrl Pts',(-39.4894396942678,18.2615396225595,-2.97023870899992));
#35710=CARTESIAN_POINT('Ctrl Pts',(-39.4912071593253,18.2620135487691,-2.97300110238481));
#35711=CARTESIAN_POINT('Ctrl Pts',(-39.4929834237806,18.2624945429552,-2.97577637133006));
#35712=CARTESIAN_POINT('Ctrl Pts',(-39.494737563525,18.2629740863298,-2.97851624630382));
#35713=CARTESIAN_POINT('Ctrl Pts',(-39.4964917032695,18.2634536297045,-2.98125612127759));
#35714=CARTESIAN_POINT('Ctrl Pts',(-39.498245849939,18.2639377205127,-2.98399518950415));
#35715=CARTESIAN_POINT('Ctrl Pts',(-39.5,18.2644264063412,-2.98673344445558));
#35716=CARTESIAN_POINT('',(-42.,18.2644264063412,-2.98673344445559));
#35717=CARTESIAN_POINT('',(-35.3179607461319,18.2644264063412,-2.9867334444556));
#35718=CARTESIAN_POINT('',(-42.,19.2255401693197,-4.54750793782168));
#35719=CARTESIAN_POINT('Origin',(-42.,20.7255401693197,-2.54750793782168));
#35720=CARTESIAN_POINT('',(-41.5,20.7255401693197,-5.04750793782167));
#35721=CARTESIAN_POINT('Ctrl Pts',(-42.,19.2255401693197,-4.54750793782168));
#35722=CARTESIAN_POINT('Ctrl Pts',(-42.,19.4186296086203,-4.6923250172971));
#35723=CARTESIAN_POINT('Ctrl Pts',(-41.9306808358121,19.6671490362798,-4.8239338831961));
#35724=CARTESIAN_POINT('Ctrl Pts',(-41.7602708300839,20.1428670310053,-4.99434388892433));
#35725=CARTESIAN_POINT('Ctrl Pts',(-41.6191747972635,20.4590572214339,-5.04750793782168));
#35726=CARTESIAN_POINT('Ctrl Pts',(-41.5,20.7255401693197,-5.04750793782168));
#35727=CARTESIAN_POINT('',(-38.5,20.7255401693197,-5.04750793782167));
#35728=CARTESIAN_POINT('',(-35.3179607461319,20.7255401693197,-5.04750793782167));
#35729=CARTESIAN_POINT('Origin',(-38.5,20.7255401693197,-2.54750793782168));
#35730=CARTESIAN_POINT('Ctrl Pts',(-38.0645258088056,18.2550018689912,-2.93018339641562));
#35731=CARTESIAN_POINT('Ctrl Pts',(-38.0644730720159,18.2528283685745,-2.91615135985618));
#35732=CARTESIAN_POINT('Ctrl Pts',(-38.0627705408083,18.2507930257081,-2.90221536006827));
#35733=CARTESIAN_POINT('Ctrl Pts',(-38.0559345119105,18.2468879595698,-2.87385547063433));
#35734=CARTESIAN_POINT('Ctrl Pts',(-38.0506165440385,18.2450719281466,-2.85969728188328));
#35735=CARTESIAN_POINT('Ctrl Pts',(-38.0297502918864,18.2401419398439,-2.81872937384456));
#35736=CARTESIAN_POINT('Ctrl Pts',(-38.009731245707,18.2377145869542,-2.7947624867808));
#35737=CARTESIAN_POINT('Ctrl Pts',(-37.9545422712628,18.2334031798558,-2.74749017343037));
#35738=CARTESIAN_POINT('Ctrl Pts',(-37.9142901746769,18.2318218020662,-2.72528538397519));
#35739=CARTESIAN_POINT('Ctrl Pts',(-37.8414545038188,18.2302840973431,-2.70167022451812));
#35740=CARTESIAN_POINT('Ctrl Pts',(-37.8150018767136,18.2299373708106,-2.69576579367227));
#35741=CARTESIAN_POINT('Ctrl Pts',(-37.7751190161242,18.2296160821703,-2.6902187720473));
#35742=CARTESIAN_POINT('Ctrl Pts',(-37.7617249415434,18.229542319151,-2.688912786255));
#35743=CARTESIAN_POINT('Ctrl Pts',(-37.7385545523854,18.2294669900933,-2.68757578997696));
#35744=CARTESIAN_POINT('Ctrl Pts',(-37.7287578120477,18.2294512869825,-2.68729453043002));
#35745=CARTESIAN_POINT('Ctrl Pts',(-37.7186850743359,18.2294512549474,-2.68729395839443));
#35746=CARTESIAN_POINT('Ctrl Pts',(-37.7184052938003,18.2294512668884,-2.68729417161882));
#35747=CARTESIAN_POINT('Ctrl Pts',(-37.7082212513325,18.2294521685178,-2.68731027148849));
#35748=CARTESIAN_POINT('Ctrl Pts',(-37.6982616367749,18.229469077187,-2.68761309404929));
#35749=CARTESIAN_POINT('Ctrl Pts',(-37.6745901668933,18.2295488107686,-2.68902760581585));
#35750=CARTESIAN_POINT('Ctrl Pts',(-37.6608510644345,18.2296269718215,-2.69041058653413));
#35751=CARTESIAN_POINT('Ctrl Pts',(-37.6204173711276,18.2299641651506,-2.69621997972945));
#35752=CARTESIAN_POINT('Ctrl Pts',(-37.593882430355,18.2303230840297,-2.7023106862664));
#35753=CARTESIAN_POINT('Ctrl Pts',(-37.5221982448574,18.2318783259906,-2.72607215467));
#35754=CARTESIAN_POINT('Ctrl Pts',(-37.4820604543081,18.2334561001718,-2.7482132333471));
#35755=CARTESIAN_POINT('Ctrl Pts',(-37.4270061886743,18.2378361403167,-2.79598498835417));
#35756=CARTESIAN_POINT('Ctrl Pts',(-37.4072815134747,18.2402743818913,-2.81993098846459));
#35757=CARTESIAN_POINT('Ctrl Pts',(-37.3868559987021,18.2451921415202,-2.86064392007558));
#35758=CARTESIAN_POINT('Ctrl Pts',(-37.3816847042406,18.2469892393911,-2.87461428212165));
#35759=CARTESIAN_POINT('Ctrl Pts',(-37.3750315800499,18.2508476435117,-2.90258940114771));
#35760=CARTESIAN_POINT('Ctrl Pts',(-37.3733738334646,18.2528576526636,-2.91634041908177));
#35761=CARTESIAN_POINT('Ctrl Pts',(-37.3733218817896,18.2550018784108,-2.9301834572279));
#35762=CARTESIAN_POINT('Origin',(-45.5,34.999999994595,6.55E-10));
#35763=CARTESIAN_POINT('',(-46.,30.499999994595,6.5499944890894E-10));
#35764=CARTESIAN_POINT('Origin',(-46.,34.999999994595,6.55E-10));
#35765=CARTESIAN_POINT('Origin',(-45.5,30.499999994595,6.5499944890894E-10));
#35766=CARTESIAN_POINT('Origin',(-42.5,34.999999994595,6.55E-10));
#35767=CARTESIAN_POINT('',(-42.5,44.7486243140984,-3.90055430318255));
#35768=CARTESIAN_POINT('',(-42.5,39.9429588225849,9.26375507215795));
#35769=CARTESIAN_POINT('Origin',(-42.5,34.999999994595,6.55E-10));
#35770=CARTESIAN_POINT('',(-42.,44.4674750811422,-3.21976947643629));
#35771=CARTESIAN_POINT('Ctrl Pts',(-42.5,44.7486243140985,-3.90055430318255));
#35772=CARTESIAN_POINT('Ctrl Pts',(-42.4544360876625,44.7486243140985,-3.90055430318255));
#35773=CARTESIAN_POINT('Ctrl Pts',(-42.4099205589807,44.7452865463964,-3.8921541598089));
#35774=CARTESIAN_POINT('Ctrl Pts',(-42.3189430447185,44.7318256326699,-3.8584039871009));
#35775=CARTESIAN_POINT('Ctrl Pts',(-42.2748783192192,44.7210296796986,-3.83138728482829));
#35776=CARTESIAN_POINT('Ctrl Pts',(-42.1833702395799,44.6900628273989,-3.75439747859195));
#35777=CARTESIAN_POINT('Ctrl Pts',(-42.1405089721587,44.6680439529169,-3.69999801674033));
#35778=CARTESIAN_POINT('Ctrl Pts',(-42.071269518933,44.6190581603652,-3.58027604363302));
#35779=CARTESIAN_POINT('Ctrl Pts',(-42.0453333388043,44.5914650656171,-3.51348614097825));
#35780=CARTESIAN_POINT('Ctrl Pts',(-42.0094486376468,44.5328201717076,-3.37321530750872));
#35781=CARTESIAN_POINT('Ctrl Pts',(-42.0003510591405,44.5011283734183,-3.29830693481085));
#35782=CARTESIAN_POINT('Ctrl Pts',(-42.0000033224979,44.4687146531266,-3.22266128213935));
#35783=CARTESIAN_POINT('Ctrl Pts',(-42.,44.4680949296128,-3.22121534995777));
#35784=CARTESIAN_POINT('Ctrl Pts',(-42.,44.4674750811422,-3.21976947643629));
#35785=CARTESIAN_POINT('',(-42.,40.1687696585666,8.56059695184988));
#35786=CARTESIAN_POINT('Origin',(-42.,34.999999994595,6.55E-10));
#35787=CARTESIAN_POINT('Ctrl Pts',(-42.,40.1687696585666,8.56059695184987));
#35788=CARTESIAN_POINT('Ctrl Pts',(-42.,40.1683075129929,8.56210529777178));
#35789=CARTESIAN_POINT('Ctrl Pts',(-42.0000033223958,40.1678452330699,8.56361360751137));
#35790=CARTESIAN_POINT('Ctrl Pts',(-42.0003519017721,40.1435951711248,8.64271093468089));
#35791=CARTESIAN_POINT('Ctrl Pts',(-42.0094939504562,40.1192631524652,8.72078571814814));
#35792=CARTESIAN_POINT('Ctrl Pts',(-42.0455618257965,40.0731794932059,8.86646140204777));
#35793=CARTESIAN_POINT('Ctrl Pts',(-42.0716251146577,40.0509849747696,8.93559739857092));
#35794=CARTESIAN_POINT('Ctrl Pts',(-42.1410737799586,40.0109460683308,9.05886941152539));
#35795=CARTESIAN_POINT('Ctrl Pts',(-42.1839363914962,39.9926110365693,9.11460125114772));
#35796=CARTESIAN_POINT('Ctrl Pts',(-42.2753727862073,39.9665354166906,9.1932806146181));
#35797=CARTESIAN_POINT('Ctrl Pts',(-42.3193584730603,39.9573371288592,9.22082690969534));
#35798=CARTESIAN_POINT('Ctrl Pts',(-42.4101445564635,39.9458315569623,9.25520747716902));
#35799=CARTESIAN_POINT('Ctrl Pts',(-42.4545481243919,39.9429588225849,9.26375507215796));
#35800=CARTESIAN_POINT('Ctrl Pts',(-42.5,39.9429588225849,9.26375507215796));
#35801=CARTESIAN_POINT('Origin',(-42.5,34.999999994595,6.55E-10));
#35802=CARTESIAN_POINT('',(-42.,41.2631553534218,-1.7386445723384));
#35803=CARTESIAN_POINT('',(-42.,38.6863865866985,5.35355525801058));
#35804=CARTESIAN_POINT('Origin',(-42.,34.999999994595,6.55E-10));
#35805=CARTESIAN_POINT('',(-42.5,40.65404535889,-2.00792704445741));
#35806=CARTESIAN_POINT('Ctrl Pts',(-42.5,40.65404535889,-2.00792704445741));
#35807=CARTESIAN_POINT('Ctrl Pts',(-42.4826491826238,40.65404535889,-2.00792704445741));
#35808=CARTESIAN_POINT('Ctrl Pts',(-42.4652566053828,40.6551721057398,-2.00745307088224));
#35809=CARTESIAN_POINT('Ctrl Pts',(-42.3984104029602,40.6639091994707,-2.00377454682564));
#35810=CARTESIAN_POINT('Ctrl Pts',(-42.3512786216695,40.6793649916246,-1.99726827466977));
#35811=CARTESIAN_POINT('Ctrl Pts',(-42.2553373204744,40.7290519040805,-1.97619081125632));
#35812=CARTESIAN_POINT('Ctrl Pts',(-42.2093703460395,40.7657123920275,-1.96055718697034));
#35813=CARTESIAN_POINT('Ctrl Pts',(-42.1185333929893,40.86385370113,-1.91818900483338));
#35814=CARTESIAN_POINT('Ctrl Pts',(-42.0788703599454,40.9295917118304,-1.88945413699724));
#35815=CARTESIAN_POINT('Ctrl Pts',(-42.0174426176906,41.0817501876172,-1.82174794014236));
#35816=CARTESIAN_POINT('Ctrl Pts',(-42.0004779950668,41.1710675280286,-1.78124834309648));
#35817=CARTESIAN_POINT('Ctrl Pts',(-42.0000033202246,41.2606497333104,-1.73980423753342));
#35818=CARTESIAN_POINT('Ctrl Pts',(-42.,41.2619025742887,-1.73922446906986));
#35819=CARTESIAN_POINT('Ctrl Pts',(-42.,41.2631553534218,-1.7386445723384));
#35820=CARTESIAN_POINT('',(-42.5,38.0494565603535,5.1672831023974));
#35821=CARTESIAN_POINT('Origin',(-42.5,34.999999994595,6.55E-10));
#35822=CARTESIAN_POINT('Ctrl Pts',(-42.,38.6863865866985,5.35355525801058));
#35823=CARTESIAN_POINT('Ctrl Pts',(-42.,38.6850595270089,5.35319169843818));
#35824=CARTESIAN_POINT('Ctrl Pts',(-42.0000033204919,38.6837325023959,5.35282800249168));
#35825=CARTESIAN_POINT('Ctrl Pts',(-42.0004662363704,38.5912113638028,5.32746066601285));
#35826=CARTESIAN_POINT('Ctrl Pts',(-42.0165992209748,38.4995599069129,5.30160691452096));
#35827=CARTESIAN_POINT('Ctrl Pts',(-42.0758441660175,38.3412349144892,5.25577584370346));
#35828=CARTESIAN_POINT('Ctrl Pts',(-42.1151456113167,38.2718504181019,5.23519478871087));
#35829=CARTESIAN_POINT('Ctrl Pts',(-42.2056695167071,38.1682609648624,5.20395060199156));
#35830=CARTESIAN_POINT('Ctrl Pts',(-42.2516602512676,38.1295569539332,5.1920877752668));
#35831=CARTESIAN_POINT('Ctrl Pts',(-42.3477951889101,38.0769631371526,5.17585630236277));
#35832=CARTESIAN_POINT('Ctrl Pts',(-42.3950686181708,38.0605047528529,5.17072674405129));
#35833=CARTESIAN_POINT('Ctrl Pts',(-42.4631644468274,38.0507635189734,5.16769091110134));
#35834=CARTESIAN_POINT('Ctrl Pts',(-42.4816022135789,38.0494565603535,5.1672831023974));
#35835=CARTESIAN_POINT('Ctrl Pts',(-42.5,38.0494565603535,5.1672831023974));
#35836=CARTESIAN_POINT('Origin',(-46.,34.999999994595,6.54998265276524E-10));
#35837=CARTESIAN_POINT('',(-45.,18.0053133249326,0.425000000655));
#35838=CARTESIAN_POINT('',(-45.,51.6342808642875,-3.50723537042861));
#35839=CARTESIAN_POINT('Origin',(-45.,34.999999994595,6.55E-10));
#35840=CARTESIAN_POINT('',(-45.5,51.6342808642875,-3.50723537042861));
#35841=CARTESIAN_POINT('',(-46.,51.6342808642875,-3.50723537042861));
#35842=CARTESIAN_POINT('',(-45.5,18.0053133249326,0.425000000655));
#35843=CARTESIAN_POINT('Origin',(-45.5,34.999999994595,6.54998265276524E-10));
#35844=CARTESIAN_POINT('',(-46.,18.0053133249326,0.425000000655));
#35845=CARTESIAN_POINT('Origin',(-46.,34.999999994595,6.54998265276524E-10));
#35846=CARTESIAN_POINT('',(-39.5,39.2396510906294,16.4628478279264));
#35847=CARTESIAN_POINT('Origin',(-39.5,34.999999994595,6.54998265276524E-10));
#35848=CARTESIAN_POINT('',(-39.,40.8143424311314,15.9747745540155));
#35849=CARTESIAN_POINT('Ctrl Pts',(-39.5,39.2396510906294,16.4628478279264));
#35850=CARTESIAN_POINT('Ctrl Pts',(-39.4999999961656,39.257290636405,16.4583051436736));
#35851=CARTESIAN_POINT('Ctrl Pts',(-39.4997042609893,39.2749148588005,16.4537361753576));
#35852=CARTESIAN_POINT('Ctrl Pts',(-39.4991310319023,39.2925241298331,16.4491409067449));
#35853=CARTESIAN_POINT('Ctrl Pts',(-39.4991304749569,39.2925412388785,16.4491364420138));
#35854=CARTESIAN_POINT('Ctrl Pts',(-39.4991299177479,39.2925583479326,16.4491319772519));
#35855=CARTESIAN_POINT('Ctrl Pts',(-39.4991293602754,39.2925754569952,16.4491275124591));
#35856=CARTESIAN_POINT('Ctrl Pts',(-39.4985550311578,39.3102018547743,16.44452771556));
#35857=CARTESIAN_POINT('Ctrl Pts',(-39.4977016731233,39.3278275737071,16.4398977782837));
#35858=CARTESIAN_POINT('Ctrl Pts',(-39.4965887044839,39.3454033797105,16.4352508177434));
#35859=CARTESIAN_POINT('Ctrl Pts',(-39.4965870036635,39.3454302387686,16.4352437163346));
#35860=CARTESIAN_POINT('Ctrl Pts',(-39.4965853022347,39.3454570977297,16.4352366148808));
#35861=CARTESIAN_POINT('Ctrl Pts',(-39.4965836001976,39.3454839565936,16.435229513382));
#35862=CARTESIAN_POINT('Ctrl Pts',(-39.4943577725402,39.3806084556226,16.4259425760085));
#35863=CARTESIAN_POINT('Ctrl Pts',(-39.4911025840849,39.41548485882,16.4166008352451));
#35864=CARTESIAN_POINT('Ctrl Pts',(-39.4869518406598,39.4501426751304,16.4072005578185));
#35865=CARTESIAN_POINT('Ctrl Pts',(-39.4869357174425,39.450277300533,16.4071640432234));
#35866=CARTESIAN_POINT('Ctrl Pts',(-39.4869195807133,39.4504119226348,16.4071275277457));
#35867=CARTESIAN_POINT('Ctrl Pts',(-39.4869034304803,39.4505465414377,16.4070910113853));
#35868=CARTESIAN_POINT('Ctrl Pts',(-39.4827323057594,39.4853145731815,16.3976599218938));
#35869=CARTESIAN_POINT('Ctrl Pts',(-39.4776595176198,39.5198623488115,16.3881699877856));
#35870=CARTESIAN_POINT('Ctrl Pts',(-39.4717924919497,39.5542134049,16.3786183860195));
#35871=CARTESIAN_POINT('Ctrl Pts',(-39.4659770096339,39.5882626779798,16.369150697572));
#35872=CARTESIAN_POINT('Ctrl Pts',(-39.4593806799903,39.6221185586476,16.3596224420949));
#35873=CARTESIAN_POINT('Ctrl Pts',(-39.4520904807254,39.6557999053799,16.3500314131952));
#35874=CARTESIAN_POINT('Ctrl Pts',(-39.4520300985524,39.656078876205,16.3499519740544));
#35875=CARTESIAN_POINT('Ctrl Pts',(-39.4519696687774,39.6563578350588,16.3498725306069));
#35876=CARTESIAN_POINT('Ctrl Pts',(-39.4519091914498,39.6566367819523,16.3497930828512));
#35877=CARTESIAN_POINT('Ctrl Pts',(-39.4372730555425,39.724144802027,16.3305659080398));
#35878=CARTESIAN_POINT('Ctrl Pts',(-39.4198586838727,39.7909539305682,16.3110863403623));
#35879=CARTESIAN_POINT('Ctrl Pts',(-39.4002375988986,39.8571885237601,16.2913387913687));
#35880=CARTESIAN_POINT('Ctrl Pts',(-39.4001338742578,39.8575386654262,16.2912343981903));
#35881=CARTESIAN_POINT('Ctrl Pts',(-39.4000300879518,39.8578887910394,16.2911299975231));
#35882=CARTESIAN_POINT('Ctrl Pts',(-39.3999262400651,39.8582389006182,16.2910255893649));
#35883=CARTESIAN_POINT('Ctrl Pts',(-39.38030451741,39.9243909743711,16.2712980052008));
#35884=CARTESIAN_POINT('Ctrl Pts',(-39.3584791470918,39.9899694404819,16.2513031922256));
#35885=CARTESIAN_POINT('Ctrl Pts',(-39.3349302503083,40.0550779956201,16.2310254274449));
#35886=CARTESIAN_POINT('Ctrl Pts',(-39.3347975544398,40.0554448763429,16.2309111641045));
#35887=CARTESIAN_POINT('Ctrl Pts',(-39.3346648036945,40.0558117425731,16.2307968916474));
#35888=CARTESIAN_POINT('Ctrl Pts',(-39.3345319981584,40.0561785943288,16.2306826100709));
#35889=CARTESIAN_POINT('Ctrl Pts',(-39.3109717092849,40.1212597166307,16.210408553474));
#35890=CARTESIAN_POINT('Ctrl Pts',(-39.2858005512003,40.1855728622067,16.1899451074169));
#35891=CARTESIAN_POINT('Ctrl Pts',(-39.2594627711653,40.2492934160747,16.1692584430621));
#35892=CARTESIAN_POINT('Ctrl Pts',(-39.2593270376094,40.2496218043196,16.1691518329185));
#35893=CARTESIAN_POINT('Ctrl Pts',(-39.2591912730754,40.2499501768249,16.1690452168479));
#35894=CARTESIAN_POINT('Ctrl Pts',(-39.2590554776243,40.2502785336145,16.1689385948457));
#35895=CARTESIAN_POINT('Ctrl Pts',(-39.2326929533815,40.3140237751508,16.1482396311102));
#35896=CARTESIAN_POINT('Ctrl Pts',(-39.205162121713,40.3771784216706,16.1273164564048));
#35897=CARTESIAN_POINT('Ctrl Pts',(-39.1768657258588,40.4399066591195,16.1061297493681));
#35898=CARTESIAN_POINT('Ctrl Pts',(-39.1767555231826,40.4401509594776,16.1060472359686));
#35899=CARTESIAN_POINT('Ctrl Pts',(-39.1766453088967,40.44039525337,16.1059647185719));
#35900=CARTESIAN_POINT('Ctrl Pts',(-39.1765350830249,40.4406395408063,16.1058821971757));
#35901=CARTESIAN_POINT('Ctrl Pts',(-39.1481971695223,40.5034432739673,16.0846668132485));
#35902=CARTESIAN_POINT('Ctrl Pts',(-39.1190922361285,40.5658197445189,16.0631871765129));
#35903=CARTESIAN_POINT('Ctrl Pts',(-39.0896053781452,40.6279237128273,16.0413987745173));
#35904=CARTESIAN_POINT('Ctrl Pts',(-39.0895425553902,40.6280560274464,16.041352353585));
#35905=CARTESIAN_POINT('Ctrl Pts',(-39.0894797309058,40.6281883408303,16.0413059312506));
#35906=CARTESIAN_POINT('Ctrl Pts',(-39.0894169046956,40.6283206529806,16.0412595075139));
#35907=CARTESIAN_POINT('Ctrl Pts',(-39.0746781404176,40.6593605261092,16.0303686944148));
#35908=CARTESIAN_POINT('Ctrl Pts',(-39.0598441294354,40.6903323484342,16.0194006149621));
#35909=CARTESIAN_POINT('Ctrl Pts',(-39.0449619049029,40.7212548030359,16.0083491790342));
#35910=CARTESIAN_POINT('Ctrl Pts',(-39.0449279153316,40.7213254269518,16.0083239386162));
#35911=CARTESIAN_POINT('Ctrl Pts',(-39.044893925509,40.7213960506103,16.0082986977632));
#35912=CARTESIAN_POINT('Ctrl Pts',(-39.0448599354357,40.7214666740117,16.0082734564755));
#35913=CARTESIAN_POINT('Ctrl Pts',(-39.0374209839921,40.7369230705795,16.0027492343792));
#35914=CARTESIAN_POINT('Ctrl Pts',(-39.0299700122027,40.7523671405465,15.9972041756753));
#35915=CARTESIAN_POINT('Ctrl Pts',(-39.0225129137083,40.7678012106761,15.9916374756535));
#35916=CARTESIAN_POINT('Ctrl Pts',(-39.0224940110446,40.7678403338065,15.9916233648759));
#35917=CARTESIAN_POINT('Ctrl Pts',(-39.0224751082747,40.7678794570111,15.9916092539093));
#35918=CARTESIAN_POINT('Ctrl Pts',(-39.0224562053995,40.7679185802883,15.9915951427543));
#35919=CARTESIAN_POINT('Ctrl Pts',(-39.0187294806157,40.7756317818559,15.9888131114259));
#35920=CARTESIAN_POINT('Ctrl Pts',(-39.0150012674768,40.783342378541,15.9860257341351));
#35921=CARTESIAN_POINT('Ctrl Pts',(-39.0112722413038,40.7910508186585,15.9832328093444));
#35922=CARTESIAN_POINT('Ctrl Pts',(-39.009398270943,40.7949245882802,15.9818292637443));
#35923=CARTESIAN_POINT('Ctrl Pts',(-39.0075241022877,40.7987978000274,15.9804243232044));
#35924=CARTESIAN_POINT('Ctrl Pts',(-39.0056498316341,40.8026704927234,15.979017976295));
#35925=CARTESIAN_POINT('Ctrl Pts',(-39.0047126963073,40.8046068390714,15.9783148028403));
#35926=CARTESIAN_POINT('Ctrl Pts',(-39.0037735239429,40.8065472120575,15.9776097691188));
#35927=CARTESIAN_POINT('Ctrl Pts',(-39.0028301473931,40.8084961158097,15.9769012314385));
#35928=CARTESIAN_POINT('Ctrl Pts',(-39.0018867708432,40.8104450195619,15.9761926937581));
#35929=CARTESIAN_POINT('Ctrl Pts',(-39.000943384461,40.812393789486,15.9754838015716));
#35930=CARTESIAN_POINT('Ctrl Pts',(-39.,40.8143424311314,15.9747745540155));
#35931=CARTESIAN_POINT('',(-39.5,42.3343534352395,15.3364682905745));
#35932=CARTESIAN_POINT('Ctrl Pts',(-39.,40.8143424311314,15.9747745540155));
#35933=CARTESIAN_POINT('Ctrl Pts',(-39.0009433844611,40.8162910727767,15.9740653064594));
#35934=CARTESIAN_POINT('Ctrl Pts',(-39.0018867708433,40.8182395842621,15.9733557042182));
#35935=CARTESIAN_POINT('Ctrl Pts',(-39.002830147393,40.8201879703936,15.9726457443865));
#35936=CARTESIAN_POINT('Ctrl Pts',(-39.0037735239428,40.8221363565251,15.9719357845549));
#35937=CARTESIAN_POINT('Ctrl Pts',(-39.004712696307,40.8240759554092,15.9712286240058));
#35938=CARTESIAN_POINT('Ctrl Pts',(-39.0056498316338,40.8260112739532,15.9705226266828));
#35939=CARTESIAN_POINT('Ctrl Pts',(-39.0075241022874,40.8298819110412,15.9691106320367));
#35940=CARTESIAN_POINT('Ctrl Pts',(-39.0093982709428,40.8337520417486,15.9676972264094));
#35941=CARTESIAN_POINT('Ctrl Pts',(-39.0112722413036,40.8376217031625,15.9662823936014));
#35942=CARTESIAN_POINT('Ctrl Pts',(-39.0150012674767,40.8453219683299,15.9634670083199));
#35943=CARTESIAN_POINT('Ctrl Pts',(-39.0187294806157,40.8530203196596,15.9606459871919));
#35944=CARTESIAN_POINT('Ctrl Pts',(-39.0224562053995,40.8607172301268,15.957819196433));
#35945=CARTESIAN_POINT('Ctrl Pts',(-39.0224751082747,40.8607562707715,15.957804858247));
#35946=CARTESIAN_POINT('Ctrl Pts',(-39.0224940110446,40.8607953112395,15.9577905199634));
#35947=CARTESIAN_POINT('Ctrl Pts',(-39.0225129137083,40.8608343515291,15.9577761815826));
#35948=CARTESIAN_POINT('Ctrl Pts',(-39.0299700122027,40.8762357409875,15.9521196921546));
#35949=CARTESIAN_POINT('Ctrl Pts',(-39.0374209839922,40.8916308799947,15.9464401967435));
#35950=CARTESIAN_POINT('Ctrl Pts',(-39.0448599354357,40.9070220682127,15.9407368161787));
#35951=CARTESIAN_POINT('Ctrl Pts',(-39.0448939255091,40.9070923936639,15.9407107562796));
#35952=CARTESIAN_POINT('Ctrl Pts',(-39.0449279153317,40.9071627190326,15.9406846958821));
#35953=CARTESIAN_POINT('Ctrl Pts',(-39.0449619049029,40.907233044319,15.9406586349859));
#35954=CARTESIAN_POINT('Ctrl Pts',(-39.0598441294354,40.9380247449178,15.9292479553879));
#35955=CARTESIAN_POINT('Ctrl Pts',(-39.0746781404176,40.9688006828774,15.9177416880645));
#35956=CARTESIAN_POINT('Ctrl Pts',(-39.0894169046956,40.9995790849222,15.9061324890668));
#35957=CARTESIAN_POINT('Ctrl Pts',(-39.0894797309058,40.9997102825124,15.9060830031016));
#35958=CARTESIAN_POINT('Ctrl Pts',(-39.0895425553903,40.9998414801463,15.906033515269));
#35959=CARTESIAN_POINT('Ctrl Pts',(-39.0896053781452,40.9999726778251,15.9059840255685));
#35960=CARTESIAN_POINT('Ctrl Pts',(-39.1190922361287,41.061552392481,15.8827552485007));
#35961=CARTESIAN_POINT('Ctrl Pts',(-39.1481971695226,41.1231423854826,15.8591147824557));
#35962=CARTESIAN_POINT('Ctrl Pts',(-39.1765350830251,41.1848898222009,15.8349972479038));
#35963=CARTESIAN_POINT('Ctrl Pts',(-39.1766453088969,41.185130000965,15.8349034380236));
#35964=CARTESIAN_POINT('Ctrl Pts',(-39.1767555231828,41.1853701821039,15.8348096209297));
#35965=CARTESIAN_POINT('Ctrl Pts',(-39.176865725859,41.1856103656265,15.8347157966176));
#35966=CARTESIAN_POINT('Ctrl Pts',(-39.205162121713,41.2472815361242,15.8106248220014));
#35967=CARTESIAN_POINT('Ctrl Pts',(-39.2326929533814,41.3091099596038,15.7860578794398));
#35968=CARTESIAN_POINT('Ctrl Pts',(-39.2590554776243,41.3712466850805,15.7609395541517));
#35969=CARTESIAN_POINT('Ctrl Pts',(-39.2591912730753,41.3715667562765,15.760810167668));
#35970=CARTESIAN_POINT('Ctrl Pts',(-39.2593270376093,41.3718868356986,15.7606807665387));
#35971=CARTESIAN_POINT('Ctrl Pts',(-39.2594627711653,41.3722069233682,15.7605513507518));
#35972=CARTESIAN_POINT('Ctrl Pts',(-39.2858005512002,41.4343168311042,15.7354394725188));
#35973=CARTESIAN_POINT('Ctrl Pts',(-39.3109717092848,41.4967372084691,15.7097756885417));
#35974=CARTESIAN_POINT('Ctrl Pts',(-39.3345319981583,41.5596241529389,15.683473177897));
#35975=CARTESIAN_POINT('Ctrl Pts',(-39.3346648036944,41.5599786364693,15.6833249149005));
#35976=CARTESIAN_POINT('Ctrl Pts',(-39.3347975544398,41.560333125226,15.683176635614));
#35977=CARTESIAN_POINT('Ctrl Pts',(-39.3349302503083,41.5606876192244,15.6830283400282));
#35978=CARTESIAN_POINT('Ctrl Pts',(-39.3584791470918,41.6235979620406,15.6567110365299));
#35979=CARTESIAN_POINT('Ctrl Pts',(-39.3803045174101,41.6866863996315,15.6298749264226));
#35980=CARTESIAN_POINT('Ctrl Pts',(-39.3999262400652,41.7500424748004,15.6024653992843));
#35981=CARTESIAN_POINT('Ctrl Pts',(-39.4000300879518,41.7503777865682,15.6023203344744));
#35982=CARTESIAN_POINT('Ctrl Pts',(-39.4001338742579,41.7507131058039,15.6021752536193));
#35983=CARTESIAN_POINT('Ctrl Pts',(-39.4002375988987,41.7510484325233,15.6020301567089));
#35984=CARTESIAN_POINT('Ctrl Pts',(-39.4198586838727,41.8144805543948,15.5745828810443));
#35985=CARTESIAN_POINT('Ctrl Pts',(-39.4372730555425,41.8781805408086,15.5465610155777));
#35986=CARTESIAN_POINT('Ctrl Pts',(-39.4519091914498,41.9422536741908,15.5178965671404));
#35987=CARTESIAN_POINT('Ctrl Pts',(-39.4519696687774,41.9425184279414,15.5177781240452));
#35988=CARTESIAN_POINT('Ctrl Pts',(-39.4520300985524,41.9427831880851,15.5176596699619));
#35989=CARTESIAN_POINT('Ctrl Pts',(-39.4520904807254,41.9430479546309,15.5175412048844));
#35990=CARTESIAN_POINT('Ctrl Pts',(-39.4593806799903,41.9750143576728,15.5032384069197));
#35991=CARTESIAN_POINT('Ctrl Pts',(-39.465977009634,42.0070741114877,15.4887753334725));
#35992=CARTESIAN_POINT('Ctrl Pts',(-39.4717924919497,42.0392430807491,15.4741415527422));
#35993=CARTESIAN_POINT('Ctrl Pts',(-39.4776595176198,42.071697167649,15.4593780709647));
#35994=CARTESIAN_POINT('Ctrl Pts',(-39.4827323057594,42.1042623112539,15.4444409001366));
#35995=CARTESIAN_POINT('Ctrl Pts',(-39.4869034304802,42.1369583562403,15.4293170738161));
#35996=CARTESIAN_POINT('Ctrl Pts',(-39.4869195807133,42.1370849524904,15.4292585156725));
#35997=CARTESIAN_POINT('Ctrl Pts',(-39.4869357174425,42.1372115507001,15.4291999547321));
#35998=CARTESIAN_POINT('Ctrl Pts',(-39.4869518406598,42.137338150871,15.4291413909941));
#35999=CARTESIAN_POINT('Ctrl Pts',(-39.4911025840849,42.1699299603236,15.4140648063774));
#36000=CARTESIAN_POINT('Ctrl Pts',(-39.4943577725402,42.2026515904045,15.3988028751326));
#36001=CARTESIAN_POINT('Ctrl Pts',(-39.4965836001976,42.2355280459786,15.383339489129));
#36002=CARTESIAN_POINT('Ctrl Pts',(-39.4965853022347,42.2355531858175,15.3833276646477));
#36003=CARTESIAN_POINT('Ctrl Pts',(-39.4965870036635,42.235578325702,15.3833158400695));
#36004=CARTESIAN_POINT('Ctrl Pts',(-39.4965887044839,42.2356034656319,15.3833040153944));
#36005=CARTESIAN_POINT('Ctrl Pts',(-39.4977016731233,42.2520543228121,15.3755662833645));
#36006=CARTESIAN_POINT('Ctrl Pts',(-39.4985550311578,42.2685324731713,15.3677834273452));
#36007=CARTESIAN_POINT('Ctrl Pts',(-39.4991293602754,42.284991769696,15.3599770461034));
#36008=CARTESIAN_POINT('Ctrl Pts',(-39.4991299177479,42.2850077459118,15.3599694688396));
#36009=CARTESIAN_POINT('Ctrl Pts',(-39.4991304749569,42.2850237221012,15.3599618915577));
#36010=CARTESIAN_POINT('Ctrl Pts',(-39.4991310319023,42.2850396982641,15.3599543142578));
#36011=CARTESIAN_POINT('Ctrl Pts',(-39.4997042609893,42.3014829642135,15.3521554730077));
#36012=CARTESIAN_POINT('Ctrl Pts',(-39.4999999961656,42.3179207780666,15.3443268740108));
#36013=CARTESIAN_POINT('Ctrl Pts',(-39.5,42.3343534352395,15.3364682905744));
#36014=CARTESIAN_POINT('',(-39.5000000131726,51.3840964769944,4.53446620038969));
#36015=CARTESIAN_POINT('Origin',(-39.5,34.999999994595,6.54998265276524E-10));
#36016=CARTESIAN_POINT('',(-39.0362682345593,51.6364368368602,3.49699430910377));
#36017=CARTESIAN_POINT('Ctrl Pts',(-39.5,51.3840964378613,4.5344662027289));
#36018=CARTESIAN_POINT('Ctrl Pts',(-39.4968435532909,51.3872502998287,4.52307055518404));
#36019=CARTESIAN_POINT('Ctrl Pts',(-39.4936766092617,51.3903962860629,4.51165705063485));
#36020=CARTESIAN_POINT('Ctrl Pts',(-39.4904960460761,51.3935276966917,4.50024993600152));
#36021=CARTESIAN_POINT('Ctrl Pts',(-39.4873154828905,51.3966591073206,4.48884282136819));
#36022=CARTESIAN_POINT('Ctrl Pts',(-39.4841222891727,51.3997773936769,4.47743687379982));
#36023=CARTESIAN_POINT('Ctrl Pts',(-39.4809141689974,51.4028823781766,4.46603286107936));
#36024=CARTESIAN_POINT('Ctrl Pts',(-39.4744979286469,51.4090923471758,4.44322483563845));
#36025=CARTESIAN_POINT('Ctrl Pts',(-39.4680219824665,51.4152491017619,4.42042454768003));
#36026=CARTESIAN_POINT('Ctrl Pts',(-39.4614661068467,51.4213511333313,4.39763877371537));
#36027=CARTESIAN_POINT('Ctrl Pts',(-39.448354355607,51.4335551964702,4.35206722578608));
#36028=CARTESIAN_POINT('Ctrl Pts',(-39.4349262143165,51.4455405254189,4.30655259604968));
#36029=CARTESIAN_POINT('Ctrl Pts',(-39.4209875904999,51.4572936361253,4.26116017089597));
#36030=CARTESIAN_POINT('Ctrl Pts',(-39.4070489666834,51.4690467468316,4.21576774574225));
#36031=CARTESIAN_POINT('Ctrl Pts',(-39.3926019608065,51.4805677623338,4.17049681288467));
#36032=CARTESIAN_POINT('Ctrl Pts',(-39.3773863627455,51.4918399213891,4.12543522969451));
#36033=CARTESIAN_POINT('Ctrl Pts',(-39.3621707646845,51.5031120804444,4.08037364650435));
#36034=CARTESIAN_POINT('Ctrl Pts',(-39.3461896001512,51.5141355464633,4.0355203834572));
#36035=CARTESIAN_POINT('Ctrl Pts',(-39.329078342351,51.524888139763,3.99099884676946));
#36036=CARTESIAN_POINT('Ctrl Pts',(-39.3119670845507,51.5356407330627,3.94647731008172));
#36037=CARTESIAN_POINT('Ctrl Pts',(-39.2937299545982,51.546122664982,3.90228605929807));
#36038=CARTESIAN_POINT('Ctrl Pts',(-39.2738440874327,51.5563035390082,3.85860246077594));
#36039=CARTESIAN_POINT('Ctrl Pts',(-39.2639011538499,51.5613939760213,3.83676066151488));
#36040=CARTESIAN_POINT('Ctrl Pts',(-39.2535431996943,51.5664090022314,3.81504674210773));
#36041=CARTESIAN_POINT('Ctrl Pts',(-39.2426841573976,51.5713437578886,3.79348993457491));
#36042=CARTESIAN_POINT('Ctrl Pts',(-39.2372546362493,51.5738111357172,3.7827115308085));
#36043=CARTESIAN_POINT('Ctrl Pts',(-39.2316948510857,51.5762604415035,3.77196362852963));
#36044=CARTESIAN_POINT('Ctrl Pts',(-39.2260082601485,51.5786842720526,3.76128005249661));
#36045=CARTESIAN_POINT('Ctrl Pts',(-39.2203216692112,51.5811081026017,3.75059647646359));
#36046=CARTESIAN_POINT('Ctrl Pts',(-39.2145161338205,51.5835032245596,3.73999156307459));
#36047=CARTESIAN_POINT('Ctrl Pts',(-39.2085825697722,51.5858687263796,3.7294716002265));
#36048=CARTESIAN_POINT('Ctrl Pts',(-39.1848483135789,51.5953307336594,3.68739174883414));
#36049=CARTESIAN_POINT('Ctrl Pts',(-39.1590761421985,51.6043196023881,3.64666374823141));
#36050=CARTESIAN_POINT('Ctrl Pts',(-39.1306063976789,51.612771528083,3.60774472224096));
#36051=CARTESIAN_POINT('Ctrl Pts',(-39.1163715254191,51.6169974909304,3.58828520924573));
#36052=CARTESIAN_POINT('Ctrl Pts',(-39.1014603874055,51.6210890945102,3.56927925006868));
#36053=CARTESIAN_POINT('Ctrl Pts',(-39.0857737045518,51.6250368411351,3.55079566517632));
#36054=CARTESIAN_POINT('Ctrl Pts',(-39.0700870216981,51.6289845877601,3.53231208028396));
#36055=CARTESIAN_POINT('Ctrl Pts',(-39.0536247940042,51.632788472119,3.51435086854871));
#36056=CARTESIAN_POINT('Ctrl Pts',(-39.0362682345593,51.6364368368601,3.49699430910376));
#36057=CARTESIAN_POINT('',(-36.5,51.9728313851128,0.960726074544506));
#36058=CARTESIAN_POINT('Origin',(-35.5392739279158,35.0000000067947,2.46239528767234E-9));
#36059=CARTESIAN_POINT('',(-39.9010326004531,51.9728313851128,0.960726074544506));
#36060=CARTESIAN_POINT('',(-46.,51.9728313851128,0.960726074544506));
#36061=CARTESIAN_POINT('',(-40.9999916854184,51.9933713732604,0.474687473337844));
#36062=CARTESIAN_POINT('Ctrl Pts',(-39.9010326004531,51.9728313851129,0.960726074543242));
#36063=CARTESIAN_POINT('Ctrl Pts',(-39.9978786264107,51.9728313941464,0.960725914951945));
#36064=CARTESIAN_POINT('Ctrl Pts',(-40.0944034219574,51.9736959398618,0.945675215530035));
#36065=CARTESIAN_POINT('Ctrl Pts',(-40.2911429224183,51.976606028045,0.891986910632592));
#36066=CARTESIAN_POINT('Ctrl Pts',(-40.3906299377519,51.9787441069525,0.851223271414997));
#36067=CARTESIAN_POINT('Ctrl Pts',(-40.6662405913416,51.9853228295072,0.71209955870285));
#36068=CARTESIAN_POINT('Ctrl Pts',(-40.8325948331438,51.9899804626179,0.595396525128735));
#36069=CARTESIAN_POINT('Ctrl Pts',(-40.9974247789548,51.993320696534,0.476500092965129));
#36070=CARTESIAN_POINT('Ctrl Pts',(-40.9980817464721,51.9933332259892,0.476051023380418));
#36071=CARTESIAN_POINT('Ctrl Pts',(-40.9999833699879,51.9933713149156,0.474687475140312));
#36072=CARTESIAN_POINT('',(-41.,51.6274934940962,-3.5392739254555));
#36073=CARTESIAN_POINT('Origin',(-41.,34.999999994595,6.54998265276524E-10));
#36074=CARTESIAN_POINT('',(-39.,51.6274934940962,-3.5392739254555));
#36075=CARTESIAN_POINT('',(-46.,51.6274934940962,-3.5392739254555));
#36076=CARTESIAN_POINT('',(-39.,51.5380870962865,-3.93594652043317));
#36077=CARTESIAN_POINT('Origin',(-39.,34.999999994595,6.54998265276524E-10));
#36078=CARTESIAN_POINT('',(-42.,51.5380870962865,-3.93594652043317));
#36079=CARTESIAN_POINT('',(-42.5,51.5380870962865,-3.93594652043317));
#36080=CARTESIAN_POINT('Origin',(-42.,34.999999994595,6.55E-10));
#36081=CARTESIAN_POINT('Origin',(-45.5,48.5946168001447,-6.3392739254555));
#36082=CARTESIAN_POINT('',(-45.5,51.536059602328,-8.74508236369084));
#36083=CARTESIAN_POINT('Ctrl Pts',(-45.5,51.536059602328,-8.74508236369081));
#36084=CARTESIAN_POINT('Ctrl Pts',(-45.5610099545588,51.536059602328,-8.74508236369081));
#36085=CARTESIAN_POINT('Ctrl Pts',(-45.6327520230047,51.5228098390117,-8.73895795786099));
#36086=CARTESIAN_POINT('Ctrl Pts',(-45.7461170544744,51.4793988730731,-8.71889221279613));
#36087=CARTESIAN_POINT('Ctrl Pts',(-45.807537611249,51.4412292854533,-8.70124917726702));
#36088=CARTESIAN_POINT('Ctrl Pts',(-45.8953862936685,51.359854656071,-8.66363558050352));
#36089=CARTESIAN_POINT('Ctrl Pts',(-45.9369188502267,51.3018827723886,-8.63683937789094));
#36090=CARTESIAN_POINT('Ctrl Pts',(-45.9852418633363,51.193700420265,-8.58683451273094));
#36091=CARTESIAN_POINT('Ctrl Pts',(-46.,51.1240450977077,-8.5546379026205));
#36092=CARTESIAN_POINT('Ctrl Pts',(-46.,51.0054363441836,-8.49981366733315));
#36093=CARTESIAN_POINT('Ctrl Pts',(-45.9850887852051,50.9353323591387,-8.46740967305372));
#36094=CARTESIAN_POINT('Ctrl Pts',(-45.9365990223064,50.8258060489551,-8.41678359343263));
#36095=CARTESIAN_POINT('Ctrl Pts',(-45.8947712520246,50.7667016000801,-8.3894638879693));
#36096=CARTESIAN_POINT('Ctrl Pts',(-45.8065209977524,50.6837579493857,-8.35112504630582));
#36097=CARTESIAN_POINT('Ctrl Pts',(-45.7450048833574,50.644733012828,-8.3330866449202));
#36098=CARTESIAN_POINT('Ctrl Pts',(-45.6318339315503,50.6006225310584,-8.31269756435638));
#36099=CARTESIAN_POINT('Ctrl Pts',(-45.5606209586284,50.5871414377259,-8.30646623141648));
#36100=CARTESIAN_POINT('Ctrl Pts',(-45.5,50.5871414377259,-8.30646623141648));
#36101=CARTESIAN_POINT('',(-45.5,44.9368005344369,-5.30952630282035));
#36102=CARTESIAN_POINT('Origin',(-45.5,48.5946168001447,-6.3392739254555));
#36103=CARTESIAN_POINT('',(-46.,45.5585549887889,-5.04608844857037));
#36104=CARTESIAN_POINT('Ctrl Pts',(-46.,45.5585549887888,-5.04608844857035));
#36105=CARTESIAN_POINT('Ctrl Pts',(-46.,45.5571993022191,-5.04661049288134));
#36106=CARTESIAN_POINT('Ctrl Pts',(-45.9999967384478,45.5558437328877,-5.04713284993456));
#36107=CARTESIAN_POINT('Ctrl Pts',(-45.9996861771746,45.4913559119876,-5.07199968453559));
#36108=CARTESIAN_POINT('Ctrl Pts',(-45.9922970303438,45.4282529161658,-5.09712381602786));
#36109=CARTESIAN_POINT('Ctrl Pts',(-45.9628850855617,45.3094004254328,-5.14578236294185));
#36110=CARTESIAN_POINT('Ctrl Pts',(-45.9415281874646,45.2530369118137,-5.16949794189751));
#36111=CARTESIAN_POINT('Ctrl Pts',(-45.880111346903,45.1423569962183,-5.21706799128967));
#36112=CARTESIAN_POINT('Ctrl Pts',(-45.8380939739815,45.0887664804345,-5.24073487943443));
#36113=CARTESIAN_POINT('Ctrl Pts',(-45.7448590805052,45.0100882393425,-5.27600141359422));
#36114=CARTESIAN_POINT('Ctrl Pts',(-45.6978771986565,44.9818172501111,-5.28888307601759));
#36115=CARTESIAN_POINT('Ctrl Pts',(-45.5993681166238,44.9458077969971,-5.30536483849589));
#36116=CARTESIAN_POINT('Ctrl Pts',(-45.5501909035189,44.9368005344368,-5.30952630282034));
#36117=CARTESIAN_POINT('Ctrl Pts',(-45.5,44.9368005344368,-5.30952630282034));
#36118=CARTESIAN_POINT('',(-46.,51.3570957323555,-4.53408414344039));
#36119=CARTESIAN_POINT('Origin',(-46.,48.5946168001447,-6.3392739254555));
#36120=CARTESIAN_POINT('',(-46.,51.8936061016832,-6.25760637783006));
#36121=CARTESIAN_POINT('Origin',(-46.,48.5946168001447,-6.3392739254555));
#36122=CARTESIAN_POINT('Ctrl Pts',(-46.,51.8936061016832,-6.25760637783005));
#36123=CARTESIAN_POINT('Ctrl Pts',(-46.,51.8446981440034,-6.29759574004589));
#36124=CARTESIAN_POINT('Ctrl Pts',(-45.9925616565093,51.7945463220741,-6.33085249730313));
#36125=CARTESIAN_POINT('Ctrl Pts',(-45.9600599922931,51.6903418761989,-6.38858294994055));
#36126=CARTESIAN_POINT('Ctrl Pts',(-45.9330606613793,51.6362874460005,-6.41168372569964));
#36127=CARTESIAN_POINT('Ctrl Pts',(-45.8593582686235,51.5403124425339,-6.44478611383869));
#36128=CARTESIAN_POINT('Ctrl Pts',(-45.8153923054053,51.4997330114652,-6.45498930021723));
#36129=CARTESIAN_POINT('Ctrl Pts',(-45.7122950951514,51.4348321270486,-6.46872532783377));
#36130=CARTESIAN_POINT('Ctrl Pts',(-45.6542008350173,51.4118321455977,-6.47201663128939));
#36131=CARTESIAN_POINT('Ctrl Pts',(-45.5624520001501,51.394281159716,-6.47449009821175));
#36132=CARTESIAN_POINT('Ctrl Pts',(-45.5312249071534,51.3913318198146,-6.47486558726599));
#36133=CARTESIAN_POINT('Ctrl Pts',(-45.5,51.3913318198146,-6.47486558726599));
#36134=CARTESIAN_POINT('Origin',(-33.5,53.0946168001448,0.460726074544506));
#36135=CARTESIAN_POINT('',(-33.5,49.0946168001448,0.960726074544506));
#36136=CARTESIAN_POINT('',(-33.5,57.0946168001448,0.960726074544506));
#36137=CARTESIAN_POINT('Origin',(-33.5,53.0946168001448,0.960726074544506));
#36138=CARTESIAN_POINT('',(-33.5,48.5946168001447,0.460726074544507));
#36139=CARTESIAN_POINT('Origin',(-33.5,49.0946168001448,0.460726074544506));
#36140=CARTESIAN_POINT('',(-33.5,57.5946168001448,0.460726074544506));
#36141=CARTESIAN_POINT('Origin',(-33.5,53.0946168001448,0.460726074544507));
#36142=CARTESIAN_POINT('Origin',(-33.5,57.0946168001448,0.460726074544506));
#36143=CARTESIAN_POINT('Origin',(-30.,20.7255401693197,-2.54750793782168));
#36144=CARTESIAN_POINT('',(-29.,22.2255401693197,-2.54750793782168));
#36145=CARTESIAN_POINT('Origin',(-30.,22.2255401693197,-2.54750793782168));
#36146=CARTESIAN_POINT('Origin',(-29.,20.7255401693197,-2.54750793782168));
#36147=CARTESIAN_POINT('Origin',(-33.5,53.0946168001448,-7.02582898583051));
#36148=CARTESIAN_POINT('',(-32.,53.0946168001448,0.960726074544506));
#36149=CARTESIAN_POINT('Origin',(-33.5,53.0946168001448,0.960726074544506));
#36150=CARTESIAN_POINT('',(-32.,53.0946168001448,-3.5392739254555));
#36151=CARTESIAN_POINT('',(-32.,53.0946168001448,-7.02582898583051));
#36152=CARTESIAN_POINT('Origin',(-33.5,53.0946168001448,-3.5392739254555));
#36153=CARTESIAN_POINT('Origin',(-39.,48.5946168001447,-6.3392739254555));
#36154=CARTESIAN_POINT('',(-42.,51.508884771774,-8.77792974158369));
#36155=CARTESIAN_POINT('Origin',(-42.,48.5946168001447,-6.3392739254555));
#36156=CARTESIAN_POINT('',(-39.,45.925692710035,-9.04424050588343));
#36157=CARTESIAN_POINT('Origin',(-39.,48.5946168001447,-6.3392739254555));
#36158=CARTESIAN_POINT('',(-40.9828862029043,45.925692710035,-9.04424050588343));
#36159=CARTESIAN_POINT('',(-35.3179607461319,45.925692710035,-9.04424050588343));
#36160=CARTESIAN_POINT('',(-42.5,45.3322472608192,-8.28784904304297));
#36161=CARTESIAN_POINT('Ctrl Pts',(-40.9828862029043,45.9256927107335,-9.04424050517556));
#36162=CARTESIAN_POINT('Ctrl Pts',(-41.0173448936212,45.9443390811737,-9.06263841535526));
#36163=CARTESIAN_POINT('Ctrl Pts',(-41.053116758968,45.9615485000311,-9.07923938046472));
#36164=CARTESIAN_POINT('Ctrl Pts',(-41.0903148592313,45.9770857982912,-9.09400285120051));
#36165=CARTESIAN_POINT('Ctrl Pts',(-41.093443851758,45.9783927491784,-9.09524471003936));
#36166=CARTESIAN_POINT('Ctrl Pts',(-41.0965829780637,45.9796878314774,-9.09647352116651));
#36167=CARTESIAN_POINT('Ctrl Pts',(-41.0997323690468,45.980970846619,-9.09768919971767));
#36168=CARTESIAN_POINT('Ctrl Pts',(-41.1175783684503,45.9882410418966,-9.10457783273117));
#36169=CARTESIAN_POINT('Ctrl Pts',(-41.1357530721898,45.995124204242,-9.11104526644371));
#36170=CARTESIAN_POINT('Ctrl Pts',(-41.1542768365912,46.0015853108649,-9.11707659944144));
#36171=CARTESIAN_POINT('Ctrl Pts',(-41.156818842632,46.0024719649871,-9.11790427596452));
#36172=CARTESIAN_POINT('Ctrl Pts',(-41.1593674315456,46.0033506623359,-9.11872373054841));
#36173=CARTESIAN_POINT('Ctrl Pts',(-41.1619226753163,46.004221294345,-9.11953490665145));
#36174=CARTESIAN_POINT('Ctrl Pts',(-41.1704135486274,46.0071143357743,-9.1222303807988));
#36175=CARTESIAN_POINT('Ctrl Pts',(-41.1789781331318,46.0099185180234,-9.12483463091471));
#36176=CARTESIAN_POINT('Ctrl Pts',(-41.1876175255668,46.012629587761,-9.12734530816554));
#36177=CARTESIAN_POINT('Ctrl Pts',(-41.1897510659709,46.0132990997512,-9.12796533224672));
#36178=CARTESIAN_POINT('Ctrl Pts',(-41.1918897775883,46.0139630703871,-9.12857977397601));
#36179=CARTESIAN_POINT('Ctrl Pts',(-41.1940327772883,46.0146211955286,-9.12918837786116));
#36180=CARTESIAN_POINT('Ctrl Pts',(-41.1994431252239,46.0162827384585,-9.13072489640275));
#36181=CARTESIAN_POINT('Ctrl Pts',(-41.2048875125716,46.0179089567826,-9.13222599105199));
#36182=CARTESIAN_POINT('Ctrl Pts',(-41.2103433164833,46.01949241214,-9.13368519234456));
#36183=CARTESIAN_POINT('Ctrl Pts',(-41.2141730168133,46.0206039182724,-9.13470947836403));
#36184=CARTESIAN_POINT('Ctrl Pts',(-41.2180113408301,46.0216952045486,-9.1357139077503));
#36185=CARTESIAN_POINT('Ctrl Pts',(-41.2218548938735,46.0227649655191,-9.13669740800758));
#36186=CARTESIAN_POINT('Ctrl Pts',(-41.2234868793636,46.0232191896087,-9.13711500550951));
#36187=CARTESIAN_POINT('Ctrl Pts',(-41.2251202992978,46.023669717826,-9.13752900998855));
#36188=CARTESIAN_POINT('Ctrl Pts',(-41.2267552532063,46.0241165597052,-9.13793943857175));
#36189=CARTESIAN_POINT('Ctrl Pts',(-41.2706392371279,46.0361102934392,-9.14895579888199));
#36190=CARTESIAN_POINT('Ctrl Pts',(-41.3154708392568,46.0454052275782,-9.15735727293221));
#36191=CARTESIAN_POINT('Ctrl Pts',(-41.3613242473302,46.0517061076808,-9.16303121925624));
#36192=CARTESIAN_POINT('Ctrl Pts',(-41.3622325672626,46.0518309231575,-9.16314361566815));
#36193=CARTESIAN_POINT('Ctrl Pts',(-41.363141287959,46.0519545639161,-9.16325494161169));
#36194=CARTESIAN_POINT('Ctrl Pts',(-41.3640504097949,46.0520770278875,-9.16336519637614));
#36195=CARTESIAN_POINT('Ctrl Pts',(-41.3746147603127,46.0535001070264,-9.16464639976599));
#36196=CARTESIAN_POINT('Ctrl Pts',(-41.3852336299998,46.0547636322353,-9.16578203782526));
#36197=CARTESIAN_POINT('Ctrl Pts',(-41.3959082607259,46.0558632218831,-9.16676933263137));
#36198=CARTESIAN_POINT('Ctrl Pts',(-41.3975829399649,46.0560357299541,-9.1669242234334));
#36199=CARTESIAN_POINT('Ctrl Pts',(-41.3992586918721,46.0562041719286,-9.16707543505593));
#36200=CARTESIAN_POINT('Ctrl Pts',(-41.400935632367,46.0563685454413,-9.16722296981535));
#36201=CARTESIAN_POINT('Ctrl Pts',(-41.4050631402276,46.056773123283,-9.16758610188894));
#36202=CARTESIAN_POINT('Ctrl Pts',(-41.4092022420157,46.0571532335852,-9.16792712030245));
#36203=CARTESIAN_POINT('Ctrl Pts',(-41.4133477595884,46.0575084263247,-9.16824566991062));
#36204=CARTESIAN_POINT('Ctrl Pts',(-41.4191775347142,46.058007928199,-9.16869364113485));
#36205=CARTESIAN_POINT('Ctrl Pts',(-41.4250298031295,46.0584589035442,-9.16909785059445));
#36206=CARTESIAN_POINT('Ctrl Pts',(-41.4308719865823,46.0588582722967,-9.16945566965012));
#36207=CARTESIAN_POINT('Ctrl Pts',(-41.4333568786799,46.0590281382834,-9.16960786304682));
#36208=CARTESIAN_POINT('Ctrl Pts',(-41.4358415456161,46.0591888251255,-9.16975180467935));
#36209=CARTESIAN_POINT('Ctrl Pts',(-41.4383245331774,46.0593401770602,-9.16988736505531));
#36210=CARTESIAN_POINT('Ctrl Pts',(-41.4591923685483,46.0606121879659,-9.17102665856302));
#36211=CARTESIAN_POINT('Ctrl Pts',(-41.4799966113902,46.0612348057782,-9.17158334235594));
#36212=CARTESIAN_POINT('Ctrl Pts',(-41.5007378023747,46.0612196712951,-9.17156968029259));
#36213=CARTESIAN_POINT('Ctrl Pts',(-41.5047693863103,46.0612167295191,-9.17156702471919));
#36214=CARTESIAN_POINT('Ctrl Pts',(-41.5087985900968,46.0611896836042,-9.17154281273808));
#36215=CARTESIAN_POINT('Ctrl Pts',(-41.5128254233789,46.0611386323799,-9.17149714643567));
#36216=CARTESIAN_POINT('Ctrl Pts',(-41.5551621119526,46.0606018980201,-9.1710170272234));
#36217=CARTESIAN_POINT('Ctrl Pts',(-41.597237127505,46.0574150733128,-9.16817483501116));
#36218=CARTESIAN_POINT('Ctrl Pts',(-41.6390554803649,46.0516537176579,-9.16298455103823));
#36219=CARTESIAN_POINT('Ctrl Pts',(-41.6459705250399,46.0507010251434,-9.16212629041595));
#36220=CARTESIAN_POINT('Ctrl Pts',(-41.6528785212426,46.0496776586956,-9.16120357316154));
#36221=CARTESIAN_POINT('Ctrl Pts',(-41.6597795012171,46.0485840352099,-9.16021652676587));
#36222=CARTESIAN_POINT('Ctrl Pts',(-41.6643042060876,46.0478669887136,-9.15956935873315));
#36223=CARTESIAN_POINT('Ctrl Pts',(-41.6688258813008,46.0471196804026,-9.15889438348601));
#36224=CARTESIAN_POINT('Ctrl Pts',(-41.6733445308942,46.0463421899949,-9.15819153918479));
#36225=CARTESIAN_POINT('Ctrl Pts',(-41.6748835466363,46.0460773830096,-9.15795215606347));
#36226=CARTESIAN_POINT('Ctrl Pts',(-41.6764221541904,46.0458090855128,-9.1577095497241));
#36227=CARTESIAN_POINT('Ctrl Pts',(-41.6779604238888,46.0455372875763,-9.15746370590037));
#36228=CARTESIAN_POINT('Ctrl Pts',(-41.6840106761485,46.0444682643214,-9.15649676417899));
#36229=CARTESIAN_POINT('Ctrl Pts',(-41.6900641690809,46.0433433592062,-9.1554781681718));
#36230=CARTESIAN_POINT('Ctrl Pts',(-41.6960827237929,46.0421703401118,-9.15441460909197));
#36231=CARTESIAN_POINT('Ctrl Pts',(-41.6998790708115,46.0414304303237,-9.15374374382032));
#36232=CARTESIAN_POINT('Ctrl Pts',(-41.7036636983394,46.0406710582769,-9.15305470289116));
#36233=CARTESIAN_POINT('Ctrl Pts',(-41.7074378395222,46.0398922878319,-9.15234745459851));
#36234=CARTESIAN_POINT('Ctrl Pts',(-41.7155936736881,46.0382093824253,-9.15081910695343));
#36235=CARTESIAN_POINT('Ctrl Pts',(-41.72369729212,46.0364364941332,-9.14920628329334));
#36236=CARTESIAN_POINT('Ctrl Pts',(-41.7317501971088,46.0345766419165,-9.14751080796047));
#36237=CARTESIAN_POINT('Ctrl Pts',(-41.7459701129861,46.0312924926432,-9.14451691735341));
#36238=CARTESIAN_POINT('Ctrl Pts',(-41.7600321613098,46.0277375113706,-9.14126567927191));
#36239=CARTESIAN_POINT('Ctrl Pts',(-41.7739425547014,46.0239257273487,-9.13776416316361));
#36240=CARTESIAN_POINT('Ctrl Pts',(-41.7829275571194,46.0214636195068,-9.13550246359741));
#36241=CARTESIAN_POINT('Ctrl Pts',(-41.7918493634354,46.0188942453244,-9.13313622688385));
#36242=CARTESIAN_POINT('Ctrl Pts',(-41.8007097354328,46.0162214790045,-9.13066740684117));
#36243=CARTESIAN_POINT('Ctrl Pts',(-41.8231045987492,46.0094659797514,-9.12442738808974));
#36244=CARTESIAN_POINT('Ctrl Pts',(-41.8451065966985,46.0020494043586,-9.1175315624867));
#36245=CARTESIAN_POINT('Ctrl Pts',(-41.8667342232812,45.9940222828129,-9.1099973249351));
#36246=CARTESIAN_POINT('Ctrl Pts',(-41.877486866624,45.9900314253456,-9.10625151542884));
#36247=CARTESIAN_POINT('Ctrl Pts',(-41.8881468432435,45.9858895015613,-9.10234771278249));
#36248=CARTESIAN_POINT('Ctrl Pts',(-41.8987157309372,45.9816019214929,-9.09828701783937));
#36249=CARTESIAN_POINT('Ctrl Pts',(-41.8992684305478,45.9813777026439,-9.09807466393998));
#36250=CARTESIAN_POINT('Ctrl Pts',(-41.8998209127248,45.9811530714684,-9.0978618675743));
#36251=CARTESIAN_POINT('Ctrl Pts',(-41.9003731723471,45.9809280309924,-9.0976486310334));
#36252=CARTESIAN_POINT('Ctrl Pts',(-41.9054678885501,45.9788519832191,-9.09568147715134));
#36253=CARTESIAN_POINT('Ctrl Pts',(-41.9105415297137,45.9767419774063,-9.09367769460556));
#36254=CARTESIAN_POINT('Ctrl Pts',(-41.9155943505303,45.9745986307123,-9.09163740977237));
#36255=CARTESIAN_POINT('Ctrl Pts',(-41.920428408595,45.9725480805845,-9.08968545942426));
#36256=CARTESIAN_POINT('Ctrl Pts',(-41.9252467388496,45.9704655358539,-9.08769868451621));
#36257=CARTESIAN_POINT('Ctrl Pts',(-41.9300373853927,45.9683566610691,-9.0856820673569));
#36258=CARTESIAN_POINT('Ctrl Pts',(-41.9302541835792,45.9682612250513,-9.08559080640934));
#36259=CARTESIAN_POINT('Ctrl Pts',(-41.9304709087346,45.9681657434396,-9.0854994922948));
#36260=CARTESIAN_POINT('Ctrl Pts',(-41.9306875601532,45.9680702166347,-9.08540812536772));
#36261=CARTESIAN_POINT('Ctrl Pts',(-41.9406956697401,45.9636574011657,-9.08118747348054));
#36262=CARTESIAN_POINT('Ctrl Pts',(-41.9505663499056,45.9591375950147,-9.076844031651));
#36263=CARTESIAN_POINT('Ctrl Pts',(-41.9603058228263,45.9545177334838,-9.07238130366819));
#36264=CARTESIAN_POINT('Ctrl Pts',(-41.9797847686677,45.945278010422,-9.06345584770257));
#36265=CARTESIAN_POINT('Ctrl Pts',(-41.9987389093858,45.9356380219542,-9.05405328598334));
#36266=CARTESIAN_POINT('Ctrl Pts',(-42.0172051609414,45.9256425922258,-9.04419084073549));
#36267=CARTESIAN_POINT('Ctrl Pts',(-42.0270287387187,45.920325276957,-9.03894426983965));
#36268=CARTESIAN_POINT('Ctrl Pts',(-42.0367132025377,45.914906801506,-9.03356697121349));
#36269=CARTESIAN_POINT('Ctrl Pts',(-42.0462652696518,45.9093943753032,-9.02806185483883));
#36270=CARTESIAN_POINT('Ctrl Pts',(-42.0726249402372,45.8941824073494,-9.01287005892311));
#36271=CARTESIAN_POINT('Ctrl Pts',(-42.0979709345613,45.8782510965609,-8.99670208157806));
#36272=CARTESIAN_POINT('Ctrl Pts',(-42.1223609992132,45.8616940208704,-8.9795641926535));
#36273=CARTESIAN_POINT('Ctrl Pts',(-42.1313706154958,45.8555778870732,-8.97323350820027));
#36274=CARTESIAN_POINT('Ctrl Pts',(-42.1402490867898,45.8493758516663,-8.96676990574525));
#36275=CARTESIAN_POINT('Ctrl Pts',(-42.1489996451523,45.8430926072868,-8.96017350691971));
#36276=CARTESIAN_POINT('Ctrl Pts',(-42.1563855691804,45.8377892239237,-8.95460580500096));
#36277=CARTESIAN_POINT('Ctrl Pts',(-42.163679614432,45.8324274898817,-8.94894301025735));
#36278=CARTESIAN_POINT('Ctrl Pts',(-42.1708825098498,45.8270094521259,-8.94318436310254));
#36279=CARTESIAN_POINT('Ctrl Pts',(-42.1715164970955,45.826532565175,-8.94267749626121));
#36280=CARTESIAN_POINT('Ctrl Pts',(-42.1721497892792,45.8260552345097,-8.94216987881008));
#36281=CARTESIAN_POINT('Ctrl Pts',(-42.1727823839537,45.8255774636144,-8.94166151241245));
#36282=CARTESIAN_POINT('Ctrl Pts',(-42.1800008105882,45.8201257039106,-8.93586063280913));
#36283=CARTESIAN_POINT('Ctrl Pts',(-42.1871355609368,45.8146106227731,-8.92995567082541));
#36284=CARTESIAN_POINT('Ctrl Pts',(-42.1941438037635,45.8090689774266,-8.92398344742641));
#36285=CARTESIAN_POINT('Ctrl Pts',(-42.1947012737151,45.8086281678201,-8.92350838753319));
#36286=CARTESIAN_POINT('Ctrl Pts',(-42.1952579602536,45.8081871725404,-8.92303288316482));
#36287=CARTESIAN_POINT('Ctrl Pts',(-42.1958138432048,45.8077460097417,-8.92255695245784));
#36288=CARTESIAN_POINT('Ctrl Pts',(-42.202858678639,45.8021550497934,-8.91652537062681));
#36289=CARTESIAN_POINT('Ctrl Pts',(-42.2097822113911,45.7965317839233,-8.9104196370166));
#36290=CARTESIAN_POINT('Ctrl Pts',(-42.2165862799542,45.7908805491703,-8.90424233881281));
#36291=CARTESIAN_POINT('Ctrl Pts',(-42.2242882910079,45.7844835130251,-8.89724981388376));
#36292=CARTESIAN_POINT('Ctrl Pts',(-42.2318368229378,45.7780494925984,-8.89016435004907));
#36293=CARTESIAN_POINT('Ctrl Pts',(-42.2392360579893,45.7715817007783,-8.8829863360389));
#36294=CARTESIAN_POINT('Ctrl Pts',(-42.2600463073129,45.7533911230477,-8.86279826792616));
#36295=CARTESIAN_POINT('Ctrl Pts',(-42.279680437653,45.7349349810326,-8.84187997974338));
#36296=CARTESIAN_POINT('Ctrl Pts',(-42.2981779437348,45.7162661626306,-8.82022080225078));
#36297=CARTESIAN_POINT('Ctrl Pts',(-42.3042442450087,45.7101436790723,-8.81311762329066));
#36298=CARTESIAN_POINT('Ctrl Pts',(-42.3101877355428,45.7039981411622,-8.80593453369296));
#36299=CARTESIAN_POINT('Ctrl Pts',(-42.3160100276813,45.6978313537452,-8.79867102180722));
#36300=CARTESIAN_POINT('Ctrl Pts',(-42.3342535775375,45.6785083635863,-8.7759115590276));
#36301=CARTESIAN_POINT('Ctrl Pts',(-42.3513057904162,45.6589759364203,-8.75236245922885));
#36302=CARTESIAN_POINT('Ctrl Pts',(-42.3671510448732,45.639270031241,-8.72798189773159));
#36303=CARTESIAN_POINT('Ctrl Pts',(-42.3715615707197,45.6337848934441,-8.7211955695645));
#36304=CARTESIAN_POINT('Ctrl Pts',(-42.3758781640535,45.6282861677551,-8.71434461824596));
#36305=CARTESIAN_POINT('Ctrl Pts',(-42.3801005365623,45.6227745982512,-8.70742804354935));
#36306=CARTESIAN_POINT('Ctrl Pts',(-42.3858833948021,45.6152260873007,-8.69795527180989));
#36307=CARTESIAN_POINT('Ctrl Pts',(-42.391488806919,45.6076532830732,-8.68835912959438));
#36308=CARTESIAN_POINT('Ctrl Pts',(-42.396913432122,45.6000574580988,-8.67863589617369));
#36309=CARTESIAN_POINT('Ctrl Pts',(-42.4005109005079,45.5950201072796,-8.67218770417322));
#36310=CARTESIAN_POINT('Ctrl Pts',(-42.4040280633186,45.5899737539531,-8.66568507158052));
#36311=CARTESIAN_POINT('Ctrl Pts',(-42.4074661359585,45.5849153351961,-8.65912243169166));
#36312=CARTESIAN_POINT('Ctrl Pts',(-42.4085128559495,45.5833753014067,-8.65712443831429));
#36313=CARTESIAN_POINT('Ctrl Pts',(-42.4095518863119,45.5818346257886,-8.6551214860273));
#36314=CARTESIAN_POINT('Ctrl Pts',(-42.4105830246306,45.5802936100937,-8.65311393995478));
#36315=CARTESIAN_POINT('Ctrl Pts',(-42.4137820536097,45.5755127249539,-8.64688567945247));
#36316=CARTESIAN_POINT('Ctrl Pts',(-42.4168989413963,45.5707374091497,-8.64062475253282));
#36317=CARTESIAN_POINT('Ctrl Pts',(-42.4199303687472,45.5659741019819,-8.63433893692391));
#36318=CARTESIAN_POINT('Ctrl Pts',(-42.4210855056866,45.5641590256413,-8.63194370294227));
#36319=CARTESIAN_POINT('Ctrl Pts',(-42.4222286704019,45.5623450452855,-8.62954401310694));
#36320=CARTESIAN_POINT('Ctrl Pts',(-42.4233600795134,45.5605318737104,-8.62713945024177));
#36321=CARTESIAN_POINT('Ctrl Pts',(-42.4261468114457,45.5560659178722,-8.62121686039213));
#36322=CARTESIAN_POINT('Ctrl Pts',(-42.4288602395602,45.5516073585664,-8.61526800567393));
#36323=CARTESIAN_POINT('Ctrl Pts',(-42.4315004765197,45.5471564369526,-8.60929272158343));
#36324=CARTESIAN_POINT('Ctrl Pts',(-42.4444002629478,45.5254099274124,-8.58009841448179));
#36325=CARTESIAN_POINT('Ctrl Pts',(-42.4555601676492,45.5038462446935,-8.55027435752416));
#36326=CARTESIAN_POINT('Ctrl Pts',(-42.4649412712655,45.4824896513182,-8.51979328516327));
#36327=CARTESIAN_POINT('Ctrl Pts',(-42.4663006213825,45.4793950167323,-8.5153764861409));
#36328=CARTESIAN_POINT('Ctrl Pts',(-42.4676225398243,45.4763047255679,-8.51094588086722));
#36329=CARTESIAN_POINT('Ctrl Pts',(-42.4689069078218,45.4732188423179,-8.50650136826789));
#36330=CARTESIAN_POINT('Ctrl Pts',(-42.4783003261938,45.4506497714042,-8.4739957574255));
#36331=CARTESIAN_POINT('Ctrl Pts',(-42.4856862257662,45.4283162396088,-8.44074673253793));
#36332=CARTESIAN_POINT('Ctrl Pts',(-42.4909152369877,45.4062381526062,-8.40669784041856));
#36333=CARTESIAN_POINT('Ctrl Pts',(-42.4912865460965,45.4046704002222,-8.40428004798091));
#36334=CARTESIAN_POINT('Ctrl Pts',(-42.4916469287141,45.4031039305286,-8.40185821169987));
#36335=CARTESIAN_POINT('Ctrl Pts',(-42.4919963320089,45.4015387505793,-8.39943230999391));
#36336=CARTESIAN_POINT('Ctrl Pts',(-42.4930452550499,45.3968400160896,-8.39214965344062));
#36337=CARTESIAN_POINT('Ctrl Pts',(-42.4939953305734,45.3921528864746,-8.38483035099147));
#36338=CARTESIAN_POINT('Ctrl Pts',(-42.4948439764137,45.3874775165642,-8.37747363926369));
#36339=CARTESIAN_POINT('Ctrl Pts',(-42.495975311871,45.3812447496024,-8.367666357555));
#36340=CARTESIAN_POINT('Ctrl Pts',(-42.4969273136303,45.3750282608174,-8.35778516090225));
#36341=CARTESIAN_POINT('Ctrl Pts',(-42.4976922377975,45.3688434603943,-8.34785239611548));
#36342=CARTESIAN_POINT('Ctrl Pts',(-42.499222086132,45.356473859548,-8.32798686654192));
#36343=CARTESIAN_POINT('Ctrl Pts',(-42.4999999944414,45.3442749544122,-8.30798620935071));
#36344=CARTESIAN_POINT('Ctrl Pts',(-42.5,45.3322472608192,-8.28784904304297));
#36345=CARTESIAN_POINT('',(-42.5,44.9368005344369,-5.30952630282035));
#36346=CARTESIAN_POINT('Origin',(-42.5,48.5946168001447,-6.3392739254555));
#36347=CARTESIAN_POINT('',(-42.,44.9368005344369,-5.30952630282035));
#36348=CARTESIAN_POINT('',(-45.,51.536059602328,-8.74508236369084));
#36349=CARTESIAN_POINT('',(-45.,51.536059602328,-8.74508236369084));
#36350=CARTESIAN_POINT('',(-45.,51.508884771774,-8.77792974158369));
#36351=CARTESIAN_POINT('Origin',(-45.,48.5946168001447,-6.3392739254555));
#36352=CARTESIAN_POINT('',(-39.,51.508884771774,-8.77792974158369));
#36353=CARTESIAN_POINT('Origin',(-33.6035533905933,20.7255401693197,-1.65106132841495));
#36354=CARTESIAN_POINT('',(-38.5,21.2255401693197,3.24538528099178));
#36355=CARTESIAN_POINT('',(-33.6035533905933,21.2255401693197,-1.65106132841495));
#36356=CARTESIAN_POINT('',(-38.1464466094067,20.7255401693197,3.59893867158506));
#36357=CARTESIAN_POINT('Origin',(-38.5,20.7255401693197,3.24538528099178));
#36358=CARTESIAN_POINT('',(-38.5,20.2255401693197,3.24538528099178));
#36359=CARTESIAN_POINT('Origin',(-38.5,20.7255401693197,3.24538528099178));
#36360=CARTESIAN_POINT('',(-33.6035533905933,20.2255401693197,-1.65106132841495));
#36361=CARTESIAN_POINT('Origin',(-56.6690017314647,51.2606171391062,-5.48344555910069));
#36362=CARTESIAN_POINT('',(-45.,52.2127601173067,-5.17779257111684));
#36363=CARTESIAN_POINT('Origin',(-45.,51.2606171391062,-5.48344555910069));
#36364=CARTESIAN_POINT('',(-46.,52.2127601173067,-5.17779257111684));
#36365=CARTESIAN_POINT('Origin',(-46.,51.2606171391062,-5.48344555910069));
#36366=CARTESIAN_POINT('',(-39.,52.2127601173067,-5.17779257111684));
#36367=CARTESIAN_POINT('Origin',(-45.5,34.999999994595,6.54998265276524E-10));
#36368=CARTESIAN_POINT('',(-46.,18.5003030276807,-0.0999999993449978));
#36369=CARTESIAN_POINT('',(-46.,51.1450373092966,-3.40408138892615));
#36370=CARTESIAN_POINT('Origin',(-46.,34.999999994595,6.54998265276524E-10));
#36371=CARTESIAN_POINT('',(-45.9555887800306,18.2967958718846,-0.306006949495285));
#36372=CARTESIAN_POINT('Ctrl Pts',(-46.,18.5003030276807,-0.0999999993450115));
#36373=CARTESIAN_POINT('Ctrl Pts',(-46.,18.4992558329104,-0.101053560099588));
#36374=CARTESIAN_POINT('Ctrl Pts',(-45.9999966700292,18.4982086857198,-0.102107173286065));
#36375=CARTESIAN_POINT('Ctrl Pts',(-45.9996635810359,18.4458478552488,-0.15479633935181));
#36376=CARTESIAN_POINT('Ctrl Pts',(-45.9913355526387,18.3943785329297,-0.206835262360072));
#36377=CARTESIAN_POINT('Ctrl Pts',(-45.9691910264621,18.3285791615519,-0.273658918954145));
#36378=CARTESIAN_POINT('Ctrl Pts',(-45.9628568381822,18.3125775652319,-0.289933483313417));
#36379=CARTESIAN_POINT('Ctrl Pts',(-45.9555887800306,18.2967958718846,-0.306006949495283));
#36380=CARTESIAN_POINT('Ctrl Pts',(-45.9555887800306,18.2967958718846,-0.306006949495305));
#36381=CARTESIAN_POINT('Ctrl Pts',(-45.9449932969391,18.2729210477128,-0.282057797773911));
#36382=CARTESIAN_POINT('Ctrl Pts',(-45.9326039209885,18.2499149945026,-0.256551740908599));
#36383=CARTESIAN_POINT('Ctrl Pts',(-45.8727877520938,18.1568360367878,-0.141654083468818));
#36384=CARTESIAN_POINT('Ctrl Pts',(-45.8108354668021,18.0994281624082,-0.0403766288579828));
#36385=CARTESIAN_POINT('Ctrl Pts',(-45.66422179789,18.0209250472194,0.185216864286121));
#36386=CARTESIAN_POINT('Ctrl Pts',(-45.5833719890191,18.0028239046249,0.303488964622345));
#36387=CARTESIAN_POINT('Ctrl Pts',(-45.5021062448037,18.005240100147,0.421930518868415));
#36388=CARTESIAN_POINT('Ctrl Pts',(-45.5010531216555,18.0052749455469,0.423465305044224));
#36389=CARTESIAN_POINT('Ctrl Pts',(-45.5,18.0053133249326,0.425000000654998));
#36390=CARTESIAN_POINT('Origin',(-45.5,51.1450373092966,-3.40408138892615));
#36391=CARTESIAN_POINT('Origin',(-38.5,20.7255401693197,-2.54750793782168));
#36392=CARTESIAN_POINT('',(-39.,22.3838525644974,-5.04750793782168));
#36393=CARTESIAN_POINT('Ctrl Pts',(-39.,22.3838525644974,-5.04750793782167));
#36394=CARTESIAN_POINT('Ctrl Pts',(-39.,21.8319612940798,-5.04750793782167));
#36395=CARTESIAN_POINT('Ctrl Pts',(-38.7253086676699,21.2293456661496,-5.04750793782167));
#36396=CARTESIAN_POINT('Ctrl Pts',(-38.5,20.7255401693197,-5.04750793782167));
#36397=CARTESIAN_POINT('',(-39.,21.7255401693197,0.280919186924516));
#36398=CARTESIAN_POINT('Origin',(-39.,20.7255401693197,-2.54750793782168));
#36399=CARTESIAN_POINT('Ctrl Pts',(-38.5,21.2255401693197,-0.0980181950384987));
#36400=CARTESIAN_POINT('Ctrl Pts',(-38.5068454246389,21.2255401693197,-0.0980181950384987));
#36401=CARTESIAN_POINT('Ctrl Pts',(-38.5137049378611,21.2256807402194,-0.0979034111946656));
#36402=CARTESIAN_POINT('Ctrl Pts',(-38.574487053383,21.2281840126506,-0.0958597862843718));
#36403=CARTESIAN_POINT('Ctrl Pts',(-38.6266179130002,21.2390520815176,-0.0869664209613689));
#36404=CARTESIAN_POINT('Ctrl Pts',(-38.7343668418878,21.2793907655706,-0.0543730508899923));
#36405=CARTESIAN_POINT('Ctrl Pts',(-38.78643803375,21.3115857796177,-0.0285603789798281));
#36406=CARTESIAN_POINT('Ctrl Pts',(-38.8850764070747,21.3983579125978,0.0395179277113517));
#36407=CARTESIAN_POINT('Ctrl Pts',(-38.9288507671717,21.4581607205219,0.0855519592452586));
#36408=CARTESIAN_POINT('Ctrl Pts',(-38.9855092027928,21.5879815055175,0.182314659292807));
#36409=CARTESIAN_POINT('Ctrl Pts',(-38.9995659056513,21.6549720437981,0.23098157372654));
#36410=CARTESIAN_POINT('Ctrl Pts',(-38.9999967004912,21.7234428444743,0.279435862662996));
#36411=CARTESIAN_POINT('Ctrl Pts',(-39.,21.7244914385065,0.280177622254829));
#36412=CARTESIAN_POINT('Ctrl Pts',(-39.,21.7255401693197,0.280919186924513));
#36413=CARTESIAN_POINT('Origin',(-29.,39.9592920728172,13.6255430020507));
#36414=CARTESIAN_POINT('',(-38.5,42.4320695804642,13.2576144795422));
#36415=CARTESIAN_POINT('',(-38.5,42.3431727827618,14.3786118971418));
#36416=CARTESIAN_POINT('Origin',(-38.5,39.9592920728172,13.6255430020507));
#36417=CARTESIAN_POINT('',(-39.0000007124813,41.5278577838399,15.5722329253343));
#36418=CARTESIAN_POINT('Ctrl Pts',(-38.5,42.3431727827618,14.3786118971418));
#36419=CARTESIAN_POINT('Ctrl Pts',(-38.5000000077005,42.3332086900109,14.4101537768502));
#36420=CARTESIAN_POINT('Ctrl Pts',(-38.5011441382107,42.3226977455079,14.4412538314269));
#36421=CARTESIAN_POINT('Ctrl Pts',(-38.5032795388733,42.3116545294946,14.4719455803148));
#36422=CARTESIAN_POINT('Ctrl Pts',(-38.5053650307195,42.3008694167266,14.5019199983108));
#36423=CARTESIAN_POINT('Ctrl Pts',(-38.508397245918,42.2895766285646,14.5315047214286));
#36424=CARTESIAN_POINT('Ctrl Pts',(-38.5122659121586,42.2777903788033,14.560725126099));
#36425=CARTESIAN_POINT('Ctrl Pts',(-38.5123584949005,42.2775083169113,14.5614244123686));
#36426=CARTESIAN_POINT('Ctrl Pts',(-38.5124515587901,42.2772259722098,14.5621234898174));
#36427=CARTESIAN_POINT('Ctrl Pts',(-38.5125451029203,42.2769433448068,14.5628223586732));
#36428=CARTESIAN_POINT('Ctrl Pts',(-38.5204047012563,42.2531969284258,14.6215414731906));
#36429=CARTESIAN_POINT('Ctrl Pts',(-38.5316230864511,42.2274542851575,14.678791826982));
#36430=CARTESIAN_POINT('Ctrl Pts',(-38.5455756576484,42.1997725506805,14.7347081062229));
#36431=CARTESIAN_POINT('Ctrl Pts',(-38.5458333631473,42.1992612660511,14.7357408859475));
#36432=CARTESIAN_POINT('Ctrl Pts',(-38.5460920078943,42.1987493186971,14.7367732092197));
#36433=CARTESIAN_POINT('Ctrl Pts',(-38.5463515890497,42.198236708752,14.7378050766535));
#36434=CARTESIAN_POINT('Ctrl Pts',(-38.5532264361405,42.1846605499451,14.7651334503657));
#36435=CARTESIAN_POINT('Ctrl Pts',(-38.5607577577241,42.1706197463063,14.7921419417493));
#36436=CARTESIAN_POINT('Ctrl Pts',(-38.5688931749403,42.1561170515871,14.8188409584105));
#36437=CARTESIAN_POINT('Ctrl Pts',(-38.5692268877671,42.1555221545926,14.8199361455517));
#36438=CARTESIAN_POINT('Ctrl Pts',(-38.5695616183357,42.1549264801115,14.8210308116731));
#36439=CARTESIAN_POINT('Ctrl Pts',(-38.5698973635473,42.154330028203,14.8221249573718));
#36440=CARTESIAN_POINT('Ctrl Pts',(-38.5738150194497,42.14737030619,14.8348920385001));
#36441=CARTESIAN_POINT('Ctrl Pts',(-38.577870714569,42.1403046598116,14.8475883947252));
#36442=CARTESIAN_POINT('Ctrl Pts',(-38.5820595331401,42.1331334156534,14.8602145438691));
#36443=CARTESIAN_POINT('Ctrl Pts',(-38.5824259517601,42.1325061081337,14.8613190214363));
#36444=CARTESIAN_POINT('Ctrl Pts',(-38.5827934015943,42.131877974359,14.8624229867996));
#36445=CARTESIAN_POINT('Ctrl Pts',(-38.583161865111,42.1312490379265,14.8635264020773));
#36446=CARTESIAN_POINT('Ctrl Pts',(-38.5854521945635,42.1273396369413,14.8703851123555));
#36447=CARTESIAN_POINT('Ctrl Pts',(-38.5877835411621,42.1233961168598,14.8772279257529));
#36448=CARTESIAN_POINT('Ctrl Pts',(-38.5901473083312,42.1194314671435,14.8840331025438));
#36449=CARTESIAN_POINT('Ctrl Pts',(-38.5921285576339,42.1161083989546,14.889737028018));
#36450=CARTESIAN_POINT('Ctrl Pts',(-38.5941334747018,42.1127691873607,14.8954168261815));
#36451=CARTESIAN_POINT('Ctrl Pts',(-38.5961604876585,42.109415270011,14.9010704368357));
#36452=CARTESIAN_POINT('Ctrl Pts',(-38.5965518410689,42.1087677324663,14.9021619739191));
#36453=CARTESIAN_POINT('Ctrl Pts',(-38.5969440505148,42.1081195824686,14.9032526548805));
#36454=CARTESIAN_POINT('Ctrl Pts',(-38.5973371193626,42.1074708069969,14.9043425046045));
#36455=CARTESIAN_POINT('Ctrl Pts',(-38.616455858449,42.0759145820762,14.9573524356527));
#36456=CARTESIAN_POINT('Ctrl Pts',(-38.637546796424,42.0429898336134,15.0082122863806));
#36457=CARTESIAN_POINT('Ctrl Pts',(-38.6602044929259,42.0087701554417,15.0571992418101));
#36458=CARTESIAN_POINT('Ctrl Pts',(-38.6605754259393,42.0082099392546,15.0580012156115));
#36459=CARTESIAN_POINT('Ctrl Pts',(-38.660946780572,42.0076493755921,15.05880268647));
#36460=CARTESIAN_POINT('Ctrl Pts',(-38.6613185556365,42.0070884646104,15.0596036552468));
#36461=CARTESIAN_POINT('Ctrl Pts',(-38.6842707148083,41.9724596813525,15.1090528104149));
#36462=CARTESIAN_POINT('Ctrl Pts',(-38.7088227250363,41.9365078483921,15.1565891613654));
#36463=CARTESIAN_POINT('Ctrl Pts',(-38.7346967461674,41.8992750612305,15.2023961989802));
#36464=CARTESIAN_POINT('Ctrl Pts',(-38.7348418833976,41.8990662083594,15.2026531480849));
#36465=CARTESIAN_POINT('Ctrl Pts',(-38.7349870623364,41.8988573151551,15.2029100427124));
#36466=CARTESIAN_POINT('Ctrl Pts',(-38.7351322829497,41.8986483816199,15.2031668828852));
#36467=CARTESIAN_POINT('Ctrl Pts',(-38.7611663896273,41.8611922807128,15.2492113410937));
#36468=CARTESIAN_POINT('Ctrl Pts',(-38.7885386651593,41.8224405096622,15.2935061409713));
#36469=CARTESIAN_POINT('Ctrl Pts',(-38.8170528293073,41.7824089839123,15.336170002502));
#36470=CARTESIAN_POINT('Ctrl Pts',(-38.8173470127179,41.7819959747595,15.3366101697196));
#36471=CARTESIAN_POINT('Ctrl Pts',(-38.8176413177686,41.7815828293836,15.3370501632323));
#36472=CARTESIAN_POINT('Ctrl Pts',(-38.8179357442455,41.7811695478035,15.3374899831624));
#36473=CARTESIAN_POINT('Ctrl Pts',(-38.8319101796259,41.7615538637952,15.3583652633232));
#36474=CARTESIAN_POINT('Ctrl Pts',(-38.8461591058041,41.7416309802697,15.3788488599945));
#36475=CARTESIAN_POINT('Ctrl Pts',(-38.8606646627554,41.721400690848,15.3989502376356));
#36476=CARTESIAN_POINT('Ctrl Pts',(-38.8612582506509,41.7205728388073,15.399772814424));
#36477=CARTESIAN_POINT('Ctrl Pts',(-38.8618522681823,41.7197444719415,15.4005947511531));
#36478=CARTESIAN_POINT('Ctrl Pts',(-38.8624467141622,41.7189155902482,15.4014160484433));
#36479=CARTESIAN_POINT('Ctrl Pts',(-38.8692685604167,41.7094033659809,15.4108412343021));
#36480=CARTESIAN_POINT('Ctrl Pts',(-38.8761468721562,41.6998233208851,15.4201821773756));
#36481=CARTESIAN_POINT('Ctrl Pts',(-38.8830800584607,41.6901753398805,15.4294396502778));
#36482=CARTESIAN_POINT('Ctrl Pts',(-38.8838431424214,41.6891134587721,15.4304585510802));
#36483=CARTESIAN_POINT('Ctrl Pts',(-38.8846068740394,41.6880507781269,15.4314764182716));
#36484=CARTESIAN_POINT('Ctrl Pts',(-38.8853712624626,41.6869872820628,15.4324932680928));
#36485=CARTESIAN_POINT('Ctrl Pts',(-38.892157093119,41.6775461341138,15.4415203157032));
#36486=CARTESIAN_POINT('Ctrl Pts',(-38.8989982959301,41.6680357161533,15.450471659057));
#36487=CARTESIAN_POINT('Ctrl Pts',(-38.9058773734152,41.6584782132661,15.4593277211414));
#36488=CARTESIAN_POINT('Ctrl Pts',(-38.906818535116,41.6571706025156,15.4605393641955));
#36489=CARTESIAN_POINT('Ctrl Pts',(-38.9077604254252,41.6558620830411,15.4617492470449));
#36490=CARTESIAN_POINT('Ctrl Pts',(-38.9087029786515,41.6545527406419,15.4629572906983));
#36491=CARTESIAN_POINT('Ctrl Pts',(-38.9384215702937,41.6132693298003,15.5010467640772));
#36492=CARTESIAN_POINT('Ctrl Pts',(-38.9688951268995,41.5710315059527,15.537445734224));
#36493=CARTESIAN_POINT('Ctrl Pts',(-39.0000000000001,41.5278577956883,15.5722329400385));
#36494=CARTESIAN_POINT('Ctrl Pts',(-39.,40.8143424311349,15.9747745540142));
#36495=CARTESIAN_POINT('Ctrl Pts',(-38.9999968905168,40.8170927138004,15.9737735329881));
#36496=CARTESIAN_POINT('Ctrl Pts',(-38.9999946894569,40.8198412391743,15.9727676820533));
#36497=CARTESIAN_POINT('Ctrl Pts',(-38.9999897502085,40.8289450514986,15.9694179091687));
#36498=CARTESIAN_POINT('Ctrl Pts',(-38.9999901119293,40.8352925259715,15.9670530039168));
#36499=CARTESIAN_POINT('Ctrl Pts',(-38.9999942307407,40.8506913969669,15.9612444021708));
#36500=CARTESIAN_POINT('Ctrl Pts',(-38.9999993739327,40.8597325759833,15.9577738411329));
#36501=CARTESIAN_POINT('Ctrl Pts',(-39.0000003297456,40.8747622467481,15.9519041034816));
#36502=CARTESIAN_POINT('Ctrl Pts',(-39.0000000885938,40.8807723014066,15.9495301114465));
#36503=CARTESIAN_POINT('Ctrl Pts',(-39.0000001965139,40.8947797407981,15.9439340336549));
#36504=CARTESIAN_POINT('Ctrl Pts',(-39.0000001605784,40.9027598121034,15.940698024332));
#36505=CARTESIAN_POINT('Ctrl Pts',(-38.9999998192051,40.942521297217,15.9243345703678));
#36506=CARTESIAN_POINT('Ctrl Pts',(-39.0000017835329,40.97404626887,15.9105936160279));
#36507=CARTESIAN_POINT('Ctrl Pts',(-38.9999985969878,41.0673343728555,15.8676202695839));
#36508=CARTESIAN_POINT('Ctrl Pts',(-39.0000128649755,41.1281933283618,15.836501644433));
#36509=CARTESIAN_POINT('Ctrl Pts',(-38.9999896085028,41.3072289986956,15.7354956717247));
#36510=CARTESIAN_POINT('Ctrl Pts',(-39.0000027484886,41.420993774444,15.6583397034461));
#36511=CARTESIAN_POINT('Ctrl Pts',(-39.0000021374439,41.5278577779207,15.5722329179781));
#36512=CARTESIAN_POINT('',(-39.0000009660842,40.0090091820249,16.1250482632156));
#36513=CARTESIAN_POINT('Ctrl Pts',(-39.0000021374439,40.009009188616,16.1250485948423));
#36514=CARTESIAN_POINT('Ctrl Pts',(-39.0000027484886,40.1462201394576,16.1223193620086));
#36515=CARTESIAN_POINT('Ctrl Pts',(-38.9999896085026,40.2829639141646,16.1082976744922));
#36516=CARTESIAN_POINT('Ctrl Pts',(-39.000012709303,40.4836859506285,16.070843227177));
#36517=CARTESIAN_POINT('Ctrl Pts',(-38.999998495505,40.5489785071788,16.0559240454488));
#36518=CARTESIAN_POINT('Ctrl Pts',(-39.00000168396,40.6474424173353,16.0292233275237));
#36519=CARTESIAN_POINT('Ctrl Pts',(-38.9999997950044,40.6810944759589,16.0193331550335));
#36520=CARTESIAN_POINT('Ctrl Pts',(-39.0000001459518,40.7229000764915,16.0060849487778));
#36521=CARTESIAN_POINT('Ctrl Pts',(-39.0000001992107,40.7312588065207,16.0033875103362));
#36522=CARTESIAN_POINT('Ctrl Pts',(-39.0000001046533,40.7458809046931,15.9985835987506));
#36523=CARTESIAN_POINT('Ctrl Pts',(-39.0000001267302,40.7521343550355,15.9965015278252));
#36524=CARTESIAN_POINT('Ctrl Pts',(-38.9999997949692,40.7677237236382,15.9912428672298));
#36525=CARTESIAN_POINT('Ctrl Pts',(-38.999994537334,40.7770652735991,15.9880299495346));
#36526=CARTESIAN_POINT('Ctrl Pts',(-38.9999906714831,40.7910293624736,15.9831344162146));
#36527=CARTESIAN_POINT('Ctrl Pts',(-38.9999900510404,40.7956664120109,15.9814933750465));
#36528=CARTESIAN_POINT('Ctrl Pts',(-38.9999915437067,40.8026152317053,15.9790111028118));
#36529=CARTESIAN_POINT('Ctrl Pts',(-38.999992445271,40.8049306360383,15.9781801334451));
#36530=CARTESIAN_POINT('Ctrl Pts',(-38.9999945939801,40.8084239880366,15.9769205901392));
#36531=CARTESIAN_POINT('Ctrl Pts',(-38.9999954547499,40.8096028407755,15.9764945475109));
#36532=CARTESIAN_POINT('Ctrl Pts',(-38.9999972820434,40.8117313539399,15.9757234829694));
#36533=CARTESIAN_POINT('Ctrl Pts',(-38.9999981957157,40.8126811315419,15.9753787697989));
#36534=CARTESIAN_POINT('Ctrl Pts',(-38.9999994703163,40.8138679676572,15.9749472039047));
#36535=CARTESIAN_POINT('Ctrl Pts',(-38.9999997317273,40.8141052060082,15.9748608968992));
#36536=CARTESIAN_POINT('Ctrl Pts',(-39.,40.8143424311286,15.9747745540165));
#36537=CARTESIAN_POINT('',(-38.5,38.6171968569105,15.7347562277442));
#36538=CARTESIAN_POINT('Ctrl Pts',(-39.0000000000001,40.0090091891848,16.1250486231625));
#36539=CARTESIAN_POINT('Ctrl Pts',(-38.9688951268995,39.9535754234747,16.1261516034788));
#36540=CARTESIAN_POINT('Ctrl Pts',(-38.9384215702936,39.8978225662111,16.1254183244919));
#36541=CARTESIAN_POINT('Ctrl Pts',(-38.9087029786515,39.8417141971955,16.1227765600433));
#36542=CARTESIAN_POINT('Ctrl Pts',(-38.900871177093,39.8269278433471,16.1220803704265));
#36543=CARTESIAN_POINT('Ctrl Pts',(-38.8930854972452,39.812104173315,16.121250562334));
#36544=CARTESIAN_POINT('Ctrl Pts',(-38.8853712624626,39.7972860007029,16.1202882861625));
#36545=CARTESIAN_POINT('Ctrl Pts',(-38.8776618357207,39.7824770637934,16.1193266097476));
#36546=CARTESIAN_POINT('Ctrl Pts',(-38.8700193900109,39.7676654292003,16.1182323509774));
#36547=CARTESIAN_POINT('Ctrl Pts',(-38.8624467141621,39.7528514459051,16.1170048756422));
#36548=CARTESIAN_POINT('Ctrl Pts',(-38.8473257421527,39.7232711718738,16.1145538767407));
#36549=CARTESIAN_POINT('Ctrl Pts',(-38.8324820332758,39.6936801258928,16.1115718386542));
#36550=CARTESIAN_POINT('Ctrl Pts',(-38.8179357442455,39.6640712649591,16.1080507411338));
#36551=CARTESIAN_POINT('Ctrl Pts',(-38.789103594054,39.6053836420433,16.1010715856711));
#36552=CARTESIAN_POINT('Ctrl Pts',(-38.7614349860432,39.546627259783,16.0919785071308));
#36553=CARTESIAN_POINT('Ctrl Pts',(-38.7351322829496,39.4877360325772,16.0806672153616));
#36554=CARTESIAN_POINT('Ctrl Pts',(-38.7090981762719,39.4294461873854,16.0694714315848));
#36555=CARTESIAN_POINT('Ctrl Pts',(-38.6843994622029,39.3710250338492,16.0561042678525));
#36556=CARTESIAN_POINT('Ctrl Pts',(-38.6613185556365,39.3123854456582,16.0403953443325));
#36557=CARTESIAN_POINT('Ctrl Pts',(-38.6382376490702,39.2537458574673,16.0246864208126));
#36558=CARTESIAN_POINT('Ctrl Pts',(-38.6167688528615,39.1948893427871,16.0066396660535));
#36559=CARTESIAN_POINT('Ctrl Pts',(-38.5973369701107,39.1356882476495,15.9859829569921));
#36560=CARTESIAN_POINT('Ctrl Pts',(-38.5949079847669,39.1282881107573,15.9834008683595));
#36561=CARTESIAN_POINT('Ctrl Pts',(-38.5925110755004,39.1208825181482,15.980777828273));
#36562=CARTESIAN_POINT('Ctrl Pts',(-38.5901473083312,39.1134711369412,15.9781131881224));
#36563=CARTESIAN_POINT('Ctrl Pts',(-38.5877835411621,39.1060597557343,15.9754485479717));
#36564=CARTESIAN_POINT('Ctrl Pts',(-38.5854521945635,39.0986403684223,15.9727414946403));
#36565=CARTESIAN_POINT('Ctrl Pts',(-38.583161865111,39.0912368995364,15.9700003322593));
#36566=CARTESIAN_POINT('Ctrl Pts',(-38.578581206206,39.0764299617645,15.9645180074973));
#36567=CARTESIAN_POINT('Ctrl Pts',(-38.5741577180041,39.0616657176126,15.9588918794025));
#36568=CARTESIAN_POINT('Ctrl Pts',(-38.5698973635473,39.0469434995135,15.9531211601745));
#36569=CARTESIAN_POINT('Ctrl Pts',(-38.5613766546335,39.0174990633154,15.9415797217185));
#36570=CARTESIAN_POINT('Ctrl Pts',(-38.5535084406888,38.9882227073311,15.9294599923279));
#36571=CARTESIAN_POINT('Ctrl Pts',(-38.5463515890497,38.9591092562873,15.9167510543452));
#36572=CARTESIAN_POINT('Ctrl Pts',(-38.5320378857717,38.9008823541996,15.8913331783798));
#36573=CARTESIAN_POINT('Ctrl Pts',(-38.5205498688876,38.8433076021544,15.8635646015542));
#36574=CARTESIAN_POINT('Ctrl Pts',(-38.5125451029203,38.7863397520739,15.8332981660507));
#36575=CARTESIAN_POINT('Ctrl Pts',(-38.5085427199367,38.7578558270336,15.8181649482989));
#36576=CARTESIAN_POINT('Ctrl Pts',(-38.5054149395359,38.7295228449587,15.8024072356763));
#36577=CARTESIAN_POINT('Ctrl Pts',(-38.5032795388733,38.7013349747927,15.7859944344156));
#36578=CARTESIAN_POINT('Ctrl Pts',(-38.5011441382107,38.6731471046267,15.7695816331548));
#36579=CARTESIAN_POINT('Ctrl Pts',(-38.5000000077005,38.6451045242559,15.7525139140583));
#36580=CARTESIAN_POINT('Ctrl Pts',(-38.5,38.6171968569105,15.7347562277442));
#36581=CARTESIAN_POINT('',(-38.5,37.8285347084959,14.9331641453451));
#36582=CARTESIAN_POINT('Origin',(-38.5,39.9592920728172,13.6255430020507));
#36583=CARTESIAN_POINT('',(-35.0170134743162,37.8285347084959,14.9331641453451));
#36584=CARTESIAN_POINT('',(-29.,37.8285347084959,14.9331641453451));
#36585=CARTESIAN_POINT('',(-34.,37.6100605208524,14.4805933603648));
#36586=CARTESIAN_POINT('Ctrl Pts',(-35.0170134743162,37.8285347084959,14.9331641453451));
#36587=CARTESIAN_POINT('Ctrl Pts',(-34.7766127063766,37.8285347084959,14.9331641453451));
#36588=CARTESIAN_POINT('Ctrl Pts',(-34.4906799668777,37.8067211571775,14.9017335941734));
#36589=CARTESIAN_POINT('Ctrl Pts',(-34.1966444375895,37.7349198556759,14.7674315769327));
#36590=CARTESIAN_POINT('Ctrl Pts',(-34.1089154055285,37.7055249860502,14.710036118503));
#36591=CARTESIAN_POINT('Ctrl Pts',(-34.0408467644713,37.6652672213039,14.619544442247));
#36592=CARTESIAN_POINT('Ctrl Pts',(-34.0255956953052,37.6540485473767,14.5934125444763));
#36593=CARTESIAN_POINT('Ctrl Pts',(-34.0051635787926,37.6314787713743,14.537775795392));
#36594=CARTESIAN_POINT('Ctrl Pts',(-34.,37.6201314456043,14.5082629987137));
#36595=CARTESIAN_POINT('Ctrl Pts',(-34.,37.6100605208524,14.4805933603648));
#36596=CARTESIAN_POINT('',(-34.,40.8143424311314,15.9747745540155));
#36597=CARTESIAN_POINT('Origin',(-34.,39.9592920728172,13.6255430020507));
#36598=CARTESIAN_POINT('',(-30.,40.8143424311314,15.9747745540155));
#36599=CARTESIAN_POINT('',(-29.,40.8143424311314,15.9747745540155));
#36600=CARTESIAN_POINT('',(-30.,39.104241714503,11.2763114500859));
#36601=CARTESIAN_POINT('Origin',(-30.,39.9592920728172,13.6255430020507));
#36602=CARTESIAN_POINT('',(-34.,39.104241714503,11.2763114500859));
#36603=CARTESIAN_POINT('',(-29.,39.104241714503,11.2763114500859));
#36604=CARTESIAN_POINT('',(-34.,37.4865145651702,13.9934715245592));
#36605=CARTESIAN_POINT('Origin',(-34.,39.9592920728172,13.6255430020507));
#36606=CARTESIAN_POINT('',(-38.5,37.4865145651702,13.9934715245592));
#36607=CARTESIAN_POINT('',(-29.,37.4865145651702,13.9934715245592));
#36608=CARTESIAN_POINT('',(-38.5,42.0900494371385,12.3179218587563));
#36609=CARTESIAN_POINT('Origin',(-38.5,39.9592920728172,13.6255430020507));
#36610=CARTESIAN_POINT('',(-35.0170134743163,42.0900494371385,12.3179218587563));
#36611=CARTESIAN_POINT('',(-29.,42.0900494371385,12.3179218587563));
#36612=CARTESIAN_POINT('',(-35.0170134743163,42.4320695804642,13.2576144795422));
#36613=CARTESIAN_POINT('Ctrl Pts',(-35.0170134743162,42.0900494371384,12.3179218587562));
#36614=CARTESIAN_POINT('Ctrl Pts',(-34.8763912574935,42.0900494371384,12.3179218587562));
#36615=CARTESIAN_POINT('Ctrl Pts',(-34.7227068456195,42.0966450458144,12.3283241056387));
#36616=CARTESIAN_POINT('Ctrl Pts',(-34.4287581602092,42.129619262702,12.3842797507388));
#36617=CARTESIAN_POINT('Ctrl Pts',(-34.2881480947843,42.1555402154976,12.4282739810068));
#36618=CARTESIAN_POINT('Ctrl Pts',(-34.1203544496629,42.2110688218831,12.5387497630338));
#36619=CARTESIAN_POINT('Ctrl Pts',(-34.0637027306899,42.2362087483756,12.5914709241387));
#36620=CARTESIAN_POINT('Ctrl Pts',(-34.0133005472596,42.2750367777858,12.6827660115511));
#36621=CARTESIAN_POINT('Ctrl Pts',(-34.,42.2936559145693,12.7296439456481));
#36622=CARTESIAN_POINT('Ctrl Pts',(-34.,42.3233913349946,12.8113413418248));
#36623=CARTESIAN_POINT('Ctrl Pts',(-34.0133005472596,42.3392608039313,12.8592200731723));
#36624=CARTESIAN_POINT('Ctrl Pts',(-34.0637027306899,42.3682001587783,12.954114343782));
#36625=CARTESIAN_POINT('Ctrl Pts',(-34.1203544496629,42.3828303669148,13.010660729539));
#36626=CARTESIAN_POINT('Ctrl Pts',(-34.2881480947843,42.4113054504164,13.1309831886277));
#36627=CARTESIAN_POINT('Ctrl Pts',(-34.4287581602092,42.419727794681,13.1813463915421));
#36628=CARTESIAN_POINT('Ctrl Pts',(-34.7227068456195,42.4304356744304,13.2454063205866));
#36629=CARTESIAN_POINT('Ctrl Pts',(-34.8763912574935,42.4320695804641,13.2576144795422));
#36630=CARTESIAN_POINT('Ctrl Pts',(-35.0170134743163,42.4320695804641,13.2576144795422));
#36631=CARTESIAN_POINT('',(-29.,42.4320695804641,13.2576144795422));
#36632=CARTESIAN_POINT('Origin',(-39.22360679775,44.2375118611403,12.0683983434524));
#36633=CARTESIAN_POINT('',(-38.5,43.7265178053794,11.7222960833984));
#36634=CARTESIAN_POINT('',(-34.22360679775,41.7172702375127,12.4536023913736));
#36635=CARTESIAN_POINT('',(-38.5441280858669,43.7468303076589,11.7137963479747));
#36636=CARTESIAN_POINT('Ctrl Pts',(-38.5440016100281,43.7469422033269,11.7139571265323));
#36637=CARTESIAN_POINT('Ctrl Pts',(-38.5292760478545,43.7401182142464,11.7166614290024));
#36638=CARTESIAN_POINT('Ctrl Pts',(-38.5146380311988,43.733428008513,11.7197809751451));
#36639=CARTESIAN_POINT('Ctrl Pts',(-38.5,43.7265178053794,11.7222960833984));
#36640=CARTESIAN_POINT('',(-38.72360679775,44.5278928504519,11.9627083067462));
#36641=CARTESIAN_POINT('Ctrl Pts',(-38.72360679775,44.5278928504519,11.9627083067462));
#36642=CARTESIAN_POINT('Ctrl Pts',(-38.7236071164119,44.5278766506594,11.9626610048945));
#36643=CARTESIAN_POINT('Ctrl Pts',(-38.7236377977353,44.5263169066445,11.9581067008717));
#36644=CARTESIAN_POINT('Ctrl Pts',(-38.7234503028571,44.520850205933,11.9447315525215));
#36645=CARTESIAN_POINT('Ctrl Pts',(-38.723342992434,44.5184918291995,11.9391932030999));
#36646=CARTESIAN_POINT('Ctrl Pts',(-38.7230280284375,44.5139105406859,11.9293688690194));
#36647=CARTESIAN_POINT('Ctrl Pts',(-38.7228315133244,44.5113575460494,11.9240782791388));
#36648=CARTESIAN_POINT('Ctrl Pts',(-38.7225554022308,44.5083537654735,11.9182473393015));
#36649=CARTESIAN_POINT('Ctrl Pts',(-38.7223509758947,44.5062438964329,11.9142436273831));
#36650=CARTESIAN_POINT('Ctrl Pts',(-38.7221757851806,44.5045443141253,11.9111107329527));
#36651=CARTESIAN_POINT('Ctrl Pts',(-38.7211370061962,44.4947708585985,11.893369944279));
#36652=CARTESIAN_POINT('Ctrl Pts',(-38.7197824514153,44.4839246948589,11.8766973126298));
#36653=CARTESIAN_POINT('Ctrl Pts',(-38.7166904074296,44.4614933674347,11.8468572654181));
#36654=CARTESIAN_POINT('Ctrl Pts',(-38.7136115309805,44.4428720028296,11.8254832543129));
#36655=CARTESIAN_POINT('Ctrl Pts',(-38.70872340737,44.4182229539639,11.802559675333));
#36656=CARTESIAN_POINT('Ctrl Pts',(-38.7059584939507,44.4051961946696,11.7916315968734));
#36657=CARTESIAN_POINT('Ctrl Pts',(-38.7047052738609,44.3994663885684,11.7870654782422));
#36658=CARTESIAN_POINT('Ctrl Pts',(-38.7038547062334,44.3956143340404,11.7840477294714));
#36659=CARTESIAN_POINT('Ctrl Pts',(-38.7032214091466,44.3927808200249,11.7818771590184));
#36660=CARTESIAN_POINT('Ctrl Pts',(-38.6991435597199,44.3746484434328,11.768149243923));
#36661=CARTESIAN_POINT('Ctrl Pts',(-38.6939534751656,44.3509398269105,11.7516647130115));
#36662=CARTESIAN_POINT('Ctrl Pts',(-38.6825469826753,44.3014072596727,11.7259746102914));
#36663=CARTESIAN_POINT('Ctrl Pts',(-38.6781356817267,44.2825555777659,11.7172813976112));
#36664=CARTESIAN_POINT('Ctrl Pts',(-38.6703956763465,44.2502811390231,11.7048893824249));
#36665=CARTESIAN_POINT('Ctrl Pts',(-38.6676285755574,44.2388574863255,11.700869024046));
#36666=CARTESIAN_POINT('Ctrl Pts',(-38.6631728052587,44.220673155864,11.6951324489139));
#36667=CARTESIAN_POINT('Ctrl Pts',(-38.6608686350217,44.2113188406999,11.692337984379));
#36668=CARTESIAN_POINT('Ctrl Pts',(-38.6584459125517,44.2015637758563,11.689680377803));
#36669=CARTESIAN_POINT('Ctrl Pts',(-38.6568040371926,44.1949707280962,11.6879419285137));
#36670=CARTESIAN_POINT('Ctrl Pts',(-38.6557035360131,44.1905661326844,11.6868273823973));
#36671=CARTESIAN_POINT('Ctrl Pts',(-38.6178946480498,44.0395516274507,11.6496180167347));
#36672=CARTESIAN_POINT('Ctrl Pts',(-38.5753923705026,43.8784299792084,11.6667202780775));
#36673=CARTESIAN_POINT('Ctrl Pts',(-38.5440337731008,43.7469571082004,11.713951220573));
#36674=CARTESIAN_POINT('',(-38.7126236016579,44.5498673281012,12.1194208390779));
#36675=CARTESIAN_POINT('Origin',(-38.4999999999771,43.897527876974,12.1921423938054));
#36676=CARTESIAN_POINT('',(-38.5,44.068537948705,12.6619887041843));
#36677=CARTESIAN_POINT('Origin',(-38.4999999999998,43.8975278770413,12.1921423937908));
#36678=CARTESIAN_POINT('',(-40.02360679775,44.7843989811175,12.4014365965151));
#36679=CARTESIAN_POINT('Origin',(-38.5,39.9592920728172,13.6255430020507));
#36680=CARTESIAN_POINT('',(-39.,42.9591643136975,13.5978565722447));
#36681=CARTESIAN_POINT('Ctrl Pts',(-39.,42.9591643136975,13.5978565722447));
#36682=CARTESIAN_POINT('Ctrl Pts',(-39.,42.9581087837868,13.5971247176931));
#36683=CARTESIAN_POINT('Ctrl Pts',(-38.9999967004912,42.957053117491,13.596393058341));
#36684=CARTESIAN_POINT('Ctrl Pts',(-38.9995659056514,42.8881025866701,13.5486238950522));
#36685=CARTESIAN_POINT('Ctrl Pts',(-38.9855092027928,42.8194585327967,13.5023184456178));
#36686=CARTESIAN_POINT('Ctrl Pts',(-38.9288507671717,42.6841300141038,13.4134216044716));
#36687=CARTESIAN_POINT('Ctrl Pts',(-38.8850764070747,42.6204184094289,13.3729699132262));
#36688=CARTESIAN_POINT('Ctrl Pts',(-38.78643803375,42.5267679096371,13.3147149323868));
#36689=CARTESIAN_POINT('Ctrl Pts',(-38.7343668418878,42.4915005890015,13.2932899690069));
#36690=CARTESIAN_POINT('Ctrl Pts',(-38.6266179130002,42.4470761971575,13.2665315943734));
#36691=CARTESIAN_POINT('Ctrl Pts',(-38.574487053383,42.435002068918,13.2593606603393));
#36692=CARTESIAN_POINT('Ctrl Pts',(-38.5137049378611,42.4322255200745,13.2577073145927));
#36693=CARTESIAN_POINT('Ctrl Pts',(-38.5068454246389,42.4320695804641,13.2576144795422));
#36694=CARTESIAN_POINT('Ctrl Pts',(-38.5,42.4320695804641,13.2576144795422));
#36695=CARTESIAN_POINT('',(-39.,42.8199489247508,14.5292256761601));
#36696=CARTESIAN_POINT('Origin',(-39.,39.9592920728172,13.6255430020507));
#36697=CARTESIAN_POINT('Origin',(-38.5,42.8199489247508,14.5292256761601));
#36698=CARTESIAN_POINT('Origin',(-45.5,34.999999994595,6.55E-10));
#36699=CARTESIAN_POINT('',(-46.,37.3980464303344,4.94968416149168));
#36700=CARTESIAN_POINT('',(-46.,40.0130956859299,-2.2624923395573));
#36701=CARTESIAN_POINT('Origin',(-46.,34.999999994595,6.55E-10));
#36702=CARTESIAN_POINT('',(-45.5,38.0494565603535,5.1672831023974));
#36703=CARTESIAN_POINT('Ctrl Pts',(-46.,37.3980464303344,4.94968416149168));
#36704=CARTESIAN_POINT('Ctrl Pts',(-46.,37.3994318538483,4.95017943538276));
#36705=CARTESIAN_POINT('Ctrl Pts',(-45.9999966939211,37.4008173501861,4.95067451566463));
#36706=CARTESIAN_POINT('Ctrl Pts',(-45.9996751413526,37.4681689180479,4.97473062725169));
#36707=CARTESIAN_POINT('Ctrl Pts',(-45.9918589780635,37.5346003819143,4.99794942213878));
#36708=CARTESIAN_POINT('Ctrl Pts',(-45.9609910872761,37.660320616289,5.04101720165774));
#36709=CARTESIAN_POINT('Ctrl Pts',(-45.9385897729845,37.7203693432866,5.06117119476266));
#36710=CARTESIAN_POINT('Ctrl Pts',(-45.8753161788561,37.8365974383146,5.09953476308977));
#36711=CARTESIAN_POINT('Ctrl Pts',(-45.8328892935188,37.8925460613842,5.1176110195544));
#36712=CARTESIAN_POINT('Ctrl Pts',(-45.7398209612911,37.9740390280872,5.14361816527401));
#36713=CARTESIAN_POINT('Ctrl Pts',(-45.6935221969332,38.0032214033414,5.15280579280595));
#36714=CARTESIAN_POINT('Ctrl Pts',(-45.5969081567834,38.0402032793475,5.16440403484684));
#36715=CARTESIAN_POINT('Ctrl Pts',(-45.548970157778,38.0494565603535,5.16728310239741));
#36716=CARTESIAN_POINT('Ctrl Pts',(-45.5,38.0494565603535,5.1672831023974));
#36717=CARTESIAN_POINT('',(-45.5,40.65404535889,-2.00792704445741));
#36718=CARTESIAN_POINT('Origin',(-45.5,34.999999994595,6.55E-10));
#36719=CARTESIAN_POINT('Ctrl Pts',(-45.5,40.6540453588901,-2.00792704445741));
#36720=CARTESIAN_POINT('Ctrl Pts',(-45.548789362425,40.6540453588901,-2.00792704445741));
#36721=CARTESIAN_POINT('Ctrl Pts',(-45.5965455901767,40.6451475101065,-2.01167834637272));
#36722=CARTESIAN_POINT('Ctrl Pts',(-45.6928616793168,40.6095174739276,-2.02660507937416));
#36723=CARTESIAN_POINT('Ctrl Pts',(-45.7390416503862,40.5813587441991,-2.03836511974797));
#36724=CARTESIAN_POINT('Ctrl Pts',(-45.8320302750286,40.5024145653791,-2.07097275523011));
#36725=CARTESIAN_POINT('Ctrl Pts',(-45.8744779446781,40.4479929468233,-2.0932224681912));
#36726=CARTESIAN_POINT('Ctrl Pts',(-45.938073114642,40.3340359761707,-2.13897191074204));
#36727=CARTESIAN_POINT('Ctrl Pts',(-45.9606603025493,40.274676254965,-2.16245456892374));
#36728=CARTESIAN_POINT('Ctrl Pts',(-45.9917939389948,40.149785821394,-2.21095308019115));
#36729=CARTESIAN_POINT('Ctrl Pts',(-45.9996738586592,40.0834454567978,-2.23623621749007));
#36730=CARTESIAN_POINT('Ctrl Pts',(-45.9999966944273,40.0158649969536,-2.261459414675));
#36731=CARTESIAN_POINT('Ctrl Pts',(-46.,40.0144803764284,-2.2619759759402));
#36732=CARTESIAN_POINT('Ctrl Pts',(-46.,40.0130956859299,-2.2624923395573));
#36733=CARTESIAN_POINT('Origin',(-45.5,34.999999994595,6.55E-10));
#36734=CARTESIAN_POINT('',(-45.5,39.9429588225849,9.26375507215795));
#36735=CARTESIAN_POINT('',(-45.5,44.7486243140984,-3.90055430318255));
#36736=CARTESIAN_POINT('Origin',(-45.5,34.999999994595,6.55E-10));
#36737=CARTESIAN_POINT('',(-46.,39.7058929474701,9.94256362962317));
#36738=CARTESIAN_POINT('Ctrl Pts',(-46.,39.7058929474701,9.94256362962317));
#36739=CARTESIAN_POINT('Ctrl Pts',(-46.,39.7064029596768,9.94115718202826));
#36740=CARTESIAN_POINT('Ctrl Pts',(-45.9999966732101,39.7069128712589,9.93975069394934));
#36741=CARTESIAN_POINT('Ctrl Pts',(-45.9994167224429,39.7513586367457,9.81712829100708));
#36742=CARTESIAN_POINT('Ctrl Pts',(-45.9741804024558,39.793704872613,9.69777801260392));
#36743=CARTESIAN_POINT('Ctrl Pts',(-45.8908401903906,39.8587623022576,9.51130839381713));
#36744=CARTESIAN_POINT('Ctrl Pts',(-45.8419265836025,39.8831029548383,9.44038249890876));
#36745=CARTESIAN_POINT('Ctrl Pts',(-45.7416688429776,39.9154223669426,9.34548629444458));
#36746=CARTESIAN_POINT('Ctrl Pts',(-45.692683116429,39.9266743500376,9.31215790076818));
#36747=CARTESIAN_POINT('Ctrl Pts',(-45.5938300790286,39.9398264006189,9.27310033615707));
#36748=CARTESIAN_POINT('Ctrl Pts',(-45.5475202328385,39.9429588225849,9.26375507215796));
#36749=CARTESIAN_POINT('Ctrl Pts',(-45.5,39.9429588225849,9.26375507215796));
#36750=CARTESIAN_POINT('',(-46.,45.0056642132324,-4.57019513127084));
#36751=CARTESIAN_POINT('Origin',(-46.,34.999999994595,6.55E-10));
#36752=CARTESIAN_POINT('Ctrl Pts',(-45.5,44.7486243140985,-3.90055430318256));
#36753=CARTESIAN_POINT('Ctrl Pts',(-45.547591906806,44.7486243140985,-3.90055430318256));
#36754=CARTESIAN_POINT('Ctrl Pts',(-45.5939774616156,44.7522730358909,-3.90971545551159));
#36755=CARTESIAN_POINT('Ctrl Pts',(-45.6929687045191,44.7674781615144,-3.94804694909195));
#36756=CARTESIAN_POINT('Ctrl Pts',(-45.7420177519214,44.7804280920619,-3.98076791095232));
#36757=CARTESIAN_POINT('Ctrl Pts',(-45.8422980854956,44.8170645841968,-4.07406216072172));
#36758=CARTESIAN_POINT('Ctrl Pts',(-45.8911666603025,44.8442733910796,-4.14382603215572));
#36759=CARTESIAN_POINT('Ctrl Pts',(-45.974280185293,44.9148993422513,-4.32766254923343));
#36760=CARTESIAN_POINT('Ctrl Pts',(-45.999417856672,44.9595063347814,-4.44561304986796));
#36761=CARTESIAN_POINT('Ctrl Pts',(-45.9999966731511,45.0046273583855,-4.56739570686552));
#36762=CARTESIAN_POINT('Ctrl Pts',(-46.,45.0051458369342,-4.56879540212099));
#36763=CARTESIAN_POINT('Ctrl Pts',(-46.,45.0056642132324,-4.57019513127083));
#36764=CARTESIAN_POINT('Ctrl Pts',(-36.918924746634,26.,0.));
#36765=CARTESIAN_POINT('Ctrl Pts',(-36.7522580799673,26.,5.19615242270663));
#36766=CARTESIAN_POINT('Ctrl Pts',(-36.5855914133007,30.5,7.79422863405995));
#36767=CARTESIAN_POINT('Ctrl Pts',(-36.418924746634,35.,10.3923048454133));
#36768=CARTESIAN_POINT('Ctrl Pts',(-36.2522580799673,39.5,7.79422863405995));
#36769=CARTESIAN_POINT('Ctrl Pts',(-36.0855914133007,44.,5.19615242270663));
#36770=CARTESIAN_POINT('Ctrl Pts',(-35.918924746634,44.,1.10218211923262E-15));
#36771=CARTESIAN_POINT('Ctrl Pts',(-35.7522580799673,44.,-5.19615242270663));
#36772=CARTESIAN_POINT('Ctrl Pts',(-35.5855914133007,39.5,-7.79422863405995));
#36773=CARTESIAN_POINT('Ctrl Pts',(-35.418924746634,35.,-10.3923048454133));
#36774=CARTESIAN_POINT('Ctrl Pts',(-35.2522580799673,30.5,-7.79422863405995));
#36775=CARTESIAN_POINT('Ctrl Pts',(-35.0855914133007,26.,-5.19615242270663));
#36776=CARTESIAN_POINT('Ctrl Pts',(-34.918924746634,26.,0.));
#36777=CARTESIAN_POINT('Ctrl Pts',(-34.7522580799673,26.,5.19615242270663));
#36778=CARTESIAN_POINT('Ctrl Pts',(-34.5855914133007,30.5,7.79422863405995));
#36779=CARTESIAN_POINT('Ctrl Pts',(-34.418924746634,35.,10.3923048454133));
#36780=CARTESIAN_POINT('Ctrl Pts',(-34.2522580799673,39.5,7.79422863405995));
#36781=CARTESIAN_POINT('Ctrl Pts',(-34.0855914133007,44.,5.19615242270663));
#36782=CARTESIAN_POINT('Ctrl Pts',(-33.918924746634,44.,1.10218211923262E-15));
#36783=CARTESIAN_POINT('Ctrl Pts',(-33.7522580799673,44.,-5.19615242270663));
#36784=CARTESIAN_POINT('Ctrl Pts',(-33.5855914133007,39.5,-7.79422863405995));
#36785=CARTESIAN_POINT('Ctrl Pts',(-33.418924746634,35.,-10.3923048454133));
#36786=CARTESIAN_POINT('Ctrl Pts',(-33.2522580799673,30.5,-7.79422863405995));
#36787=CARTESIAN_POINT('Ctrl Pts',(-33.0855914133007,26.,-5.19615242270663));
#36788=CARTESIAN_POINT('Ctrl Pts',(-32.918924746634,26.,0.));
#36789=CARTESIAN_POINT('Ctrl Pts',(-32.7522580799673,26.,5.19615242270663));
#36790=CARTESIAN_POINT('Ctrl Pts',(-32.5855914133007,30.5,7.79422863405995));
#36791=CARTESIAN_POINT('Ctrl Pts',(-32.418924746634,35.,10.3923048454133));
#36792=CARTESIAN_POINT('Ctrl Pts',(-32.2522580799673,39.5,7.79422863405995));
#36793=CARTESIAN_POINT('Ctrl Pts',(-32.0855914133007,44.,5.19615242270663));
#36794=CARTESIAN_POINT('Ctrl Pts',(-31.918924746634,44.,1.10218211923262E-15));
#36795=CARTESIAN_POINT('Ctrl Pts',(-31.7522580799673,44.,-5.19615242270663));
#36796=CARTESIAN_POINT('Ctrl Pts',(-31.5855914133007,39.5,-7.79422863405995));
#36797=CARTESIAN_POINT('Ctrl Pts',(-31.418924746634,35.,-10.3923048454133));
#36798=CARTESIAN_POINT('Ctrl Pts',(-31.2522580799673,30.5,-7.79422863405995));
#36799=CARTESIAN_POINT('Ctrl Pts',(-31.0855914133007,26.,-5.19615242270663));
#36800=CARTESIAN_POINT('Ctrl Pts',(-30.918924746634,26.,0.));
#36801=CARTESIAN_POINT('Ctrl Pts',(-30.7522580799673,26.,5.19615242270663));
#36802=CARTESIAN_POINT('Ctrl Pts',(-30.5855914133007,30.5,7.79422863405995));
#36803=CARTESIAN_POINT('Ctrl Pts',(-30.418924746634,35.,10.3923048454133));
#36804=CARTESIAN_POINT('Ctrl Pts',(-30.2522580799673,39.5,7.79422863405995));
#36805=CARTESIAN_POINT('Ctrl Pts',(-30.0855914133007,44.,5.19615242270663));
#36806=CARTESIAN_POINT('Ctrl Pts',(-29.918924746634,44.,1.10218211923262E-15));
#36807=CARTESIAN_POINT('Ctrl Pts',(-29.7522580799673,44.,-5.19615242270663));
#36808=CARTESIAN_POINT('Ctrl Pts',(-29.5855914133007,39.5,-7.79422863405995));
#36809=CARTESIAN_POINT('Ctrl Pts',(-29.418924746634,35.,-10.3923048454133));
#36810=CARTESIAN_POINT('Ctrl Pts',(-29.2522580799673,30.5,-7.79422863405995));
#36811=CARTESIAN_POINT('Ctrl Pts',(-29.0855914133007,26.,-5.19615242270663));
#36812=CARTESIAN_POINT('Ctrl Pts',(-28.918924746634,26.,0.));
#36813=CARTESIAN_POINT('Ctrl Pts',(-28.7522580799673,26.,5.19615242270663));
#36814=CARTESIAN_POINT('Ctrl Pts',(-28.5855914133007,30.5,7.79422863405995));
#36815=CARTESIAN_POINT('Ctrl Pts',(-28.418924746634,35.,10.3923048454133));
#36816=CARTESIAN_POINT('Ctrl Pts',(-28.2522580799673,39.5,7.79422863405995));
#36817=CARTESIAN_POINT('Ctrl Pts',(-28.0855914133007,44.,5.19615242270663));
#36818=CARTESIAN_POINT('Ctrl Pts',(-27.918924746634,44.,1.10218211923262E-15));
#36819=CARTESIAN_POINT('Ctrl Pts',(-27.7522580799673,44.,-5.19615242270663));
#36820=CARTESIAN_POINT('Ctrl Pts',(-27.5855914133007,39.5,-7.79422863405995));
#36821=CARTESIAN_POINT('Ctrl Pts',(-27.418924746634,35.,-10.3923048454133));
#36822=CARTESIAN_POINT('Ctrl Pts',(-27.2522580799673,30.5,-7.79422863405995));
#36823=CARTESIAN_POINT('Ctrl Pts',(-27.0855914133007,26.,-5.19615242270663));
#36824=CARTESIAN_POINT('Ctrl Pts',(-26.918924746634,26.,0.));
#36825=CARTESIAN_POINT('Ctrl Pts',(-26.7522580799673,26.,5.19615242270663));
#36826=CARTESIAN_POINT('Ctrl Pts',(-26.5855914133007,30.5,7.79422863405995));
#36827=CARTESIAN_POINT('Ctrl Pts',(-26.418924746634,35.,10.3923048454133));
#36828=CARTESIAN_POINT('Ctrl Pts',(-26.2522580799673,39.5,7.79422863405995));
#36829=CARTESIAN_POINT('Ctrl Pts',(-26.0855914133007,44.,5.19615242270663));
#36830=CARTESIAN_POINT('Ctrl Pts',(-25.918924746634,44.,1.10218211923262E-15));
#36831=CARTESIAN_POINT('Ctrl Pts',(-25.7522580799673,44.,-5.19615242270663));
#36832=CARTESIAN_POINT('Ctrl Pts',(-25.5855914133007,39.5,-7.79422863405995));
#36833=CARTESIAN_POINT('Ctrl Pts',(-25.418924746634,35.,-10.3923048454133));
#36834=CARTESIAN_POINT('Ctrl Pts',(-25.2522580799673,30.5,-7.79422863405995));
#36835=CARTESIAN_POINT('Ctrl Pts',(-25.0855914133007,26.,-5.19615242270663));
#36836=CARTESIAN_POINT('Ctrl Pts',(-24.918924746634,26.,0.));
#36837=CARTESIAN_POINT('Ctrl Pts',(-24.7522580799673,26.,5.19615242270663));
#36838=CARTESIAN_POINT('Ctrl Pts',(-24.5855914133007,30.5,7.79422863405995));
#36839=CARTESIAN_POINT('Ctrl Pts',(-24.418924746634,35.,10.3923048454133));
#36840=CARTESIAN_POINT('Ctrl Pts',(-24.2522580799673,39.5,7.79422863405995));
#36841=CARTESIAN_POINT('Ctrl Pts',(-24.0855914133007,44.,5.19615242270663));
#36842=CARTESIAN_POINT('Ctrl Pts',(-23.918924746634,44.,1.10218211923262E-15));
#36843=CARTESIAN_POINT('Ctrl Pts',(-23.7522580799673,44.,-5.19615242270663));
#36844=CARTESIAN_POINT('Ctrl Pts',(-23.5855914133007,39.5,-7.79422863405995));
#36845=CARTESIAN_POINT('Ctrl Pts',(-23.418924746634,35.,-10.3923048454133));
#36846=CARTESIAN_POINT('Ctrl Pts',(-23.2522580799673,30.5,-7.79422863405995));
#36847=CARTESIAN_POINT('Ctrl Pts',(-23.0855914133007,26.,-5.19615242270663));
#36848=CARTESIAN_POINT('Ctrl Pts',(-22.918924746634,26.,0.));
#36849=CARTESIAN_POINT('Ctrl Pts',(-22.7522580799673,26.,5.19615242270663));
#36850=CARTESIAN_POINT('Ctrl Pts',(-22.5855914133007,30.5,7.79422863405995));
#36851=CARTESIAN_POINT('Ctrl Pts',(-22.418924746634,35.,10.3923048454133));
#36852=CARTESIAN_POINT('Ctrl Pts',(-22.2522580799674,39.5,7.79422863405995));
#36853=CARTESIAN_POINT('Ctrl Pts',(-22.0855914133007,44.,5.19615242270663));
#36854=CARTESIAN_POINT('Ctrl Pts',(-21.918924746634,44.,1.10218211923262E-15));
#36855=CARTESIAN_POINT('Ctrl Pts',(-21.7522580799673,44.,-5.19615242270663));
#36856=CARTESIAN_POINT('Ctrl Pts',(-21.5855914133006,39.5,-7.79422863405995));
#36857=CARTESIAN_POINT('Ctrl Pts',(-21.418924746634,35.,-10.3923048454133));
#36858=CARTESIAN_POINT('Ctrl Pts',(-21.2522580799673,30.5,-7.79422863405995));
#36859=CARTESIAN_POINT('Ctrl Pts',(-21.0855914133007,26.,-5.19615242270663));
#36860=CARTESIAN_POINT('Ctrl Pts',(-20.918924746634,26.,0.));
#36861=CARTESIAN_POINT('Ctrl Pts',(-20.7522580799673,26.,5.19615242270663));
#36862=CARTESIAN_POINT('Ctrl Pts',(-20.5855914133006,30.5,7.79422863405995));
#36863=CARTESIAN_POINT('Ctrl Pts',(-20.418924746634,35.,10.3923048454133));
#36864=CARTESIAN_POINT('Ctrl Pts',(-20.2522580799673,39.5,7.79422863405995));
#36865=CARTESIAN_POINT('Ctrl Pts',(-20.0855914133007,44.,5.19615242270663));
#36866=CARTESIAN_POINT('Ctrl Pts',(-19.918924746634,44.,1.10218211923262E-15));
#36867=CARTESIAN_POINT('Ctrl Pts',(-19.7522580799674,44.,-5.19615242270663));
#36868=CARTESIAN_POINT('Ctrl Pts',(-19.5855914133006,39.5,-7.79422863405995));
#36869=CARTESIAN_POINT('Ctrl Pts',(-19.418924746634,35.,-10.3923048454133));
#36870=CARTESIAN_POINT('Ctrl Pts',(-19.2522580799674,30.5,-7.79422863405995));
#36871=CARTESIAN_POINT('Ctrl Pts',(-19.0855914133007,26.,-5.19615242270663));
#36872=CARTESIAN_POINT('Ctrl Pts',(-18.918924746634,26.,0.));
#36873=CARTESIAN_POINT('Ctrl Pts',(-18.7522580799673,26.,5.19615242270663));
#36874=CARTESIAN_POINT('Ctrl Pts',(-18.5855914133006,30.5,7.79422863405995));
#36875=CARTESIAN_POINT('Ctrl Pts',(-18.418924746634,35.,10.3923048454133));
#36876=CARTESIAN_POINT('Ctrl Pts',(-18.2522580799673,39.5,7.79422863405995));
#36877=CARTESIAN_POINT('Ctrl Pts',(-18.0855914133006,44.,5.19615242270663));
#36878=CARTESIAN_POINT('Ctrl Pts',(-17.918924746634,44.,1.10218211923262E-15));
#36879=CARTESIAN_POINT('Ctrl Pts',(-17.7522580799673,44.,-5.19615242270663));
#36880=CARTESIAN_POINT('Ctrl Pts',(-17.5855914133006,39.5,-7.79422863405995));
#36881=CARTESIAN_POINT('Ctrl Pts',(-17.418924746634,35.,-10.3923048454133));
#36882=CARTESIAN_POINT('Ctrl Pts',(-17.2522580799673,30.5,-7.79422863405995));
#36883=CARTESIAN_POINT('Ctrl Pts',(-17.0855914133007,26.,-5.19615242270663));
#36884=CARTESIAN_POINT('Ctrl Pts',(-16.918924746634,26.,0.));
#36885=CARTESIAN_POINT('Ctrl Pts',(-36.918924746634,24.4,0.));
#36886=CARTESIAN_POINT('Ctrl Pts',(-36.7522580799673,24.4,6.11991285341003));
#36887=CARTESIAN_POINT('Ctrl Pts',(-36.5855914133007,29.7,9.17986928011504));
#36888=CARTESIAN_POINT('Ctrl Pts',(-36.418924746634,35.,12.2398257068201));
#36889=CARTESIAN_POINT('Ctrl Pts',(-36.2522580799673,40.3,9.17986928011504));
#36890=CARTESIAN_POINT('Ctrl Pts',(-36.0855914133007,45.6,6.11991285341004));
#36891=CARTESIAN_POINT('Ctrl Pts',(-35.918924746634,45.6,1.29812560709619E-15));
#36892=CARTESIAN_POINT('Ctrl Pts',(-35.7522580799673,45.6,-6.11991285341003));
#36893=CARTESIAN_POINT('Ctrl Pts',(-35.5855914133007,40.3,-9.17986928011504));
#36894=CARTESIAN_POINT('Ctrl Pts',(-35.418924746634,35.,-12.2398257068201));
#36895=CARTESIAN_POINT('Ctrl Pts',(-35.2522580799673,29.7,-9.17986928011506));
#36896=CARTESIAN_POINT('Ctrl Pts',(-35.0855914133007,24.4,-6.11991285341004));
#36897=CARTESIAN_POINT('Ctrl Pts',(-34.918924746634,24.4,0.));
#36898=CARTESIAN_POINT('Ctrl Pts',(-34.7522580799673,24.4,6.11991285341003));
#36899=CARTESIAN_POINT('Ctrl Pts',(-34.5855914133007,29.7,9.17986928011504));
#36900=CARTESIAN_POINT('Ctrl Pts',(-34.418924746634,35.,12.2398257068201));
#36901=CARTESIAN_POINT('Ctrl Pts',(-34.2522580799673,40.3,9.17986928011504));
#36902=CARTESIAN_POINT('Ctrl Pts',(-34.0855914133007,45.6,6.11991285341004));
#36903=CARTESIAN_POINT('Ctrl Pts',(-33.918924746634,45.6,1.29812560709619E-15));
#36904=CARTESIAN_POINT('Ctrl Pts',(-33.7522580799673,45.6,-6.11991285341003));
#36905=CARTESIAN_POINT('Ctrl Pts',(-33.5855914133007,40.3,-9.17986928011504));
#36906=CARTESIAN_POINT('Ctrl Pts',(-33.418924746634,35.,-12.2398257068201));
#36907=CARTESIAN_POINT('Ctrl Pts',(-33.2522580799673,29.7,-9.17986928011506));
#36908=CARTESIAN_POINT('Ctrl Pts',(-33.0855914133007,24.4,-6.11991285341004));
#36909=CARTESIAN_POINT('Ctrl Pts',(-32.918924746634,24.4,0.));
#36910=CARTESIAN_POINT('Ctrl Pts',(-32.7522580799673,24.4,6.11991285341003));
#36911=CARTESIAN_POINT('Ctrl Pts',(-32.5855914133007,29.7,9.17986928011504));
#36912=CARTESIAN_POINT('Ctrl Pts',(-32.418924746634,35.,12.2398257068201));
#36913=CARTESIAN_POINT('Ctrl Pts',(-32.2522580799673,40.3,9.17986928011504));
#36914=CARTESIAN_POINT('Ctrl Pts',(-32.0855914133007,45.6,6.11991285341004));
#36915=CARTESIAN_POINT('Ctrl Pts',(-31.918924746634,45.6,1.29812560709619E-15));
#36916=CARTESIAN_POINT('Ctrl Pts',(-31.7522580799673,45.6,-6.11991285341003));
#36917=CARTESIAN_POINT('Ctrl Pts',(-31.5855914133007,40.3,-9.17986928011504));
#36918=CARTESIAN_POINT('Ctrl Pts',(-31.418924746634,35.,-12.2398257068201));
#36919=CARTESIAN_POINT('Ctrl Pts',(-31.2522580799673,29.7,-9.17986928011506));
#36920=CARTESIAN_POINT('Ctrl Pts',(-31.0855914133007,24.4,-6.11991285341004));
#36921=CARTESIAN_POINT('Ctrl Pts',(-30.918924746634,24.4,0.));
#36922=CARTESIAN_POINT('Ctrl Pts',(-30.7522580799673,24.4,6.11991285341003));
#36923=CARTESIAN_POINT('Ctrl Pts',(-30.5855914133007,29.7,9.17986928011504));
#36924=CARTESIAN_POINT('Ctrl Pts',(-30.418924746634,35.,12.2398257068201));
#36925=CARTESIAN_POINT('Ctrl Pts',(-30.2522580799673,40.3,9.17986928011504));
#36926=CARTESIAN_POINT('Ctrl Pts',(-30.0855914133007,45.6,6.11991285341004));
#36927=CARTESIAN_POINT('Ctrl Pts',(-29.918924746634,45.6,1.29812560709619E-15));
#36928=CARTESIAN_POINT('Ctrl Pts',(-29.7522580799673,45.6,-6.11991285341003));
#36929=CARTESIAN_POINT('Ctrl Pts',(-29.5855914133007,40.3,-9.17986928011504));
#36930=CARTESIAN_POINT('Ctrl Pts',(-29.418924746634,35.,-12.2398257068201));
#36931=CARTESIAN_POINT('Ctrl Pts',(-29.2522580799673,29.7,-9.17986928011506));
#36932=CARTESIAN_POINT('Ctrl Pts',(-29.0855914133007,24.4,-6.11991285341004));
#36933=CARTESIAN_POINT('Ctrl Pts',(-28.918924746634,24.4,0.));
#36934=CARTESIAN_POINT('Ctrl Pts',(-28.7522580799673,24.4,6.11991285341003));
#36935=CARTESIAN_POINT('Ctrl Pts',(-28.5855914133007,29.7,9.17986928011504));
#36936=CARTESIAN_POINT('Ctrl Pts',(-28.418924746634,35.,12.2398257068201));
#36937=CARTESIAN_POINT('Ctrl Pts',(-28.2522580799673,40.3,9.17986928011504));
#36938=CARTESIAN_POINT('Ctrl Pts',(-28.0855914133007,45.6,6.11991285341004));
#36939=CARTESIAN_POINT('Ctrl Pts',(-27.918924746634,45.6,1.29812560709619E-15));
#36940=CARTESIAN_POINT('Ctrl Pts',(-27.7522580799673,45.6,-6.11991285341003));
#36941=CARTESIAN_POINT('Ctrl Pts',(-27.5855914133007,40.3,-9.17986928011504));
#36942=CARTESIAN_POINT('Ctrl Pts',(-27.418924746634,35.,-12.2398257068201));
#36943=CARTESIAN_POINT('Ctrl Pts',(-27.2522580799673,29.7,-9.17986928011506));
#36944=CARTESIAN_POINT('Ctrl Pts',(-27.0855914133007,24.4,-6.11991285341004));
#36945=CARTESIAN_POINT('Ctrl Pts',(-26.918924746634,24.4,0.));
#36946=CARTESIAN_POINT('Ctrl Pts',(-26.7522580799673,24.4,6.11991285341003));
#36947=CARTESIAN_POINT('Ctrl Pts',(-26.5855914133007,29.7,9.17986928011504));
#36948=CARTESIAN_POINT('Ctrl Pts',(-26.418924746634,35.,12.2398257068201));
#36949=CARTESIAN_POINT('Ctrl Pts',(-26.2522580799673,40.3,9.17986928011504));
#36950=CARTESIAN_POINT('Ctrl Pts',(-26.0855914133007,45.6,6.11991285341004));
#36951=CARTESIAN_POINT('Ctrl Pts',(-25.918924746634,45.6,1.29812560709619E-15));
#36952=CARTESIAN_POINT('Ctrl Pts',(-25.7522580799673,45.6,-6.11991285341003));
#36953=CARTESIAN_POINT('Ctrl Pts',(-25.5855914133007,40.3,-9.17986928011504));
#36954=CARTESIAN_POINT('Ctrl Pts',(-25.418924746634,35.,-12.2398257068201));
#36955=CARTESIAN_POINT('Ctrl Pts',(-25.2522580799673,29.7,-9.17986928011506));
#36956=CARTESIAN_POINT('Ctrl Pts',(-25.0855914133007,24.4,-6.11991285341004));
#36957=CARTESIAN_POINT('Ctrl Pts',(-24.918924746634,24.4,0.));
#36958=CARTESIAN_POINT('Ctrl Pts',(-24.7522580799673,24.4,6.11991285341003));
#36959=CARTESIAN_POINT('Ctrl Pts',(-24.5855914133007,29.7,9.17986928011504));
#36960=CARTESIAN_POINT('Ctrl Pts',(-24.418924746634,35.,12.2398257068201));
#36961=CARTESIAN_POINT('Ctrl Pts',(-24.2522580799673,40.3,9.17986928011504));
#36962=CARTESIAN_POINT('Ctrl Pts',(-24.0855914133007,45.6,6.11991285341004));
#36963=CARTESIAN_POINT('Ctrl Pts',(-23.918924746634,45.6,1.29812560709619E-15));
#36964=CARTESIAN_POINT('Ctrl Pts',(-23.7522580799673,45.6,-6.11991285341003));
#36965=CARTESIAN_POINT('Ctrl Pts',(-23.5855914133007,40.3,-9.17986928011504));
#36966=CARTESIAN_POINT('Ctrl Pts',(-23.418924746634,35.,-12.2398257068201));
#36967=CARTESIAN_POINT('Ctrl Pts',(-23.2522580799673,29.7,-9.17986928011506));
#36968=CARTESIAN_POINT('Ctrl Pts',(-23.0855914133007,24.4,-6.11991285341004));
#36969=CARTESIAN_POINT('Ctrl Pts',(-22.918924746634,24.4,0.));
#36970=CARTESIAN_POINT('Ctrl Pts',(-22.7522580799673,24.4,6.11991285341003));
#36971=CARTESIAN_POINT('Ctrl Pts',(-22.5855914133007,29.7,9.17986928011504));
#36972=CARTESIAN_POINT('Ctrl Pts',(-22.418924746634,35.,12.2398257068201));
#36973=CARTESIAN_POINT('Ctrl Pts',(-22.2522580799673,40.3,9.17986928011504));
#36974=CARTESIAN_POINT('Ctrl Pts',(-22.0855914133007,45.6,6.11991285341004));
#36975=CARTESIAN_POINT('Ctrl Pts',(-21.918924746634,45.6,1.29812560709619E-15));
#36976=CARTESIAN_POINT('Ctrl Pts',(-21.7522580799673,45.6,-6.11991285341003));
#36977=CARTESIAN_POINT('Ctrl Pts',(-21.5855914133007,40.3,-9.17986928011504));
#36978=CARTESIAN_POINT('Ctrl Pts',(-21.418924746634,35.,-12.2398257068201));
#36979=CARTESIAN_POINT('Ctrl Pts',(-21.2522580799673,29.7,-9.17986928011506));
#36980=CARTESIAN_POINT('Ctrl Pts',(-21.0855914133007,24.4,-6.11991285341004));
#36981=CARTESIAN_POINT('Ctrl Pts',(-20.918924746634,24.4,0.));
#36982=CARTESIAN_POINT('Ctrl Pts',(-20.7522580799673,24.4,6.11991285341003));
#36983=CARTESIAN_POINT('Ctrl Pts',(-20.5855914133007,29.7,9.17986928011504));
#36984=CARTESIAN_POINT('Ctrl Pts',(-20.418924746634,35.,12.2398257068201));
#36985=CARTESIAN_POINT('Ctrl Pts',(-20.2522580799673,40.3,9.17986928011504));
#36986=CARTESIAN_POINT('Ctrl Pts',(-20.0855914133007,45.6,6.11991285341004));
#36987=CARTESIAN_POINT('Ctrl Pts',(-19.918924746634,45.6,1.29812560709619E-15));
#36988=CARTESIAN_POINT('Ctrl Pts',(-19.7522580799673,45.6,-6.11991285341003));
#36989=CARTESIAN_POINT('Ctrl Pts',(-19.5855914133007,40.3,-9.17986928011504));
#36990=CARTESIAN_POINT('Ctrl Pts',(-19.418924746634,35.,-12.2398257068201));
#36991=CARTESIAN_POINT('Ctrl Pts',(-19.2522580799673,29.7,-9.17986928011506));
#36992=CARTESIAN_POINT('Ctrl Pts',(-19.0855914133006,24.4,-6.11991285341004));
#36993=CARTESIAN_POINT('Ctrl Pts',(-18.918924746634,24.4,0.));
#36994=CARTESIAN_POINT('Ctrl Pts',(-18.7522580799673,24.4,6.11991285341003));
#36995=CARTESIAN_POINT('Ctrl Pts',(-18.5855914133007,29.7,9.17986928011504));
#36996=CARTESIAN_POINT('Ctrl Pts',(-18.418924746634,35.,12.2398257068201));
#36997=CARTESIAN_POINT('Ctrl Pts',(-18.2522580799673,40.3,9.17986928011504));
#36998=CARTESIAN_POINT('Ctrl Pts',(-18.0855914133007,45.6,6.11991285341004));
#36999=CARTESIAN_POINT('Ctrl Pts',(-17.918924746634,45.6,1.29812560709619E-15));
#37000=CARTESIAN_POINT('Ctrl Pts',(-17.7522580799674,45.6,-6.11991285341003));
#37001=CARTESIAN_POINT('Ctrl Pts',(-17.5855914133007,40.3,-9.17986928011504));
#37002=CARTESIAN_POINT('Ctrl Pts',(-17.418924746634,35.,-12.2398257068201));
#37003=CARTESIAN_POINT('Ctrl Pts',(-17.2522580799674,29.7,-9.17986928011506));
#37004=CARTESIAN_POINT('Ctrl Pts',(-17.0855914133007,24.4,-6.11991285341004));
#37005=CARTESIAN_POINT('Ctrl Pts',(-16.918924746634,24.4,0.));
#37006=CARTESIAN_POINT('Ctrl Pts',(-38.518924746634,24.4,0.));
#37007=CARTESIAN_POINT('Ctrl Pts',(-38.3522580799673,24.4,6.11991285341003));
#37008=CARTESIAN_POINT('Ctrl Pts',(-38.1855914133007,29.7,9.17986928011504));
#37009=CARTESIAN_POINT('Ctrl Pts',(-38.018924746634,35.,12.2398257068201));
#37010=CARTESIAN_POINT('Ctrl Pts',(-37.8522580799673,40.3,9.17986928011504));
#37011=CARTESIAN_POINT('Ctrl Pts',(-37.6855914133007,45.6,6.11991285341004));
#37012=CARTESIAN_POINT('Ctrl Pts',(-37.518924746634,45.6,1.29812560709619E-15));
#37013=CARTESIAN_POINT('Ctrl Pts',(-37.3522580799673,45.6,-6.11991285341003));
#37014=CARTESIAN_POINT('Ctrl Pts',(-37.1855914133007,40.3,-9.17986928011504));
#37015=CARTESIAN_POINT('Ctrl Pts',(-37.018924746634,35.,-12.2398257068201));
#37016=CARTESIAN_POINT('Ctrl Pts',(-36.8522580799673,29.7,-9.17986928011506));
#37017=CARTESIAN_POINT('Ctrl Pts',(-36.6855914133007,24.4,-6.11991285341004));
#37018=CARTESIAN_POINT('Ctrl Pts',(-36.518924746634,24.4,0.));
#37019=CARTESIAN_POINT('Ctrl Pts',(-36.3522580799673,24.4,6.11991285341003));
#37020=CARTESIAN_POINT('Ctrl Pts',(-36.1855914133007,29.7,9.17986928011504));
#37021=CARTESIAN_POINT('Ctrl Pts',(-36.018924746634,35.,12.2398257068201));
#37022=CARTESIAN_POINT('Ctrl Pts',(-35.8522580799673,40.3,9.17986928011504));
#37023=CARTESIAN_POINT('Ctrl Pts',(-35.6855914133007,45.6,6.11991285341004));
#37024=CARTESIAN_POINT('Ctrl Pts',(-35.518924746634,45.6,1.29812560709619E-15));
#37025=CARTESIAN_POINT('Ctrl Pts',(-35.3522580799673,45.6,-6.11991285341003));
#37026=CARTESIAN_POINT('Ctrl Pts',(-35.1855914133007,40.3,-9.17986928011504));
#37027=CARTESIAN_POINT('Ctrl Pts',(-35.018924746634,35.,-12.2398257068201));
#37028=CARTESIAN_POINT('Ctrl Pts',(-34.8522580799673,29.7,-9.17986928011506));
#37029=CARTESIAN_POINT('Ctrl Pts',(-34.6855914133007,24.4,-6.11991285341004));
#37030=CARTESIAN_POINT('Ctrl Pts',(-34.518924746634,24.4,0.));
#37031=CARTESIAN_POINT('Ctrl Pts',(-34.3522580799673,24.4,6.11991285341003));
#37032=CARTESIAN_POINT('Ctrl Pts',(-34.1855914133007,29.7,9.17986928011504));
#37033=CARTESIAN_POINT('Ctrl Pts',(-34.018924746634,35.,12.2398257068201));
#37034=CARTESIAN_POINT('Ctrl Pts',(-33.8522580799673,40.3,9.17986928011504));
#37035=CARTESIAN_POINT('Ctrl Pts',(-33.6855914133007,45.6,6.11991285341004));
#37036=CARTESIAN_POINT('Ctrl Pts',(-33.518924746634,45.6,1.29812560709619E-15));
#37037=CARTESIAN_POINT('Ctrl Pts',(-33.3522580799673,45.6,-6.11991285341003));
#37038=CARTESIAN_POINT('Ctrl Pts',(-33.1855914133007,40.3,-9.17986928011504));
#37039=CARTESIAN_POINT('Ctrl Pts',(-33.018924746634,35.,-12.2398257068201));
#37040=CARTESIAN_POINT('Ctrl Pts',(-32.8522580799673,29.7,-9.17986928011506));
#37041=CARTESIAN_POINT('Ctrl Pts',(-32.6855914133007,24.4,-6.11991285341004));
#37042=CARTESIAN_POINT('Ctrl Pts',(-32.518924746634,24.4,0.));
#37043=CARTESIAN_POINT('Ctrl Pts',(-32.3522580799673,24.4,6.11991285341003));
#37044=CARTESIAN_POINT('Ctrl Pts',(-32.1855914133007,29.7,9.17986928011504));
#37045=CARTESIAN_POINT('Ctrl Pts',(-32.018924746634,35.,12.2398257068201));
#37046=CARTESIAN_POINT('Ctrl Pts',(-31.8522580799674,40.3,9.17986928011504));
#37047=CARTESIAN_POINT('Ctrl Pts',(-31.6855914133007,45.6,6.11991285341004));
#37048=CARTESIAN_POINT('Ctrl Pts',(-31.518924746634,45.6,1.29812560709619E-15));
#37049=CARTESIAN_POINT('Ctrl Pts',(-31.3522580799673,45.6,-6.11991285341003));
#37050=CARTESIAN_POINT('Ctrl Pts',(-31.1855914133007,40.3,-9.17986928011504));
#37051=CARTESIAN_POINT('Ctrl Pts',(-31.018924746634,35.,-12.2398257068201));
#37052=CARTESIAN_POINT('Ctrl Pts',(-30.8522580799673,29.7,-9.17986928011506));
#37053=CARTESIAN_POINT('Ctrl Pts',(-30.6855914133007,24.4,-6.11991285341004));
#37054=CARTESIAN_POINT('Ctrl Pts',(-30.518924746634,24.4,0.));
#37055=CARTESIAN_POINT('Ctrl Pts',(-30.3522580799673,24.4,6.11991285341003));
#37056=CARTESIAN_POINT('Ctrl Pts',(-30.1855914133007,29.7,9.17986928011504));
#37057=CARTESIAN_POINT('Ctrl Pts',(-30.018924746634,35.,12.2398257068201));
#37058=CARTESIAN_POINT('Ctrl Pts',(-29.8522580799673,40.3,9.17986928011504));
#37059=CARTESIAN_POINT('Ctrl Pts',(-29.6855914133007,45.6,6.11991285341004));
#37060=CARTESIAN_POINT('Ctrl Pts',(-29.518924746634,45.6,1.29812560709619E-15));
#37061=CARTESIAN_POINT('Ctrl Pts',(-29.3522580799673,45.6,-6.11991285341003));
#37062=CARTESIAN_POINT('Ctrl Pts',(-29.1855914133007,40.3,-9.17986928011504));
#37063=CARTESIAN_POINT('Ctrl Pts',(-29.018924746634,35.,-12.2398257068201));
#37064=CARTESIAN_POINT('Ctrl Pts',(-28.8522580799673,29.7,-9.17986928011506));
#37065=CARTESIAN_POINT('Ctrl Pts',(-28.6855914133007,24.4,-6.11991285341004));
#37066=CARTESIAN_POINT('Ctrl Pts',(-28.518924746634,24.4,0.));
#37067=CARTESIAN_POINT('Ctrl Pts',(-28.3522580799673,24.4,6.11991285341003));
#37068=CARTESIAN_POINT('Ctrl Pts',(-28.1855914133007,29.7,9.17986928011504));
#37069=CARTESIAN_POINT('Ctrl Pts',(-28.018924746634,35.,12.2398257068201));
#37070=CARTESIAN_POINT('Ctrl Pts',(-27.8522580799673,40.3,9.17986928011504));
#37071=CARTESIAN_POINT('Ctrl Pts',(-27.6855914133007,45.6,6.11991285341004));
#37072=CARTESIAN_POINT('Ctrl Pts',(-27.518924746634,45.6,1.29812560709619E-15));
#37073=CARTESIAN_POINT('Ctrl Pts',(-27.3522580799673,45.6,-6.11991285341003));
#37074=CARTESIAN_POINT('Ctrl Pts',(-27.1855914133007,40.3,-9.17986928011504));
#37075=CARTESIAN_POINT('Ctrl Pts',(-27.018924746634,35.,-12.2398257068201));
#37076=CARTESIAN_POINT('Ctrl Pts',(-26.8522580799673,29.7,-9.17986928011506));
#37077=CARTESIAN_POINT('Ctrl Pts',(-26.6855914133007,24.4,-6.11991285341004));
#37078=CARTESIAN_POINT('Ctrl Pts',(-26.518924746634,24.4,0.));
#37079=CARTESIAN_POINT('Ctrl Pts',(-26.3522580799673,24.4,6.11991285341003));
#37080=CARTESIAN_POINT('Ctrl Pts',(-26.1855914133007,29.7,9.17986928011504));
#37081=CARTESIAN_POINT('Ctrl Pts',(-26.018924746634,35.,12.2398257068201));
#37082=CARTESIAN_POINT('Ctrl Pts',(-25.8522580799673,40.3,9.17986928011504));
#37083=CARTESIAN_POINT('Ctrl Pts',(-25.6855914133007,45.6,6.11991285341004));
#37084=CARTESIAN_POINT('Ctrl Pts',(-25.518924746634,45.6,1.29812560709619E-15));
#37085=CARTESIAN_POINT('Ctrl Pts',(-25.3522580799673,45.6,-6.11991285341003));
#37086=CARTESIAN_POINT('Ctrl Pts',(-25.1855914133007,40.3,-9.17986928011504));
#37087=CARTESIAN_POINT('Ctrl Pts',(-25.018924746634,35.,-12.2398257068201));
#37088=CARTESIAN_POINT('Ctrl Pts',(-24.8522580799673,29.7,-9.17986928011506));
#37089=CARTESIAN_POINT('Ctrl Pts',(-24.6855914133007,24.4,-6.11991285341004));
#37090=CARTESIAN_POINT('Ctrl Pts',(-24.518924746634,24.4,0.));
#37091=CARTESIAN_POINT('Ctrl Pts',(-24.3522580799673,24.4,6.11991285341003));
#37092=CARTESIAN_POINT('Ctrl Pts',(-24.1855914133007,29.7,9.17986928011504));
#37093=CARTESIAN_POINT('Ctrl Pts',(-24.018924746634,35.,12.2398257068201));
#37094=CARTESIAN_POINT('Ctrl Pts',(-23.8522580799674,40.3,9.17986928011504));
#37095=CARTESIAN_POINT('Ctrl Pts',(-23.6855914133007,45.6,6.11991285341004));
#37096=CARTESIAN_POINT('Ctrl Pts',(-23.518924746634,45.6,1.29812560709619E-15));
#37097=CARTESIAN_POINT('Ctrl Pts',(-23.3522580799673,45.6,-6.11991285341003));
#37098=CARTESIAN_POINT('Ctrl Pts',(-23.1855914133007,40.3,-9.17986928011504));
#37099=CARTESIAN_POINT('Ctrl Pts',(-23.018924746634,35.,-12.2398257068201));
#37100=CARTESIAN_POINT('Ctrl Pts',(-22.8522580799673,29.7,-9.17986928011506));
#37101=CARTESIAN_POINT('Ctrl Pts',(-22.6855914133007,24.4,-6.11991285341004));
#37102=CARTESIAN_POINT('Ctrl Pts',(-22.518924746634,24.4,0.));
#37103=CARTESIAN_POINT('Ctrl Pts',(-22.3522580799673,24.4,6.11991285341003));
#37104=CARTESIAN_POINT('Ctrl Pts',(-22.1855914133007,29.7,9.17986928011504));
#37105=CARTESIAN_POINT('Ctrl Pts',(-22.018924746634,35.,12.2398257068201));
#37106=CARTESIAN_POINT('Ctrl Pts',(-21.8522580799673,40.3,9.17986928011504));
#37107=CARTESIAN_POINT('Ctrl Pts',(-21.6855914133007,45.6,6.11991285341004));
#37108=CARTESIAN_POINT('Ctrl Pts',(-21.518924746634,45.6,1.29812560709619E-15));
#37109=CARTESIAN_POINT('Ctrl Pts',(-21.3522580799673,45.6,-6.11991285341003));
#37110=CARTESIAN_POINT('Ctrl Pts',(-21.1855914133007,40.3,-9.17986928011504));
#37111=CARTESIAN_POINT('Ctrl Pts',(-21.018924746634,35.,-12.2398257068201));
#37112=CARTESIAN_POINT('Ctrl Pts',(-20.8522580799674,29.7,-9.17986928011506));
#37113=CARTESIAN_POINT('Ctrl Pts',(-20.6855914133006,24.4,-6.11991285341004));
#37114=CARTESIAN_POINT('Ctrl Pts',(-20.518924746634,24.4,0.));
#37115=CARTESIAN_POINT('Ctrl Pts',(-20.3522580799673,24.4,6.11991285341003));
#37116=CARTESIAN_POINT('Ctrl Pts',(-20.1855914133007,29.7,9.17986928011504));
#37117=CARTESIAN_POINT('Ctrl Pts',(-20.018924746634,35.,12.2398257068201));
#37118=CARTESIAN_POINT('Ctrl Pts',(-19.8522580799673,40.3,9.17986928011504));
#37119=CARTESIAN_POINT('Ctrl Pts',(-19.6855914133007,45.6,6.11991285341004));
#37120=CARTESIAN_POINT('Ctrl Pts',(-19.518924746634,45.6,1.29812560709619E-15));
#37121=CARTESIAN_POINT('Ctrl Pts',(-19.3522580799673,45.6,-6.11991285341003));
#37122=CARTESIAN_POINT('Ctrl Pts',(-19.1855914133007,40.3,-9.17986928011504));
#37123=CARTESIAN_POINT('Ctrl Pts',(-19.018924746634,35.,-12.2398257068201));
#37124=CARTESIAN_POINT('Ctrl Pts',(-18.8522580799673,29.7,-9.17986928011506));
#37125=CARTESIAN_POINT('Ctrl Pts',(-18.6855914133007,24.4,-6.11991285341004));
#37126=CARTESIAN_POINT('Ctrl Pts',(-18.518924746634,24.4,0.));
#37127=CARTESIAN_POINT('Ctrl Pts',(-38.518924746634,26.,0.));
#37128=CARTESIAN_POINT('Ctrl Pts',(-38.3522580799673,26.,5.19615242270663));
#37129=CARTESIAN_POINT('Ctrl Pts',(-38.1855914133007,30.5,7.79422863405995));
#37130=CARTESIAN_POINT('Ctrl Pts',(-38.018924746634,35.,10.3923048454133));
#37131=CARTESIAN_POINT('Ctrl Pts',(-37.8522580799673,39.5,7.79422863405995));
#37132=CARTESIAN_POINT('Ctrl Pts',(-37.6855914133007,44.,5.19615242270663));
#37133=CARTESIAN_POINT('Ctrl Pts',(-37.518924746634,44.,1.10218211923262E-15));
#37134=CARTESIAN_POINT('Ctrl Pts',(-37.3522580799673,44.,-5.19615242270663));
#37135=CARTESIAN_POINT('Ctrl Pts',(-37.1855914133007,39.5,-7.79422863405995));
#37136=CARTESIAN_POINT('Ctrl Pts',(-37.018924746634,35.,-10.3923048454133));
#37137=CARTESIAN_POINT('Ctrl Pts',(-36.8522580799673,30.5,-7.79422863405995));
#37138=CARTESIAN_POINT('Ctrl Pts',(-36.6855914133007,26.,-5.19615242270663));
#37139=CARTESIAN_POINT('Ctrl Pts',(-36.518924746634,26.,0.));
#37140=CARTESIAN_POINT('Ctrl Pts',(-36.3522580799673,26.,5.19615242270663));
#37141=CARTESIAN_POINT('Ctrl Pts',(-36.1855914133007,30.5,7.79422863405995));
#37142=CARTESIAN_POINT('Ctrl Pts',(-36.018924746634,35.,10.3923048454133));
#37143=CARTESIAN_POINT('Ctrl Pts',(-35.8522580799673,39.5,7.79422863405995));
#37144=CARTESIAN_POINT('Ctrl Pts',(-35.6855914133007,44.,5.19615242270663));
#37145=CARTESIAN_POINT('Ctrl Pts',(-35.518924746634,44.,1.10218211923262E-15));
#37146=CARTESIAN_POINT('Ctrl Pts',(-35.3522580799673,44.,-5.19615242270663));
#37147=CARTESIAN_POINT('Ctrl Pts',(-35.1855914133007,39.5,-7.79422863405995));
#37148=CARTESIAN_POINT('Ctrl Pts',(-35.018924746634,35.,-10.3923048454133));
#37149=CARTESIAN_POINT('Ctrl Pts',(-34.8522580799673,30.5,-7.79422863405995));
#37150=CARTESIAN_POINT('Ctrl Pts',(-34.6855914133007,26.,-5.19615242270663));
#37151=CARTESIAN_POINT('Ctrl Pts',(-34.518924746634,26.,0.));
#37152=CARTESIAN_POINT('Ctrl Pts',(-34.3522580799673,26.,5.19615242270663));
#37153=CARTESIAN_POINT('Ctrl Pts',(-34.1855914133007,30.5,7.79422863405995));
#37154=CARTESIAN_POINT('Ctrl Pts',(-34.018924746634,35.,10.3923048454133));
#37155=CARTESIAN_POINT('Ctrl Pts',(-33.8522580799673,39.5,7.79422863405995));
#37156=CARTESIAN_POINT('Ctrl Pts',(-33.6855914133007,44.,5.19615242270663));
#37157=CARTESIAN_POINT('Ctrl Pts',(-33.518924746634,44.,1.10218211923262E-15));
#37158=CARTESIAN_POINT('Ctrl Pts',(-33.3522580799673,44.,-5.19615242270663));
#37159=CARTESIAN_POINT('Ctrl Pts',(-33.1855914133007,39.5,-7.79422863405995));
#37160=CARTESIAN_POINT('Ctrl Pts',(-33.018924746634,35.,-10.3923048454133));
#37161=CARTESIAN_POINT('Ctrl Pts',(-32.8522580799673,30.5,-7.79422863405995));
#37162=CARTESIAN_POINT('Ctrl Pts',(-32.6855914133007,26.,-5.19615242270663));
#37163=CARTESIAN_POINT('Ctrl Pts',(-32.518924746634,26.,0.));
#37164=CARTESIAN_POINT('Ctrl Pts',(-32.3522580799673,26.,5.19615242270663));
#37165=CARTESIAN_POINT('Ctrl Pts',(-32.1855914133007,30.5,7.79422863405995));
#37166=CARTESIAN_POINT('Ctrl Pts',(-32.018924746634,35.,10.3923048454133));
#37167=CARTESIAN_POINT('Ctrl Pts',(-31.8522580799673,39.5,7.79422863405995));
#37168=CARTESIAN_POINT('Ctrl Pts',(-31.6855914133007,44.,5.19615242270663));
#37169=CARTESIAN_POINT('Ctrl Pts',(-31.518924746634,44.,1.10218211923262E-15));
#37170=CARTESIAN_POINT('Ctrl Pts',(-31.3522580799673,44.,-5.19615242270663));
#37171=CARTESIAN_POINT('Ctrl Pts',(-31.1855914133007,39.5,-7.79422863405995));
#37172=CARTESIAN_POINT('Ctrl Pts',(-31.018924746634,35.,-10.3923048454133));
#37173=CARTESIAN_POINT('Ctrl Pts',(-30.8522580799673,30.5,-7.79422863405995));
#37174=CARTESIAN_POINT('Ctrl Pts',(-30.6855914133007,26.,-5.19615242270663));
#37175=CARTESIAN_POINT('Ctrl Pts',(-30.518924746634,26.,0.));
#37176=CARTESIAN_POINT('Ctrl Pts',(-30.3522580799673,26.,5.19615242270663));
#37177=CARTESIAN_POINT('Ctrl Pts',(-30.1855914133007,30.5,7.79422863405995));
#37178=CARTESIAN_POINT('Ctrl Pts',(-30.018924746634,35.,10.3923048454133));
#37179=CARTESIAN_POINT('Ctrl Pts',(-29.8522580799673,39.5,7.79422863405995));
#37180=CARTESIAN_POINT('Ctrl Pts',(-29.6855914133007,44.,5.19615242270663));
#37181=CARTESIAN_POINT('Ctrl Pts',(-29.518924746634,44.,1.10218211923262E-15));
#37182=CARTESIAN_POINT('Ctrl Pts',(-29.3522580799673,44.,-5.19615242270663));
#37183=CARTESIAN_POINT('Ctrl Pts',(-29.1855914133007,39.5,-7.79422863405995));
#37184=CARTESIAN_POINT('Ctrl Pts',(-29.018924746634,35.,-10.3923048454133));
#37185=CARTESIAN_POINT('Ctrl Pts',(-28.8522580799673,30.5,-7.79422863405995));
#37186=CARTESIAN_POINT('Ctrl Pts',(-28.6855914133007,26.,-5.19615242270663));
#37187=CARTESIAN_POINT('Ctrl Pts',(-28.518924746634,26.,0.));
#37188=CARTESIAN_POINT('Ctrl Pts',(-28.3522580799673,26.,5.19615242270663));
#37189=CARTESIAN_POINT('Ctrl Pts',(-28.1855914133007,30.5,7.79422863405995));
#37190=CARTESIAN_POINT('Ctrl Pts',(-28.018924746634,35.,10.3923048454133));
#37191=CARTESIAN_POINT('Ctrl Pts',(-27.8522580799673,39.5,7.79422863405995));
#37192=CARTESIAN_POINT('Ctrl Pts',(-27.6855914133007,44.,5.19615242270663));
#37193=CARTESIAN_POINT('Ctrl Pts',(-27.518924746634,44.,1.10218211923262E-15));
#37194=CARTESIAN_POINT('Ctrl Pts',(-27.3522580799673,44.,-5.19615242270663));
#37195=CARTESIAN_POINT('Ctrl Pts',(-27.1855914133007,39.5,-7.79422863405995));
#37196=CARTESIAN_POINT('Ctrl Pts',(-27.018924746634,35.,-10.3923048454133));
#37197=CARTESIAN_POINT('Ctrl Pts',(-26.8522580799673,30.5,-7.79422863405995));
#37198=CARTESIAN_POINT('Ctrl Pts',(-26.6855914133007,26.,-5.19615242270663));
#37199=CARTESIAN_POINT('Ctrl Pts',(-26.518924746634,26.,0.));
#37200=CARTESIAN_POINT('Ctrl Pts',(-26.3522580799673,26.,5.19615242270663));
#37201=CARTESIAN_POINT('Ctrl Pts',(-26.1855914133007,30.5,7.79422863405995));
#37202=CARTESIAN_POINT('Ctrl Pts',(-26.018924746634,35.,10.3923048454133));
#37203=CARTESIAN_POINT('Ctrl Pts',(-25.8522580799673,39.5,7.79422863405995));
#37204=CARTESIAN_POINT('Ctrl Pts',(-25.6855914133007,44.,5.19615242270663));
#37205=CARTESIAN_POINT('Ctrl Pts',(-25.518924746634,44.,1.10218211923262E-15));
#37206=CARTESIAN_POINT('Ctrl Pts',(-25.3522580799673,44.,-5.19615242270663));
#37207=CARTESIAN_POINT('Ctrl Pts',(-25.1855914133007,39.5,-7.79422863405995));
#37208=CARTESIAN_POINT('Ctrl Pts',(-25.018924746634,35.,-10.3923048454133));
#37209=CARTESIAN_POINT('Ctrl Pts',(-24.8522580799673,30.5,-7.79422863405995));
#37210=CARTESIAN_POINT('Ctrl Pts',(-24.6855914133007,26.,-5.19615242270663));
#37211=CARTESIAN_POINT('Ctrl Pts',(-24.518924746634,26.,0.));
#37212=CARTESIAN_POINT('Ctrl Pts',(-24.3522580799673,26.,5.19615242270663));
#37213=CARTESIAN_POINT('Ctrl Pts',(-24.1855914133007,30.5,7.79422863405995));
#37214=CARTESIAN_POINT('Ctrl Pts',(-24.018924746634,35.,10.3923048454133));
#37215=CARTESIAN_POINT('Ctrl Pts',(-23.8522580799673,39.5,7.79422863405995));
#37216=CARTESIAN_POINT('Ctrl Pts',(-23.6855914133007,44.,5.19615242270663));
#37217=CARTESIAN_POINT('Ctrl Pts',(-23.518924746634,44.,1.10218211923262E-15));
#37218=CARTESIAN_POINT('Ctrl Pts',(-23.3522580799673,44.,-5.19615242270663));
#37219=CARTESIAN_POINT('Ctrl Pts',(-23.1855914133007,39.5,-7.79422863405995));
#37220=CARTESIAN_POINT('Ctrl Pts',(-23.018924746634,35.,-10.3923048454133));
#37221=CARTESIAN_POINT('Ctrl Pts',(-22.8522580799673,30.5,-7.79422863405995));
#37222=CARTESIAN_POINT('Ctrl Pts',(-22.6855914133007,26.,-5.19615242270663));
#37223=CARTESIAN_POINT('Ctrl Pts',(-22.518924746634,26.,0.));
#37224=CARTESIAN_POINT('Ctrl Pts',(-22.3522580799673,26.,5.19615242270663));
#37225=CARTESIAN_POINT('Ctrl Pts',(-22.1855914133007,30.5,7.79422863405995));
#37226=CARTESIAN_POINT('Ctrl Pts',(-22.018924746634,35.,10.3923048454133));
#37227=CARTESIAN_POINT('Ctrl Pts',(-21.8522580799673,39.5,7.79422863405995));
#37228=CARTESIAN_POINT('Ctrl Pts',(-21.6855914133007,44.,5.19615242270663));
#37229=CARTESIAN_POINT('Ctrl Pts',(-21.518924746634,44.,1.10218211923262E-15));
#37230=CARTESIAN_POINT('Ctrl Pts',(-21.3522580799673,44.,-5.19615242270663));
#37231=CARTESIAN_POINT('Ctrl Pts',(-21.1855914133006,39.5,-7.79422863405995));
#37232=CARTESIAN_POINT('Ctrl Pts',(-21.018924746634,35.,-10.3923048454133));
#37233=CARTESIAN_POINT('Ctrl Pts',(-20.8522580799673,30.5,-7.79422863405995));
#37234=CARTESIAN_POINT('Ctrl Pts',(-20.6855914133007,26.,-5.19615242270663));
#37235=CARTESIAN_POINT('Ctrl Pts',(-20.518924746634,26.,0.));
#37236=CARTESIAN_POINT('Ctrl Pts',(-20.3522580799673,26.,5.19615242270663));
#37237=CARTESIAN_POINT('Ctrl Pts',(-20.1855914133006,30.5,7.79422863405995));
#37238=CARTESIAN_POINT('Ctrl Pts',(-20.018924746634,35.,10.3923048454133));
#37239=CARTESIAN_POINT('Ctrl Pts',(-19.8522580799674,39.5,7.79422863405995));
#37240=CARTESIAN_POINT('Ctrl Pts',(-19.6855914133006,44.,5.19615242270663));
#37241=CARTESIAN_POINT('Ctrl Pts',(-19.518924746634,44.,1.10218211923262E-15));
#37242=CARTESIAN_POINT('Ctrl Pts',(-19.3522580799673,44.,-5.19615242270663));
#37243=CARTESIAN_POINT('Ctrl Pts',(-19.1855914133007,39.5,-7.79422863405995));
#37244=CARTESIAN_POINT('Ctrl Pts',(-19.018924746634,35.,-10.3923048454133));
#37245=CARTESIAN_POINT('Ctrl Pts',(-18.8522580799674,30.5,-7.79422863405995));
#37246=CARTESIAN_POINT('Ctrl Pts',(-18.6855914133007,26.,-5.19615242270663));
#37247=CARTESIAN_POINT('Ctrl Pts',(-18.518924746634,26.,0.));
#37248=CARTESIAN_POINT('Ctrl Pts',(-38.518924746634,27.6,0.));
#37249=CARTESIAN_POINT('Ctrl Pts',(-38.3522580799673,27.6,4.27239199200323));
#37250=CARTESIAN_POINT('Ctrl Pts',(-38.1855914133007,31.3,6.40858798800485));
#37251=CARTESIAN_POINT('Ctrl Pts',(-38.018924746634,35.,8.54478398400645));
#37252=CARTESIAN_POINT('Ctrl Pts',(-37.8522580799673,38.7,6.40858798800485));
#37253=CARTESIAN_POINT('Ctrl Pts',(-37.6855914133007,42.4,4.27239199200323));
#37254=CARTESIAN_POINT('Ctrl Pts',(-37.518924746634,42.4,9.06238631369041E-16));
#37255=CARTESIAN_POINT('Ctrl Pts',(-37.3522580799673,42.4,-4.27239199200323));
#37256=CARTESIAN_POINT('Ctrl Pts',(-37.1855914133007,38.7,-6.40858798800485));
#37257=CARTESIAN_POINT('Ctrl Pts',(-37.018924746634,35.,-8.54478398400645));
#37258=CARTESIAN_POINT('Ctrl Pts',(-36.8522580799673,31.3,-6.40858798800485));
#37259=CARTESIAN_POINT('Ctrl Pts',(-36.6855914133007,27.6,-4.27239199200323));
#37260=CARTESIAN_POINT('Ctrl Pts',(-36.518924746634,27.6,0.));
#37261=CARTESIAN_POINT('Ctrl Pts',(-36.3522580799673,27.6,4.27239199200323));
#37262=CARTESIAN_POINT('Ctrl Pts',(-36.1855914133007,31.3,6.40858798800485));
#37263=CARTESIAN_POINT('Ctrl Pts',(-36.018924746634,35.,8.54478398400645));
#37264=CARTESIAN_POINT('Ctrl Pts',(-35.8522580799673,38.7,6.40858798800485));
#37265=CARTESIAN_POINT('Ctrl Pts',(-35.6855914133007,42.4,4.27239199200323));
#37266=CARTESIAN_POINT('Ctrl Pts',(-35.518924746634,42.4,9.06238631369041E-16));
#37267=CARTESIAN_POINT('Ctrl Pts',(-35.3522580799673,42.4,-4.27239199200323));
#37268=CARTESIAN_POINT('Ctrl Pts',(-35.1855914133007,38.7,-6.40858798800485));
#37269=CARTESIAN_POINT('Ctrl Pts',(-35.018924746634,35.,-8.54478398400645));
#37270=CARTESIAN_POINT('Ctrl Pts',(-34.8522580799673,31.3,-6.40858798800485));
#37271=CARTESIAN_POINT('Ctrl Pts',(-34.6855914133007,27.6,-4.27239199200323));
#37272=CARTESIAN_POINT('Ctrl Pts',(-34.518924746634,27.6,0.));
#37273=CARTESIAN_POINT('Ctrl Pts',(-34.3522580799673,27.6,4.27239199200323));
#37274=CARTESIAN_POINT('Ctrl Pts',(-34.1855914133007,31.3,6.40858798800485));
#37275=CARTESIAN_POINT('Ctrl Pts',(-34.018924746634,35.,8.54478398400645));
#37276=CARTESIAN_POINT('Ctrl Pts',(-33.8522580799673,38.7,6.40858798800485));
#37277=CARTESIAN_POINT('Ctrl Pts',(-33.6855914133007,42.4,4.27239199200323));
#37278=CARTESIAN_POINT('Ctrl Pts',(-33.518924746634,42.4,9.06238631369041E-16));
#37279=CARTESIAN_POINT('Ctrl Pts',(-33.3522580799673,42.4,-4.27239199200323));
#37280=CARTESIAN_POINT('Ctrl Pts',(-33.1855914133007,38.7,-6.40858798800485));
#37281=CARTESIAN_POINT('Ctrl Pts',(-33.018924746634,35.,-8.54478398400645));
#37282=CARTESIAN_POINT('Ctrl Pts',(-32.8522580799673,31.3,-6.40858798800485));
#37283=CARTESIAN_POINT('Ctrl Pts',(-32.6855914133007,27.6,-4.27239199200323));
#37284=CARTESIAN_POINT('Ctrl Pts',(-32.518924746634,27.6,0.));
#37285=CARTESIAN_POINT('Ctrl Pts',(-32.3522580799673,27.6,4.27239199200323));
#37286=CARTESIAN_POINT('Ctrl Pts',(-32.1855914133007,31.3,6.40858798800485));
#37287=CARTESIAN_POINT('Ctrl Pts',(-32.018924746634,35.,8.54478398400645));
#37288=CARTESIAN_POINT('Ctrl Pts',(-31.8522580799674,38.7,6.40858798800485));
#37289=CARTESIAN_POINT('Ctrl Pts',(-31.6855914133007,42.4,4.27239199200323));
#37290=CARTESIAN_POINT('Ctrl Pts',(-31.518924746634,42.4,9.06238631369041E-16));
#37291=CARTESIAN_POINT('Ctrl Pts',(-31.3522580799673,42.4,-4.27239199200323));
#37292=CARTESIAN_POINT('Ctrl Pts',(-31.1855914133007,38.7,-6.40858798800485));
#37293=CARTESIAN_POINT('Ctrl Pts',(-31.018924746634,35.,-8.54478398400645));
#37294=CARTESIAN_POINT('Ctrl Pts',(-30.8522580799673,31.3,-6.40858798800485));
#37295=CARTESIAN_POINT('Ctrl Pts',(-30.6855914133007,27.6,-4.27239199200323));
#37296=CARTESIAN_POINT('Ctrl Pts',(-30.518924746634,27.6,0.));
#37297=CARTESIAN_POINT('Ctrl Pts',(-30.3522580799673,27.6,4.27239199200323));
#37298=CARTESIAN_POINT('Ctrl Pts',(-30.1855914133007,31.3,6.40858798800485));
#37299=CARTESIAN_POINT('Ctrl Pts',(-30.018924746634,35.,8.54478398400645));
#37300=CARTESIAN_POINT('Ctrl Pts',(-29.8522580799673,38.7,6.40858798800485));
#37301=CARTESIAN_POINT('Ctrl Pts',(-29.6855914133007,42.4,4.27239199200323));
#37302=CARTESIAN_POINT('Ctrl Pts',(-29.518924746634,42.4,9.06238631369041E-16));
#37303=CARTESIAN_POINT('Ctrl Pts',(-29.3522580799673,42.4,-4.27239199200323));
#37304=CARTESIAN_POINT('Ctrl Pts',(-29.1855914133007,38.7,-6.40858798800485));
#37305=CARTESIAN_POINT('Ctrl Pts',(-29.018924746634,35.,-8.54478398400645));
#37306=CARTESIAN_POINT('Ctrl Pts',(-28.8522580799673,31.3,-6.40858798800485));
#37307=CARTESIAN_POINT('Ctrl Pts',(-28.6855914133007,27.6,-4.27239199200323));
#37308=CARTESIAN_POINT('Ctrl Pts',(-28.518924746634,27.6,0.));
#37309=CARTESIAN_POINT('Ctrl Pts',(-28.3522580799673,27.6,4.27239199200323));
#37310=CARTESIAN_POINT('Ctrl Pts',(-28.1855914133007,31.3,6.40858798800485));
#37311=CARTESIAN_POINT('Ctrl Pts',(-28.018924746634,35.,8.54478398400645));
#37312=CARTESIAN_POINT('Ctrl Pts',(-27.8522580799673,38.7,6.40858798800485));
#37313=CARTESIAN_POINT('Ctrl Pts',(-27.6855914133007,42.4,4.27239199200323));
#37314=CARTESIAN_POINT('Ctrl Pts',(-27.518924746634,42.4,9.06238631369041E-16));
#37315=CARTESIAN_POINT('Ctrl Pts',(-27.3522580799673,42.4,-4.27239199200323));
#37316=CARTESIAN_POINT('Ctrl Pts',(-27.1855914133007,38.7,-6.40858798800485));
#37317=CARTESIAN_POINT('Ctrl Pts',(-27.018924746634,35.,-8.54478398400645));
#37318=CARTESIAN_POINT('Ctrl Pts',(-26.8522580799673,31.3,-6.40858798800485));
#37319=CARTESIAN_POINT('Ctrl Pts',(-26.6855914133007,27.6,-4.27239199200323));
#37320=CARTESIAN_POINT('Ctrl Pts',(-26.518924746634,27.6,0.));
#37321=CARTESIAN_POINT('Ctrl Pts',(-26.3522580799673,27.6,4.27239199200323));
#37322=CARTESIAN_POINT('Ctrl Pts',(-26.1855914133007,31.3,6.40858798800485));
#37323=CARTESIAN_POINT('Ctrl Pts',(-26.018924746634,35.,8.54478398400645));
#37324=CARTESIAN_POINT('Ctrl Pts',(-25.8522580799673,38.7,6.40858798800485));
#37325=CARTESIAN_POINT('Ctrl Pts',(-25.6855914133007,42.4,4.27239199200323));
#37326=CARTESIAN_POINT('Ctrl Pts',(-25.518924746634,42.4,9.06238631369041E-16));
#37327=CARTESIAN_POINT('Ctrl Pts',(-25.3522580799673,42.4,-4.27239199200323));
#37328=CARTESIAN_POINT('Ctrl Pts',(-25.1855914133007,38.7,-6.40858798800485));
#37329=CARTESIAN_POINT('Ctrl Pts',(-25.018924746634,35.,-8.54478398400645));
#37330=CARTESIAN_POINT('Ctrl Pts',(-24.8522580799673,31.3,-6.40858798800485));
#37331=CARTESIAN_POINT('Ctrl Pts',(-24.6855914133007,27.6,-4.27239199200323));
#37332=CARTESIAN_POINT('Ctrl Pts',(-24.518924746634,27.6,0.));
#37333=CARTESIAN_POINT('Ctrl Pts',(-24.3522580799673,27.6,4.27239199200323));
#37334=CARTESIAN_POINT('Ctrl Pts',(-24.1855914133007,31.3,6.40858798800485));
#37335=CARTESIAN_POINT('Ctrl Pts',(-24.018924746634,35.,8.54478398400645));
#37336=CARTESIAN_POINT('Ctrl Pts',(-23.8522580799674,38.7,6.40858798800485));
#37337=CARTESIAN_POINT('Ctrl Pts',(-23.6855914133007,42.4,4.27239199200323));
#37338=CARTESIAN_POINT('Ctrl Pts',(-23.518924746634,42.4,9.06238631369041E-16));
#37339=CARTESIAN_POINT('Ctrl Pts',(-23.3522580799673,42.4,-4.27239199200323));
#37340=CARTESIAN_POINT('Ctrl Pts',(-23.1855914133007,38.7,-6.40858798800485));
#37341=CARTESIAN_POINT('Ctrl Pts',(-23.018924746634,35.,-8.54478398400645));
#37342=CARTESIAN_POINT('Ctrl Pts',(-22.8522580799673,31.3,-6.40858798800485));
#37343=CARTESIAN_POINT('Ctrl Pts',(-22.6855914133007,27.6,-4.27239199200323));
#37344=CARTESIAN_POINT('Ctrl Pts',(-22.518924746634,27.6,0.));
#37345=CARTESIAN_POINT('Ctrl Pts',(-22.3522580799673,27.6,4.27239199200323));
#37346=CARTESIAN_POINT('Ctrl Pts',(-22.1855914133007,31.3,6.40858798800485));
#37347=CARTESIAN_POINT('Ctrl Pts',(-22.018924746634,35.,8.54478398400645));
#37348=CARTESIAN_POINT('Ctrl Pts',(-21.8522580799673,38.7,6.40858798800485));
#37349=CARTESIAN_POINT('Ctrl Pts',(-21.6855914133007,42.4,4.27239199200323));
#37350=CARTESIAN_POINT('Ctrl Pts',(-21.518924746634,42.4,9.06238631369041E-16));
#37351=CARTESIAN_POINT('Ctrl Pts',(-21.3522580799673,42.4,-4.27239199200323));
#37352=CARTESIAN_POINT('Ctrl Pts',(-21.1855914133007,38.7,-6.40858798800485));
#37353=CARTESIAN_POINT('Ctrl Pts',(-21.018924746634,35.,-8.54478398400645));
#37354=CARTESIAN_POINT('Ctrl Pts',(-20.8522580799674,31.3,-6.40858798800485));
#37355=CARTESIAN_POINT('Ctrl Pts',(-20.6855914133006,27.6,-4.27239199200323));
#37356=CARTESIAN_POINT('Ctrl Pts',(-20.518924746634,27.6,0.));
#37357=CARTESIAN_POINT('Ctrl Pts',(-20.3522580799673,27.6,4.27239199200323));
#37358=CARTESIAN_POINT('Ctrl Pts',(-20.1855914133007,31.3,6.40858798800485));
#37359=CARTESIAN_POINT('Ctrl Pts',(-20.018924746634,35.,8.54478398400645));
#37360=CARTESIAN_POINT('Ctrl Pts',(-19.8522580799673,38.7,6.40858798800485));
#37361=CARTESIAN_POINT('Ctrl Pts',(-19.6855914133007,42.4,4.27239199200323));
#37362=CARTESIAN_POINT('Ctrl Pts',(-19.518924746634,42.4,9.06238631369041E-16));
#37363=CARTESIAN_POINT('Ctrl Pts',(-19.3522580799673,42.4,-4.27239199200323));
#37364=CARTESIAN_POINT('Ctrl Pts',(-19.1855914133007,38.7,-6.40858798800485));
#37365=CARTESIAN_POINT('Ctrl Pts',(-19.018924746634,35.,-8.54478398400645));
#37366=CARTESIAN_POINT('Ctrl Pts',(-18.8522580799673,31.3,-6.40858798800485));
#37367=CARTESIAN_POINT('Ctrl Pts',(-18.6855914133007,27.6,-4.27239199200323));
#37368=CARTESIAN_POINT('Ctrl Pts',(-18.518924746634,27.6,0.));
#37369=CARTESIAN_POINT('Ctrl Pts',(-36.918924746634,27.6,0.));
#37370=CARTESIAN_POINT('Ctrl Pts',(-36.7522580799673,27.6,4.27239199200323));
#37371=CARTESIAN_POINT('Ctrl Pts',(-36.5855914133007,31.3,6.40858798800485));
#37372=CARTESIAN_POINT('Ctrl Pts',(-36.418924746634,35.,8.54478398400645));
#37373=CARTESIAN_POINT('Ctrl Pts',(-36.2522580799673,38.7,6.40858798800485));
#37374=CARTESIAN_POINT('Ctrl Pts',(-36.0855914133007,42.4,4.27239199200323));
#37375=CARTESIAN_POINT('Ctrl Pts',(-35.918924746634,42.4,9.06238631369041E-16));
#37376=CARTESIAN_POINT('Ctrl Pts',(-35.7522580799673,42.4,-4.27239199200323));
#37377=CARTESIAN_POINT('Ctrl Pts',(-35.5855914133007,38.7,-6.40858798800485));
#37378=CARTESIAN_POINT('Ctrl Pts',(-35.418924746634,35.,-8.54478398400645));
#37379=CARTESIAN_POINT('Ctrl Pts',(-35.2522580799673,31.3,-6.40858798800485));
#37380=CARTESIAN_POINT('Ctrl Pts',(-35.0855914133007,27.6,-4.27239199200323));
#37381=CARTESIAN_POINT('Ctrl Pts',(-34.918924746634,27.6,0.));
#37382=CARTESIAN_POINT('Ctrl Pts',(-34.7522580799673,27.6,4.27239199200323));
#37383=CARTESIAN_POINT('Ctrl Pts',(-34.5855914133007,31.3,6.40858798800485));
#37384=CARTESIAN_POINT('Ctrl Pts',(-34.418924746634,35.,8.54478398400645));
#37385=CARTESIAN_POINT('Ctrl Pts',(-34.2522580799673,38.7,6.40858798800485));
#37386=CARTESIAN_POINT('Ctrl Pts',(-34.0855914133007,42.4,4.27239199200323));
#37387=CARTESIAN_POINT('Ctrl Pts',(-33.918924746634,42.4,9.06238631369041E-16));
#37388=CARTESIAN_POINT('Ctrl Pts',(-33.7522580799673,42.4,-4.27239199200323));
#37389=CARTESIAN_POINT('Ctrl Pts',(-33.5855914133007,38.7,-6.40858798800485));
#37390=CARTESIAN_POINT('Ctrl Pts',(-33.418924746634,35.,-8.54478398400645));
#37391=CARTESIAN_POINT('Ctrl Pts',(-33.2522580799673,31.3,-6.40858798800485));
#37392=CARTESIAN_POINT('Ctrl Pts',(-33.0855914133007,27.6,-4.27239199200323));
#37393=CARTESIAN_POINT('Ctrl Pts',(-32.918924746634,27.6,0.));
#37394=CARTESIAN_POINT('Ctrl Pts',(-32.7522580799673,27.6,4.27239199200323));
#37395=CARTESIAN_POINT('Ctrl Pts',(-32.5855914133007,31.3,6.40858798800485));
#37396=CARTESIAN_POINT('Ctrl Pts',(-32.418924746634,35.,8.54478398400645));
#37397=CARTESIAN_POINT('Ctrl Pts',(-32.2522580799673,38.7,6.40858798800485));
#37398=CARTESIAN_POINT('Ctrl Pts',(-32.0855914133007,42.4,4.27239199200323));
#37399=CARTESIAN_POINT('Ctrl Pts',(-31.918924746634,42.4,9.06238631369041E-16));
#37400=CARTESIAN_POINT('Ctrl Pts',(-31.7522580799673,42.4,-4.27239199200323));
#37401=CARTESIAN_POINT('Ctrl Pts',(-31.5855914133007,38.7,-6.40858798800485));
#37402=CARTESIAN_POINT('Ctrl Pts',(-31.418924746634,35.,-8.54478398400645));
#37403=CARTESIAN_POINT('Ctrl Pts',(-31.2522580799673,31.3,-6.40858798800485));
#37404=CARTESIAN_POINT('Ctrl Pts',(-31.0855914133007,27.6,-4.27239199200323));
#37405=CARTESIAN_POINT('Ctrl Pts',(-30.918924746634,27.6,0.));
#37406=CARTESIAN_POINT('Ctrl Pts',(-30.7522580799673,27.6,4.27239199200323));
#37407=CARTESIAN_POINT('Ctrl Pts',(-30.5855914133007,31.3,6.40858798800485));
#37408=CARTESIAN_POINT('Ctrl Pts',(-30.418924746634,35.,8.54478398400645));
#37409=CARTESIAN_POINT('Ctrl Pts',(-30.2522580799673,38.7,6.40858798800485));
#37410=CARTESIAN_POINT('Ctrl Pts',(-30.0855914133007,42.4,4.27239199200323));
#37411=CARTESIAN_POINT('Ctrl Pts',(-29.918924746634,42.4,9.06238631369041E-16));
#37412=CARTESIAN_POINT('Ctrl Pts',(-29.7522580799673,42.4,-4.27239199200323));
#37413=CARTESIAN_POINT('Ctrl Pts',(-29.5855914133007,38.7,-6.40858798800485));
#37414=CARTESIAN_POINT('Ctrl Pts',(-29.418924746634,35.,-8.54478398400645));
#37415=CARTESIAN_POINT('Ctrl Pts',(-29.2522580799673,31.3,-6.40858798800485));
#37416=CARTESIAN_POINT('Ctrl Pts',(-29.0855914133007,27.6,-4.27239199200323));
#37417=CARTESIAN_POINT('Ctrl Pts',(-28.918924746634,27.6,0.));
#37418=CARTESIAN_POINT('Ctrl Pts',(-28.7522580799673,27.6,4.27239199200323));
#37419=CARTESIAN_POINT('Ctrl Pts',(-28.5855914133007,31.3,6.40858798800485));
#37420=CARTESIAN_POINT('Ctrl Pts',(-28.418924746634,35.,8.54478398400645));
#37421=CARTESIAN_POINT('Ctrl Pts',(-28.2522580799673,38.7,6.40858798800485));
#37422=CARTESIAN_POINT('Ctrl Pts',(-28.0855914133007,42.4,4.27239199200323));
#37423=CARTESIAN_POINT('Ctrl Pts',(-27.918924746634,42.4,9.06238631369041E-16));
#37424=CARTESIAN_POINT('Ctrl Pts',(-27.7522580799673,42.4,-4.27239199200323));
#37425=CARTESIAN_POINT('Ctrl Pts',(-27.5855914133007,38.7,-6.40858798800485));
#37426=CARTESIAN_POINT('Ctrl Pts',(-27.418924746634,35.,-8.54478398400645));
#37427=CARTESIAN_POINT('Ctrl Pts',(-27.2522580799673,31.3,-6.40858798800485));
#37428=CARTESIAN_POINT('Ctrl Pts',(-27.0855914133007,27.6,-4.27239199200323));
#37429=CARTESIAN_POINT('Ctrl Pts',(-26.918924746634,27.6,0.));
#37430=CARTESIAN_POINT('Ctrl Pts',(-26.7522580799673,27.6,4.27239199200323));
#37431=CARTESIAN_POINT('Ctrl Pts',(-26.5855914133007,31.3,6.40858798800485));
#37432=CARTESIAN_POINT('Ctrl Pts',(-26.418924746634,35.,8.54478398400645));
#37433=CARTESIAN_POINT('Ctrl Pts',(-26.2522580799673,38.7,6.40858798800485));
#37434=CARTESIAN_POINT('Ctrl Pts',(-26.0855914133007,42.4,4.27239199200323));
#37435=CARTESIAN_POINT('Ctrl Pts',(-25.918924746634,42.4,9.06238631369041E-16));
#37436=CARTESIAN_POINT('Ctrl Pts',(-25.7522580799673,42.4,-4.27239199200323));
#37437=CARTESIAN_POINT('Ctrl Pts',(-25.5855914133007,38.7,-6.40858798800485));
#37438=CARTESIAN_POINT('Ctrl Pts',(-25.418924746634,35.,-8.54478398400645));
#37439=CARTESIAN_POINT('Ctrl Pts',(-25.2522580799673,31.3,-6.40858798800485));
#37440=CARTESIAN_POINT('Ctrl Pts',(-25.0855914133007,27.6,-4.27239199200323));
#37441=CARTESIAN_POINT('Ctrl Pts',(-24.918924746634,27.6,0.));
#37442=CARTESIAN_POINT('Ctrl Pts',(-24.7522580799673,27.6,4.27239199200323));
#37443=CARTESIAN_POINT('Ctrl Pts',(-24.5855914133007,31.3,6.40858798800485));
#37444=CARTESIAN_POINT('Ctrl Pts',(-24.418924746634,35.,8.54478398400645));
#37445=CARTESIAN_POINT('Ctrl Pts',(-24.2522580799673,38.7,6.40858798800485));
#37446=CARTESIAN_POINT('Ctrl Pts',(-24.0855914133007,42.4,4.27239199200323));
#37447=CARTESIAN_POINT('Ctrl Pts',(-23.918924746634,42.4,9.06238631369041E-16));
#37448=CARTESIAN_POINT('Ctrl Pts',(-23.7522580799673,42.4,-4.27239199200323));
#37449=CARTESIAN_POINT('Ctrl Pts',(-23.5855914133007,38.7,-6.40858798800485));
#37450=CARTESIAN_POINT('Ctrl Pts',(-23.418924746634,35.,-8.54478398400645));
#37451=CARTESIAN_POINT('Ctrl Pts',(-23.2522580799673,31.3,-6.40858798800485));
#37452=CARTESIAN_POINT('Ctrl Pts',(-23.0855914133007,27.6,-4.27239199200323));
#37453=CARTESIAN_POINT('Ctrl Pts',(-22.918924746634,27.6,0.));
#37454=CARTESIAN_POINT('Ctrl Pts',(-22.7522580799673,27.6,4.27239199200323));
#37455=CARTESIAN_POINT('Ctrl Pts',(-22.5855914133007,31.3,6.40858798800485));
#37456=CARTESIAN_POINT('Ctrl Pts',(-22.418924746634,35.,8.54478398400645));
#37457=CARTESIAN_POINT('Ctrl Pts',(-22.2522580799673,38.7,6.40858798800485));
#37458=CARTESIAN_POINT('Ctrl Pts',(-22.0855914133007,42.4,4.27239199200323));
#37459=CARTESIAN_POINT('Ctrl Pts',(-21.918924746634,42.4,9.06238631369041E-16));
#37460=CARTESIAN_POINT('Ctrl Pts',(-21.7522580799673,42.4,-4.27239199200323));
#37461=CARTESIAN_POINT('Ctrl Pts',(-21.5855914133007,38.7,-6.40858798800485));
#37462=CARTESIAN_POINT('Ctrl Pts',(-21.418924746634,35.,-8.54478398400645));
#37463=CARTESIAN_POINT('Ctrl Pts',(-21.2522580799673,31.3,-6.40858798800485));
#37464=CARTESIAN_POINT('Ctrl Pts',(-21.0855914133007,27.6,-4.27239199200323));
#37465=CARTESIAN_POINT('Ctrl Pts',(-20.918924746634,27.6,0.));
#37466=CARTESIAN_POINT('Ctrl Pts',(-20.7522580799673,27.6,4.27239199200323));
#37467=CARTESIAN_POINT('Ctrl Pts',(-20.5855914133007,31.3,6.40858798800485));
#37468=CARTESIAN_POINT('Ctrl Pts',(-20.418924746634,35.,8.54478398400645));
#37469=CARTESIAN_POINT('Ctrl Pts',(-20.2522580799673,38.7,6.40858798800485));
#37470=CARTESIAN_POINT('Ctrl Pts',(-20.0855914133007,42.4,4.27239199200323));
#37471=CARTESIAN_POINT('Ctrl Pts',(-19.918924746634,42.4,9.06238631369041E-16));
#37472=CARTESIAN_POINT('Ctrl Pts',(-19.7522580799673,42.4,-4.27239199200323));
#37473=CARTESIAN_POINT('Ctrl Pts',(-19.5855914133007,38.7,-6.40858798800485));
#37474=CARTESIAN_POINT('Ctrl Pts',(-19.418924746634,35.,-8.54478398400645));
#37475=CARTESIAN_POINT('Ctrl Pts',(-19.2522580799673,31.3,-6.40858798800485));
#37476=CARTESIAN_POINT('Ctrl Pts',(-19.0855914133006,27.6,-4.27239199200323));
#37477=CARTESIAN_POINT('Ctrl Pts',(-18.918924746634,27.6,0.));
#37478=CARTESIAN_POINT('Ctrl Pts',(-18.7522580799673,27.6,4.27239199200323));
#37479=CARTESIAN_POINT('Ctrl Pts',(-18.5855914133007,31.3,6.40858798800485));
#37480=CARTESIAN_POINT('Ctrl Pts',(-18.418924746634,35.,8.54478398400645));
#37481=CARTESIAN_POINT('Ctrl Pts',(-18.2522580799673,38.7,6.40858798800485));
#37482=CARTESIAN_POINT('Ctrl Pts',(-18.0855914133007,42.4,4.27239199200323));
#37483=CARTESIAN_POINT('Ctrl Pts',(-17.918924746634,42.4,9.06238631369041E-16));
#37484=CARTESIAN_POINT('Ctrl Pts',(-17.7522580799673,42.4,-4.27239199200323));
#37485=CARTESIAN_POINT('Ctrl Pts',(-17.5855914133007,38.7,-6.40858798800485));
#37486=CARTESIAN_POINT('Ctrl Pts',(-17.418924746634,35.,-8.54478398400645));
#37487=CARTESIAN_POINT('Ctrl Pts',(-17.2522580799674,31.3,-6.40858798800485));
#37488=CARTESIAN_POINT('Ctrl Pts',(-17.0855914133007,27.6,-4.27239199200323));
#37489=CARTESIAN_POINT('Ctrl Pts',(-16.918924746634,27.6,0.));
#37490=CARTESIAN_POINT('Ctrl Pts',(-36.918924746634,26.,0.));
#37491=CARTESIAN_POINT('Ctrl Pts',(-36.7522580799673,26.,5.19615242270663));
#37492=CARTESIAN_POINT('Ctrl Pts',(-36.5855914133007,30.5,7.79422863405995));
#37493=CARTESIAN_POINT('Ctrl Pts',(-36.418924746634,35.,10.3923048454133));
#37494=CARTESIAN_POINT('Ctrl Pts',(-36.2522580799673,39.5,7.79422863405995));
#37495=CARTESIAN_POINT('Ctrl Pts',(-36.0855914133007,44.,5.19615242270663));
#37496=CARTESIAN_POINT('Ctrl Pts',(-35.918924746634,44.,1.10218211923262E-15));
#37497=CARTESIAN_POINT('Ctrl Pts',(-35.7522580799673,44.,-5.19615242270663));
#37498=CARTESIAN_POINT('Ctrl Pts',(-35.5855914133007,39.5,-7.79422863405995));
#37499=CARTESIAN_POINT('Ctrl Pts',(-35.418924746634,35.,-10.3923048454133));
#37500=CARTESIAN_POINT('Ctrl Pts',(-35.2522580799673,30.5,-7.79422863405995));
#37501=CARTESIAN_POINT('Ctrl Pts',(-35.0855914133007,26.,-5.19615242270663));
#37502=CARTESIAN_POINT('Ctrl Pts',(-34.918924746634,26.,0.));
#37503=CARTESIAN_POINT('Ctrl Pts',(-34.7522580799673,26.,5.19615242270663));
#37504=CARTESIAN_POINT('Ctrl Pts',(-34.5855914133007,30.5,7.79422863405995));
#37505=CARTESIAN_POINT('Ctrl Pts',(-34.418924746634,35.,10.3923048454133));
#37506=CARTESIAN_POINT('Ctrl Pts',(-34.2522580799673,39.5,7.79422863405995));
#37507=CARTESIAN_POINT('Ctrl Pts',(-34.0855914133007,44.,5.19615242270663));
#37508=CARTESIAN_POINT('Ctrl Pts',(-33.918924746634,44.,1.10218211923262E-15));
#37509=CARTESIAN_POINT('Ctrl Pts',(-33.7522580799673,44.,-5.19615242270663));
#37510=CARTESIAN_POINT('Ctrl Pts',(-33.5855914133007,39.5,-7.79422863405995));
#37511=CARTESIAN_POINT('Ctrl Pts',(-33.418924746634,35.,-10.3923048454133));
#37512=CARTESIAN_POINT('Ctrl Pts',(-33.2522580799673,30.5,-7.79422863405995));
#37513=CARTESIAN_POINT('Ctrl Pts',(-33.0855914133007,26.,-5.19615242270663));
#37514=CARTESIAN_POINT('Ctrl Pts',(-32.918924746634,26.,0.));
#37515=CARTESIAN_POINT('Ctrl Pts',(-32.7522580799673,26.,5.19615242270663));
#37516=CARTESIAN_POINT('Ctrl Pts',(-32.5855914133007,30.5,7.79422863405995));
#37517=CARTESIAN_POINT('Ctrl Pts',(-32.418924746634,35.,10.3923048454133));
#37518=CARTESIAN_POINT('Ctrl Pts',(-32.2522580799673,39.5,7.79422863405995));
#37519=CARTESIAN_POINT('Ctrl Pts',(-32.0855914133007,44.,5.19615242270663));
#37520=CARTESIAN_POINT('Ctrl Pts',(-31.918924746634,44.,1.10218211923262E-15));
#37521=CARTESIAN_POINT('Ctrl Pts',(-31.7522580799673,44.,-5.19615242270663));
#37522=CARTESIAN_POINT('Ctrl Pts',(-31.5855914133007,39.5,-7.79422863405995));
#37523=CARTESIAN_POINT('Ctrl Pts',(-31.418924746634,35.,-10.3923048454133));
#37524=CARTESIAN_POINT('Ctrl Pts',(-31.2522580799673,30.5,-7.79422863405995));
#37525=CARTESIAN_POINT('Ctrl Pts',(-31.0855914133007,26.,-5.19615242270663));
#37526=CARTESIAN_POINT('Ctrl Pts',(-30.918924746634,26.,0.));
#37527=CARTESIAN_POINT('Ctrl Pts',(-30.7522580799673,26.,5.19615242270663));
#37528=CARTESIAN_POINT('Ctrl Pts',(-30.5855914133007,30.5,7.79422863405995));
#37529=CARTESIAN_POINT('Ctrl Pts',(-30.418924746634,35.,10.3923048454133));
#37530=CARTESIAN_POINT('Ctrl Pts',(-30.2522580799673,39.5,7.79422863405995));
#37531=CARTESIAN_POINT('Ctrl Pts',(-30.0855914133007,44.,5.19615242270663));
#37532=CARTESIAN_POINT('Ctrl Pts',(-29.918924746634,44.,1.10218211923262E-15));
#37533=CARTESIAN_POINT('Ctrl Pts',(-29.7522580799673,44.,-5.19615242270663));
#37534=CARTESIAN_POINT('Ctrl Pts',(-29.5855914133007,39.5,-7.79422863405995));
#37535=CARTESIAN_POINT('Ctrl Pts',(-29.418924746634,35.,-10.3923048454133));
#37536=CARTESIAN_POINT('Ctrl Pts',(-29.2522580799673,30.5,-7.79422863405995));
#37537=CARTESIAN_POINT('Ctrl Pts',(-29.0855914133007,26.,-5.19615242270663));
#37538=CARTESIAN_POINT('Ctrl Pts',(-28.918924746634,26.,0.));
#37539=CARTESIAN_POINT('Ctrl Pts',(-28.7522580799673,26.,5.19615242270663));
#37540=CARTESIAN_POINT('Ctrl Pts',(-28.5855914133007,30.5,7.79422863405995));
#37541=CARTESIAN_POINT('Ctrl Pts',(-28.418924746634,35.,10.3923048454133));
#37542=CARTESIAN_POINT('Ctrl Pts',(-28.2522580799673,39.5,7.79422863405995));
#37543=CARTESIAN_POINT('Ctrl Pts',(-28.0855914133007,44.,5.19615242270663));
#37544=CARTESIAN_POINT('Ctrl Pts',(-27.918924746634,44.,1.10218211923262E-15));
#37545=CARTESIAN_POINT('Ctrl Pts',(-27.7522580799673,44.,-5.19615242270663));
#37546=CARTESIAN_POINT('Ctrl Pts',(-27.5855914133007,39.5,-7.79422863405995));
#37547=CARTESIAN_POINT('Ctrl Pts',(-27.418924746634,35.,-10.3923048454133));
#37548=CARTESIAN_POINT('Ctrl Pts',(-27.2522580799673,30.5,-7.79422863405995));
#37549=CARTESIAN_POINT('Ctrl Pts',(-27.0855914133007,26.,-5.19615242270663));
#37550=CARTESIAN_POINT('Ctrl Pts',(-26.918924746634,26.,0.));
#37551=CARTESIAN_POINT('Ctrl Pts',(-26.7522580799673,26.,5.19615242270663));
#37552=CARTESIAN_POINT('Ctrl Pts',(-26.5855914133007,30.5,7.79422863405995));
#37553=CARTESIAN_POINT('Ctrl Pts',(-26.418924746634,35.,10.3923048454133));
#37554=CARTESIAN_POINT('Ctrl Pts',(-26.2522580799673,39.5,7.79422863405995));
#37555=CARTESIAN_POINT('Ctrl Pts',(-26.0855914133007,44.,5.19615242270663));
#37556=CARTESIAN_POINT('Ctrl Pts',(-25.918924746634,44.,1.10218211923262E-15));
#37557=CARTESIAN_POINT('Ctrl Pts',(-25.7522580799673,44.,-5.19615242270663));
#37558=CARTESIAN_POINT('Ctrl Pts',(-25.5855914133007,39.5,-7.79422863405995));
#37559=CARTESIAN_POINT('Ctrl Pts',(-25.418924746634,35.,-10.3923048454133));
#37560=CARTESIAN_POINT('Ctrl Pts',(-25.2522580799673,30.5,-7.79422863405995));
#37561=CARTESIAN_POINT('Ctrl Pts',(-25.0855914133007,26.,-5.19615242270663));
#37562=CARTESIAN_POINT('Ctrl Pts',(-24.918924746634,26.,0.));
#37563=CARTESIAN_POINT('Ctrl Pts',(-24.7522580799673,26.,5.19615242270663));
#37564=CARTESIAN_POINT('Ctrl Pts',(-24.5855914133007,30.5,7.79422863405995));
#37565=CARTESIAN_POINT('Ctrl Pts',(-24.418924746634,35.,10.3923048454133));
#37566=CARTESIAN_POINT('Ctrl Pts',(-24.2522580799673,39.5,7.79422863405995));
#37567=CARTESIAN_POINT('Ctrl Pts',(-24.0855914133007,44.,5.19615242270663));
#37568=CARTESIAN_POINT('Ctrl Pts',(-23.918924746634,44.,1.10218211923262E-15));
#37569=CARTESIAN_POINT('Ctrl Pts',(-23.7522580799673,44.,-5.19615242270663));
#37570=CARTESIAN_POINT('Ctrl Pts',(-23.5855914133007,39.5,-7.79422863405995));
#37571=CARTESIAN_POINT('Ctrl Pts',(-23.418924746634,35.,-10.3923048454133));
#37572=CARTESIAN_POINT('Ctrl Pts',(-23.2522580799673,30.5,-7.79422863405995));
#37573=CARTESIAN_POINT('Ctrl Pts',(-23.0855914133007,26.,-5.19615242270663));
#37574=CARTESIAN_POINT('Ctrl Pts',(-22.918924746634,26.,0.));
#37575=CARTESIAN_POINT('Ctrl Pts',(-22.7522580799673,26.,5.19615242270663));
#37576=CARTESIAN_POINT('Ctrl Pts',(-22.5855914133007,30.5,7.79422863405995));
#37577=CARTESIAN_POINT('Ctrl Pts',(-22.418924746634,35.,10.3923048454133));
#37578=CARTESIAN_POINT('Ctrl Pts',(-22.2522580799674,39.5,7.79422863405995));
#37579=CARTESIAN_POINT('Ctrl Pts',(-22.0855914133007,44.,5.19615242270663));
#37580=CARTESIAN_POINT('Ctrl Pts',(-21.918924746634,44.,1.10218211923262E-15));
#37581=CARTESIAN_POINT('Ctrl Pts',(-21.7522580799673,44.,-5.19615242270663));
#37582=CARTESIAN_POINT('Ctrl Pts',(-21.5855914133006,39.5,-7.79422863405995));
#37583=CARTESIAN_POINT('Ctrl Pts',(-21.418924746634,35.,-10.3923048454133));
#37584=CARTESIAN_POINT('Ctrl Pts',(-21.2522580799673,30.5,-7.79422863405995));
#37585=CARTESIAN_POINT('Ctrl Pts',(-21.0855914133007,26.,-5.19615242270663));
#37586=CARTESIAN_POINT('Ctrl Pts',(-20.918924746634,26.,0.));
#37587=CARTESIAN_POINT('Ctrl Pts',(-20.7522580799673,26.,5.19615242270663));
#37588=CARTESIAN_POINT('Ctrl Pts',(-20.5855914133006,30.5,7.79422863405995));
#37589=CARTESIAN_POINT('Ctrl Pts',(-20.418924746634,35.,10.3923048454133));
#37590=CARTESIAN_POINT('Ctrl Pts',(-20.2522580799673,39.5,7.79422863405995));
#37591=CARTESIAN_POINT('Ctrl Pts',(-20.0855914133007,44.,5.19615242270663));
#37592=CARTESIAN_POINT('Ctrl Pts',(-19.918924746634,44.,1.10218211923262E-15));
#37593=CARTESIAN_POINT('Ctrl Pts',(-19.7522580799674,44.,-5.19615242270663));
#37594=CARTESIAN_POINT('Ctrl Pts',(-19.5855914133006,39.5,-7.79422863405995));
#37595=CARTESIAN_POINT('Ctrl Pts',(-19.418924746634,35.,-10.3923048454133));
#37596=CARTESIAN_POINT('Ctrl Pts',(-19.2522580799674,30.5,-7.79422863405995));
#37597=CARTESIAN_POINT('Ctrl Pts',(-19.0855914133007,26.,-5.19615242270663));
#37598=CARTESIAN_POINT('Ctrl Pts',(-18.918924746634,26.,0.));
#37599=CARTESIAN_POINT('Ctrl Pts',(-18.7522580799673,26.,5.19615242270663));
#37600=CARTESIAN_POINT('Ctrl Pts',(-18.5855914133006,30.5,7.79422863405995));
#37601=CARTESIAN_POINT('Ctrl Pts',(-18.418924746634,35.,10.3923048454133));
#37602=CARTESIAN_POINT('Ctrl Pts',(-18.2522580799673,39.5,7.79422863405995));
#37603=CARTESIAN_POINT('Ctrl Pts',(-18.0855914133006,44.,5.19615242270663));
#37604=CARTESIAN_POINT('Ctrl Pts',(-17.918924746634,44.,1.10218211923262E-15));
#37605=CARTESIAN_POINT('Ctrl Pts',(-17.7522580799673,44.,-5.19615242270663));
#37606=CARTESIAN_POINT('Ctrl Pts',(-17.5855914133006,39.5,-7.79422863405995));
#37607=CARTESIAN_POINT('Ctrl Pts',(-17.418924746634,35.,-10.3923048454133));
#37608=CARTESIAN_POINT('Ctrl Pts',(-17.2522580799673,30.5,-7.79422863405995));
#37609=CARTESIAN_POINT('Ctrl Pts',(-17.0855914133007,26.,-5.19615242270663));
#37610=CARTESIAN_POINT('Ctrl Pts',(-16.918924746634,26.,0.));
#37611=CARTESIAN_POINT('Ctrl Pts',(-38.518924746634,26.,0.));
#37612=CARTESIAN_POINT('Ctrl Pts',(-38.3522580799673,26.,5.19615242270663));
#37613=CARTESIAN_POINT('Ctrl Pts',(-38.1855914133007,30.5,7.79422863405995));
#37614=CARTESIAN_POINT('Ctrl Pts',(-38.018924746634,35.,10.3923048454133));
#37615=CARTESIAN_POINT('Ctrl Pts',(-37.8522580799673,39.5,7.79422863405995));
#37616=CARTESIAN_POINT('Ctrl Pts',(-37.6855914133007,44.,5.19615242270663));
#37617=CARTESIAN_POINT('Ctrl Pts',(-37.518924746634,44.,1.10218211923262E-15));
#37618=CARTESIAN_POINT('Ctrl Pts',(-37.3522580799673,44.,-5.19615242270663));
#37619=CARTESIAN_POINT('Ctrl Pts',(-37.1855914133007,39.5,-7.79422863405995));
#37620=CARTESIAN_POINT('Ctrl Pts',(-37.018924746634,35.,-10.3923048454133));
#37621=CARTESIAN_POINT('Ctrl Pts',(-36.8522580799673,30.5,-7.79422863405995));
#37622=CARTESIAN_POINT('Ctrl Pts',(-36.6855914133007,26.,-5.19615242270663));
#37623=CARTESIAN_POINT('Ctrl Pts',(-36.518924746634,26.,0.));
#37624=CARTESIAN_POINT('Ctrl Pts',(-36.3522580799673,26.,5.19615242270663));
#37625=CARTESIAN_POINT('Ctrl Pts',(-36.1855914133007,30.5,7.79422863405995));
#37626=CARTESIAN_POINT('Ctrl Pts',(-36.018924746634,35.,10.3923048454133));
#37627=CARTESIAN_POINT('Ctrl Pts',(-35.8522580799673,39.5,7.79422863405995));
#37628=CARTESIAN_POINT('Ctrl Pts',(-35.6855914133007,44.,5.19615242270663));
#37629=CARTESIAN_POINT('Ctrl Pts',(-35.518924746634,44.,1.10218211923262E-15));
#37630=CARTESIAN_POINT('Ctrl Pts',(-35.3522580799673,44.,-5.19615242270663));
#37631=CARTESIAN_POINT('Ctrl Pts',(-35.1855914133007,39.5,-7.79422863405995));
#37632=CARTESIAN_POINT('Ctrl Pts',(-35.018924746634,35.,-10.3923048454133));
#37633=CARTESIAN_POINT('Ctrl Pts',(-34.8522580799673,30.5,-7.79422863405995));
#37634=CARTESIAN_POINT('Ctrl Pts',(-34.6855914133007,26.,-5.19615242270663));
#37635=CARTESIAN_POINT('Ctrl Pts',(-34.518924746634,26.,0.));
#37636=CARTESIAN_POINT('Ctrl Pts',(-34.3522580799673,26.,5.19615242270663));
#37637=CARTESIAN_POINT('Ctrl Pts',(-34.1855914133007,30.5,7.79422863405995));
#37638=CARTESIAN_POINT('Ctrl Pts',(-34.018924746634,35.,10.3923048454133));
#37639=CARTESIAN_POINT('Ctrl Pts',(-33.8522580799673,39.5,7.79422863405995));
#37640=CARTESIAN_POINT('Ctrl Pts',(-33.6855914133007,44.,5.19615242270663));
#37641=CARTESIAN_POINT('Ctrl Pts',(-33.518924746634,44.,1.10218211923262E-15));
#37642=CARTESIAN_POINT('Ctrl Pts',(-33.3522580799673,44.,-5.19615242270663));
#37643=CARTESIAN_POINT('Ctrl Pts',(-33.1855914133007,39.5,-7.79422863405995));
#37644=CARTESIAN_POINT('Ctrl Pts',(-33.018924746634,35.,-10.3923048454133));
#37645=CARTESIAN_POINT('Ctrl Pts',(-32.8522580799673,30.5,-7.79422863405995));
#37646=CARTESIAN_POINT('Ctrl Pts',(-32.6855914133007,26.,-5.19615242270663));
#37647=CARTESIAN_POINT('Ctrl Pts',(-32.518924746634,26.,0.));
#37648=CARTESIAN_POINT('Ctrl Pts',(-32.3522580799673,26.,5.19615242270663));
#37649=CARTESIAN_POINT('Ctrl Pts',(-32.1855914133007,30.5,7.79422863405995));
#37650=CARTESIAN_POINT('Ctrl Pts',(-32.018924746634,35.,10.3923048454133));
#37651=CARTESIAN_POINT('Ctrl Pts',(-31.8522580799673,39.5,7.79422863405995));
#37652=CARTESIAN_POINT('Ctrl Pts',(-31.6855914133007,44.,5.19615242270663));
#37653=CARTESIAN_POINT('Ctrl Pts',(-31.518924746634,44.,1.10218211923262E-15));
#37654=CARTESIAN_POINT('Ctrl Pts',(-31.3522580799673,44.,-5.19615242270663));
#37655=CARTESIAN_POINT('Ctrl Pts',(-31.1855914133007,39.5,-7.79422863405995));
#37656=CARTESIAN_POINT('Ctrl Pts',(-31.018924746634,35.,-10.3923048454133));
#37657=CARTESIAN_POINT('Ctrl Pts',(-30.8522580799673,30.5,-7.79422863405995));
#37658=CARTESIAN_POINT('Ctrl Pts',(-30.6855914133007,26.,-5.19615242270663));
#37659=CARTESIAN_POINT('Ctrl Pts',(-30.518924746634,26.,0.));
#37660=CARTESIAN_POINT('Ctrl Pts',(-30.3522580799673,26.,5.19615242270663));
#37661=CARTESIAN_POINT('Ctrl Pts',(-30.1855914133007,30.5,7.79422863405995));
#37662=CARTESIAN_POINT('Ctrl Pts',(-30.018924746634,35.,10.3923048454133));
#37663=CARTESIAN_POINT('Ctrl Pts',(-29.8522580799673,39.5,7.79422863405995));
#37664=CARTESIAN_POINT('Ctrl Pts',(-29.6855914133007,44.,5.19615242270663));
#37665=CARTESIAN_POINT('Ctrl Pts',(-29.518924746634,44.,1.10218211923262E-15));
#37666=CARTESIAN_POINT('Ctrl Pts',(-29.3522580799673,44.,-5.19615242270663));
#37667=CARTESIAN_POINT('Ctrl Pts',(-29.1855914133007,39.5,-7.79422863405995));
#37668=CARTESIAN_POINT('Ctrl Pts',(-29.018924746634,35.,-10.3923048454133));
#37669=CARTESIAN_POINT('Ctrl Pts',(-28.8522580799673,30.5,-7.79422863405995));
#37670=CARTESIAN_POINT('Ctrl Pts',(-28.6855914133007,26.,-5.19615242270663));
#37671=CARTESIAN_POINT('Ctrl Pts',(-28.518924746634,26.,0.));
#37672=CARTESIAN_POINT('Ctrl Pts',(-28.3522580799673,26.,5.19615242270663));
#37673=CARTESIAN_POINT('Ctrl Pts',(-28.1855914133007,30.5,7.79422863405995));
#37674=CARTESIAN_POINT('Ctrl Pts',(-28.018924746634,35.,10.3923048454133));
#37675=CARTESIAN_POINT('Ctrl Pts',(-27.8522580799673,39.5,7.79422863405995));
#37676=CARTESIAN_POINT('Ctrl Pts',(-27.6855914133007,44.,5.19615242270663));
#37677=CARTESIAN_POINT('Ctrl Pts',(-27.518924746634,44.,1.10218211923262E-15));
#37678=CARTESIAN_POINT('Ctrl Pts',(-27.3522580799673,44.,-5.19615242270663));
#37679=CARTESIAN_POINT('Ctrl Pts',(-27.1855914133007,39.5,-7.79422863405995));
#37680=CARTESIAN_POINT('Ctrl Pts',(-27.018924746634,35.,-10.3923048454133));
#37681=CARTESIAN_POINT('Ctrl Pts',(-26.8522580799673,30.5,-7.79422863405995));
#37682=CARTESIAN_POINT('Ctrl Pts',(-26.6855914133007,26.,-5.19615242270663));
#37683=CARTESIAN_POINT('Ctrl Pts',(-26.518924746634,26.,0.));
#37684=CARTESIAN_POINT('Ctrl Pts',(-26.3522580799673,26.,5.19615242270663));
#37685=CARTESIAN_POINT('Ctrl Pts',(-26.1855914133007,30.5,7.79422863405995));
#37686=CARTESIAN_POINT('Ctrl Pts',(-26.018924746634,35.,10.3923048454133));
#37687=CARTESIAN_POINT('Ctrl Pts',(-25.8522580799673,39.5,7.79422863405995));
#37688=CARTESIAN_POINT('Ctrl Pts',(-25.6855914133007,44.,5.19615242270663));
#37689=CARTESIAN_POINT('Ctrl Pts',(-25.518924746634,44.,1.10218211923262E-15));
#37690=CARTESIAN_POINT('Ctrl Pts',(-25.3522580799673,44.,-5.19615242270663));
#37691=CARTESIAN_POINT('Ctrl Pts',(-25.1855914133007,39.5,-7.79422863405995));
#37692=CARTESIAN_POINT('Ctrl Pts',(-25.018924746634,35.,-10.3923048454133));
#37693=CARTESIAN_POINT('Ctrl Pts',(-24.8522580799673,30.5,-7.79422863405995));
#37694=CARTESIAN_POINT('Ctrl Pts',(-24.6855914133007,26.,-5.19615242270663));
#37695=CARTESIAN_POINT('Ctrl Pts',(-24.518924746634,26.,0.));
#37696=CARTESIAN_POINT('Ctrl Pts',(-24.3522580799673,26.,5.19615242270663));
#37697=CARTESIAN_POINT('Ctrl Pts',(-24.1855914133007,30.5,7.79422863405995));
#37698=CARTESIAN_POINT('Ctrl Pts',(-24.018924746634,35.,10.3923048454133));
#37699=CARTESIAN_POINT('Ctrl Pts',(-23.8522580799673,39.5,7.79422863405995));
#37700=CARTESIAN_POINT('Ctrl Pts',(-23.6855914133007,44.,5.19615242270663));
#37701=CARTESIAN_POINT('Ctrl Pts',(-23.518924746634,44.,1.10218211923262E-15));
#37702=CARTESIAN_POINT('Ctrl Pts',(-23.3522580799673,44.,-5.19615242270663));
#37703=CARTESIAN_POINT('Ctrl Pts',(-23.1855914133007,39.5,-7.79422863405995));
#37704=CARTESIAN_POINT('Ctrl Pts',(-23.018924746634,35.,-10.3923048454133));
#37705=CARTESIAN_POINT('Ctrl Pts',(-22.8522580799673,30.5,-7.79422863405995));
#37706=CARTESIAN_POINT('Ctrl Pts',(-22.6855914133007,26.,-5.19615242270663));
#37707=CARTESIAN_POINT('Ctrl Pts',(-22.518924746634,26.,0.));
#37708=CARTESIAN_POINT('Ctrl Pts',(-22.3522580799673,26.,5.19615242270663));
#37709=CARTESIAN_POINT('Ctrl Pts',(-22.1855914133007,30.5,7.79422863405995));
#37710=CARTESIAN_POINT('Ctrl Pts',(-22.018924746634,35.,10.3923048454133));
#37711=CARTESIAN_POINT('Ctrl Pts',(-21.8522580799673,39.5,7.79422863405995));
#37712=CARTESIAN_POINT('Ctrl Pts',(-21.6855914133007,44.,5.19615242270663));
#37713=CARTESIAN_POINT('Ctrl Pts',(-21.518924746634,44.,1.10218211923262E-15));
#37714=CARTESIAN_POINT('Ctrl Pts',(-21.3522580799673,44.,-5.19615242270663));
#37715=CARTESIAN_POINT('Ctrl Pts',(-21.1855914133006,39.5,-7.79422863405995));
#37716=CARTESIAN_POINT('Ctrl Pts',(-21.018924746634,35.,-10.3923048454133));
#37717=CARTESIAN_POINT('Ctrl Pts',(-20.8522580799673,30.5,-7.79422863405995));
#37718=CARTESIAN_POINT('Ctrl Pts',(-20.6855914133007,26.,-5.19615242270663));
#37719=CARTESIAN_POINT('Ctrl Pts',(-20.518924746634,26.,0.));
#37720=CARTESIAN_POINT('Ctrl Pts',(-20.3522580799673,26.,5.19615242270663));
#37721=CARTESIAN_POINT('Ctrl Pts',(-20.1855914133006,30.5,7.79422863405995));
#37722=CARTESIAN_POINT('Ctrl Pts',(-20.018924746634,35.,10.3923048454133));
#37723=CARTESIAN_POINT('Ctrl Pts',(-19.8522580799674,39.5,7.79422863405995));
#37724=CARTESIAN_POINT('Ctrl Pts',(-19.6855914133006,44.,5.19615242270663));
#37725=CARTESIAN_POINT('Ctrl Pts',(-19.518924746634,44.,1.10218211923262E-15));
#37726=CARTESIAN_POINT('Ctrl Pts',(-19.3522580799673,44.,-5.19615242270663));
#37727=CARTESIAN_POINT('Ctrl Pts',(-19.1855914133007,39.5,-7.79422863405995));
#37728=CARTESIAN_POINT('Ctrl Pts',(-19.018924746634,35.,-10.3923048454133));
#37729=CARTESIAN_POINT('Ctrl Pts',(-18.8522580799674,30.5,-7.79422863405995));
#37730=CARTESIAN_POINT('Ctrl Pts',(-18.6855914133007,26.,-5.19615242270663));
#37731=CARTESIAN_POINT('Ctrl Pts',(-18.518924746634,26.,-2.20436423846523E-14));
#37732=CARTESIAN_POINT('Ctrl Pts',(-36.918924746634,26.,0.));
#37733=CARTESIAN_POINT('Ctrl Pts',(-36.7522580799673,26.,5.19615242270663));
#37734=CARTESIAN_POINT('Ctrl Pts',(-36.5855914133007,30.5,7.79422863405995));
#37735=CARTESIAN_POINT('Ctrl Pts',(-36.418924746634,35.,10.3923048454133));
#37736=CARTESIAN_POINT('Ctrl Pts',(-36.2522580799673,39.5,7.79422863405995));
#37737=CARTESIAN_POINT('Ctrl Pts',(-36.0855914133007,44.,5.19615242270663));
#37738=CARTESIAN_POINT('Ctrl Pts',(-35.918924746634,44.,1.10218211923262E-15));
#37739=CARTESIAN_POINT('Ctrl Pts',(-35.7522580799673,44.,-5.19615242270663));
#37740=CARTESIAN_POINT('Ctrl Pts',(-35.5855914133007,39.5,-7.79422863405995));
#37741=CARTESIAN_POINT('Ctrl Pts',(-35.418924746634,35.,-10.3923048454133));
#37742=CARTESIAN_POINT('Ctrl Pts',(-35.2522580799673,30.5,-7.79422863405995));
#37743=CARTESIAN_POINT('Ctrl Pts',(-35.0855914133007,26.,-5.19615242270663));
#37744=CARTESIAN_POINT('Ctrl Pts',(-34.918924746634,26.,0.));
#37745=CARTESIAN_POINT('Ctrl Pts',(-34.7522580799673,26.,5.19615242270663));
#37746=CARTESIAN_POINT('Ctrl Pts',(-34.5855914133007,30.5,7.79422863405995));
#37747=CARTESIAN_POINT('Ctrl Pts',(-34.418924746634,35.,10.3923048454133));
#37748=CARTESIAN_POINT('Ctrl Pts',(-34.2522580799673,39.5,7.79422863405995));
#37749=CARTESIAN_POINT('Ctrl Pts',(-34.0855914133007,44.,5.19615242270663));
#37750=CARTESIAN_POINT('Ctrl Pts',(-33.918924746634,44.,1.10218211923262E-15));
#37751=CARTESIAN_POINT('Ctrl Pts',(-33.7522580799673,44.,-5.19615242270663));
#37752=CARTESIAN_POINT('Ctrl Pts',(-33.5855914133007,39.5,-7.79422863405995));
#37753=CARTESIAN_POINT('Ctrl Pts',(-33.418924746634,35.,-10.3923048454133));
#37754=CARTESIAN_POINT('Ctrl Pts',(-33.2522580799673,30.5,-7.79422863405995));
#37755=CARTESIAN_POINT('Ctrl Pts',(-33.0855914133007,26.,-5.19615242270663));
#37756=CARTESIAN_POINT('Ctrl Pts',(-32.918924746634,26.,0.));
#37757=CARTESIAN_POINT('Ctrl Pts',(-32.7522580799673,26.,5.19615242270663));
#37758=CARTESIAN_POINT('Ctrl Pts',(-32.5855914133007,30.5,7.79422863405995));
#37759=CARTESIAN_POINT('Ctrl Pts',(-32.418924746634,35.,10.3923048454133));
#37760=CARTESIAN_POINT('Ctrl Pts',(-32.2522580799673,39.5,7.79422863405995));
#37761=CARTESIAN_POINT('Ctrl Pts',(-32.0855914133007,44.,5.19615242270663));
#37762=CARTESIAN_POINT('Ctrl Pts',(-31.918924746634,44.,1.10218211923262E-15));
#37763=CARTESIAN_POINT('Ctrl Pts',(-31.7522580799673,44.,-5.19615242270663));
#37764=CARTESIAN_POINT('Ctrl Pts',(-31.5855914133007,39.5,-7.79422863405995));
#37765=CARTESIAN_POINT('Ctrl Pts',(-31.418924746634,35.,-10.3923048454133));
#37766=CARTESIAN_POINT('Ctrl Pts',(-31.2522580799673,30.5,-7.79422863405995));
#37767=CARTESIAN_POINT('Ctrl Pts',(-31.0855914133007,26.,-5.19615242270663));
#37768=CARTESIAN_POINT('Ctrl Pts',(-30.918924746634,26.,0.));
#37769=CARTESIAN_POINT('Ctrl Pts',(-30.7522580799673,26.,5.19615242270663));
#37770=CARTESIAN_POINT('Ctrl Pts',(-30.5855914133007,30.5,7.79422863405995));
#37771=CARTESIAN_POINT('Ctrl Pts',(-30.418924746634,35.,10.3923048454133));
#37772=CARTESIAN_POINT('Ctrl Pts',(-30.2522580799673,39.5,7.79422863405995));
#37773=CARTESIAN_POINT('Ctrl Pts',(-30.0855914133007,44.,5.19615242270663));
#37774=CARTESIAN_POINT('Ctrl Pts',(-29.918924746634,44.,1.10218211923262E-15));
#37775=CARTESIAN_POINT('Ctrl Pts',(-29.7522580799673,44.,-5.19615242270663));
#37776=CARTESIAN_POINT('Ctrl Pts',(-29.5855914133007,39.5,-7.79422863405995));
#37777=CARTESIAN_POINT('Ctrl Pts',(-29.418924746634,35.,-10.3923048454133));
#37778=CARTESIAN_POINT('Ctrl Pts',(-29.2522580799673,30.5,-7.79422863405995));
#37779=CARTESIAN_POINT('Ctrl Pts',(-29.0855914133007,26.,-5.19615242270663));
#37780=CARTESIAN_POINT('Ctrl Pts',(-28.918924746634,26.,0.));
#37781=CARTESIAN_POINT('Ctrl Pts',(-28.7522580799673,26.,5.19615242270663));
#37782=CARTESIAN_POINT('Ctrl Pts',(-28.5855914133007,30.5,7.79422863405995));
#37783=CARTESIAN_POINT('Ctrl Pts',(-28.418924746634,35.,10.3923048454133));
#37784=CARTESIAN_POINT('Ctrl Pts',(-28.2522580799673,39.5,7.79422863405995));
#37785=CARTESIAN_POINT('Ctrl Pts',(-28.0855914133007,44.,5.19615242270663));
#37786=CARTESIAN_POINT('Ctrl Pts',(-27.918924746634,44.,1.10218211923262E-15));
#37787=CARTESIAN_POINT('Ctrl Pts',(-27.7522580799673,44.,-5.19615242270663));
#37788=CARTESIAN_POINT('Ctrl Pts',(-27.5855914133007,39.5,-7.79422863405995));
#37789=CARTESIAN_POINT('Ctrl Pts',(-27.418924746634,35.,-10.3923048454133));
#37790=CARTESIAN_POINT('Ctrl Pts',(-27.2522580799673,30.5,-7.79422863405995));
#37791=CARTESIAN_POINT('Ctrl Pts',(-27.0855914133007,26.,-5.19615242270663));
#37792=CARTESIAN_POINT('Ctrl Pts',(-26.918924746634,26.,0.));
#37793=CARTESIAN_POINT('Ctrl Pts',(-26.7522580799673,26.,5.19615242270663));
#37794=CARTESIAN_POINT('Ctrl Pts',(-26.5855914133007,30.5,7.79422863405995));
#37795=CARTESIAN_POINT('Ctrl Pts',(-26.418924746634,35.,10.3923048454133));
#37796=CARTESIAN_POINT('Ctrl Pts',(-26.2522580799673,39.5,7.79422863405995));
#37797=CARTESIAN_POINT('Ctrl Pts',(-26.0855914133007,44.,5.19615242270663));
#37798=CARTESIAN_POINT('Ctrl Pts',(-25.918924746634,44.,1.10218211923262E-15));
#37799=CARTESIAN_POINT('Ctrl Pts',(-25.7522580799673,44.,-5.19615242270663));
#37800=CARTESIAN_POINT('Ctrl Pts',(-25.5855914133007,39.5,-7.79422863405995));
#37801=CARTESIAN_POINT('Ctrl Pts',(-25.418924746634,35.,-10.3923048454133));
#37802=CARTESIAN_POINT('Ctrl Pts',(-25.2522580799673,30.5,-7.79422863405995));
#37803=CARTESIAN_POINT('Ctrl Pts',(-25.0855914133007,26.,-5.19615242270663));
#37804=CARTESIAN_POINT('Ctrl Pts',(-24.918924746634,26.,0.));
#37805=CARTESIAN_POINT('Ctrl Pts',(-24.7522580799673,26.,5.19615242270663));
#37806=CARTESIAN_POINT('Ctrl Pts',(-24.5855914133007,30.5,7.79422863405995));
#37807=CARTESIAN_POINT('Ctrl Pts',(-24.418924746634,35.,10.3923048454133));
#37808=CARTESIAN_POINT('Ctrl Pts',(-24.2522580799673,39.5,7.79422863405995));
#37809=CARTESIAN_POINT('Ctrl Pts',(-24.0855914133007,44.,5.19615242270663));
#37810=CARTESIAN_POINT('Ctrl Pts',(-23.918924746634,44.,1.10218211923262E-15));
#37811=CARTESIAN_POINT('Ctrl Pts',(-23.7522580799673,44.,-5.19615242270663));
#37812=CARTESIAN_POINT('Ctrl Pts',(-23.5855914133007,39.5,-7.79422863405995));
#37813=CARTESIAN_POINT('Ctrl Pts',(-23.418924746634,35.,-10.3923048454133));
#37814=CARTESIAN_POINT('Ctrl Pts',(-23.2522580799673,30.5,-7.79422863405995));
#37815=CARTESIAN_POINT('Ctrl Pts',(-23.0855914133007,26.,-5.19615242270663));
#37816=CARTESIAN_POINT('Ctrl Pts',(-22.918924746634,26.,0.));
#37817=CARTESIAN_POINT('Ctrl Pts',(-22.7522580799673,26.,5.19615242270663));
#37818=CARTESIAN_POINT('Ctrl Pts',(-22.5855914133007,30.5,7.79422863405995));
#37819=CARTESIAN_POINT('Ctrl Pts',(-22.418924746634,35.,10.3923048454133));
#37820=CARTESIAN_POINT('Ctrl Pts',(-22.2522580799674,39.5,7.79422863405995));
#37821=CARTESIAN_POINT('Ctrl Pts',(-22.0855914133007,44.,5.19615242270663));
#37822=CARTESIAN_POINT('Ctrl Pts',(-21.918924746634,44.,1.10218211923262E-15));
#37823=CARTESIAN_POINT('Ctrl Pts',(-21.7522580799673,44.,-5.19615242270663));
#37824=CARTESIAN_POINT('Ctrl Pts',(-21.5855914133006,39.5,-7.79422863405995));
#37825=CARTESIAN_POINT('Ctrl Pts',(-21.418924746634,35.,-10.3923048454133));
#37826=CARTESIAN_POINT('Ctrl Pts',(-21.2522580799673,30.5,-7.79422863405995));
#37827=CARTESIAN_POINT('Ctrl Pts',(-21.0855914133007,26.,-5.19615242270663));
#37828=CARTESIAN_POINT('Ctrl Pts',(-20.918924746634,26.,0.));
#37829=CARTESIAN_POINT('Ctrl Pts',(-20.7522580799673,26.,5.19615242270663));
#37830=CARTESIAN_POINT('Ctrl Pts',(-20.5855914133006,30.5,7.79422863405995));
#37831=CARTESIAN_POINT('Ctrl Pts',(-20.418924746634,35.,10.3923048454133));
#37832=CARTESIAN_POINT('Ctrl Pts',(-20.2522580799673,39.5,7.79422863405995));
#37833=CARTESIAN_POINT('Ctrl Pts',(-20.0855914133007,44.,5.19615242270663));
#37834=CARTESIAN_POINT('Ctrl Pts',(-19.918924746634,44.,1.10218211923262E-15));
#37835=CARTESIAN_POINT('Ctrl Pts',(-19.7522580799674,44.,-5.19615242270663));
#37836=CARTESIAN_POINT('Ctrl Pts',(-19.5855914133006,39.5,-7.79422863405995));
#37837=CARTESIAN_POINT('Ctrl Pts',(-19.418924746634,35.,-10.3923048454133));
#37838=CARTESIAN_POINT('Ctrl Pts',(-19.2522580799674,30.5,-7.79422863405995));
#37839=CARTESIAN_POINT('Ctrl Pts',(-19.0855914133007,26.,-5.19615242270663));
#37840=CARTESIAN_POINT('Ctrl Pts',(-18.918924746634,26.,0.));
#37841=CARTESIAN_POINT('Ctrl Pts',(-18.7522580799673,26.,5.19615242270663));
#37842=CARTESIAN_POINT('Ctrl Pts',(-18.5855914133006,30.5,7.79422863405995));
#37843=CARTESIAN_POINT('Ctrl Pts',(-18.418924746634,35.,10.3923048454133));
#37844=CARTESIAN_POINT('Ctrl Pts',(-18.2522580799673,39.5,7.79422863405995));
#37845=CARTESIAN_POINT('Ctrl Pts',(-18.0855914133006,44.,5.19615242270663));
#37846=CARTESIAN_POINT('Ctrl Pts',(-17.918924746634,44.,1.10218211923262E-15));
#37847=CARTESIAN_POINT('Ctrl Pts',(-17.7522580799673,44.,-5.19615242270663));
#37848=CARTESIAN_POINT('Ctrl Pts',(-17.5855914133006,39.5,-7.79422863405995));
#37849=CARTESIAN_POINT('Ctrl Pts',(-17.418924746634,35.,-10.3923048454133));
#37850=CARTESIAN_POINT('Ctrl Pts',(-17.2522580799673,30.5,-7.79422863405995));
#37851=CARTESIAN_POINT('Ctrl Pts',(-17.0855914133007,26.,-5.19615242270663));
#37852=CARTESIAN_POINT('Ctrl Pts',(-16.918924746634,26.,-2.20436423846523E-14));
#37853=CARTESIAN_POINT('Ctrl Pts',(-16.9340264307573,17.163528852123,6.73969634090002));
#37854=CARTESIAN_POINT('Ctrl Pts',(-16.9457712867961,17.2557485214382,6.26075296190838));
#37855=CARTESIAN_POINT('Ctrl Pts',(-17.4245878781802,17.16390605946,6.24262002709426));
#37856=CARTESIAN_POINT('Ctrl Pts',(-16.9238487697737,17.1121753468508,6.73379116642023));
#37857=CARTESIAN_POINT('Ctrl Pts',(-16.9318068964855,17.2064962780678,6.25102883540689));
#37858=CARTESIAN_POINT('Ctrl Pts',(-17.420771254245,17.144754794966,6.23883889336594));
#37859=CARTESIAN_POINT('Ctrl Pts',(-16.9188836705717,17.0606673879271,6.72780634103384));
#37860=CARTESIAN_POINT('Ctrl Pts',(-16.9228736444101,17.1565405083055,6.24116580803177));
#37861=CARTESIAN_POINT('Ctrl Pts',(-17.4189093402838,17.1255458393,6.23504636936957));
#37862=CARTESIAN_POINT('Ctrl Pts',(-16.9189456649685,16.983243156343,6.7187202593339));
#37863=CARTESIAN_POINT('Ctrl Pts',(-16.9168638503772,17.0804387429173,6.22614064079103));
#37864=CARTESIAN_POINT('Ctrl Pts',(-17.4189325924229,17.0966716564302,6.22934558931084));
#37865=CARTESIAN_POINT('Ctrl Pts',(-16.9202265012116,16.9574044014087,6.7156730067294));
#37866=CARTESIAN_POINT('Ctrl Pts',(-16.9161095341114,17.0547943482532,6.22107753461143));
#37867=CARTESIAN_POINT('Ctrl Pts',(-17.4194128979399,17.0870354499882,6.22744306296841));
#37868=CARTESIAN_POINT('Ctrl Pts',(-16.9240802930149,16.9185992377109,6.71107449121992));
#37869=CARTESIAN_POINT('Ctrl Pts',(-16.9169275550253,17.0160227636108,6.21342265905803));
#37870=CARTESIAN_POINT('Ctrl Pts',(-17.4208580798572,17.0725635360787,6.22458579775681));
#37871=CARTESIAN_POINT('Ctrl Pts',(-16.9256893119182,16.905644695499,6.70953565876855));
#37872=CARTESIAN_POINT('Ctrl Pts',(-16.9175289419495,17.0030164596971,6.21085475684852));
#37873=CARTESIAN_POINT('Ctrl Pts',(-17.4214614628586,17.0677322859808,6.22363193892933));
#37874=CARTESIAN_POINT('Ctrl Pts',(-16.9295597285367,16.8797683534593,6.70645460032402));
#37875=CARTESIAN_POINT('Ctrl Pts',(-16.919402781573,16.9769365576265,6.20570566617719));
#37876=CARTESIAN_POINT('Ctrl Pts',(-17.4229128606045,17.0580819710591,6.22172662707637));
#37877=CARTESIAN_POINT('Ctrl Pts',(-16.9318080465975,16.8669299669448,6.70492231261218));
#37878=CARTESIAN_POINT('Ctrl Pts',(-16.9206699203638,16.9639474234362,6.20314115387546));
#37879=CARTESIAN_POINT('Ctrl Pts',(-17.4237559870977,17.0532940171532,6.2207813164412));
#37880=CARTESIAN_POINT('Ctrl Pts',(-16.9445834894833,16.8032276683107,6.69730199287355));
#37881=CARTESIAN_POINT('Ctrl Pts',(-16.928658984358,16.8990583262999,6.1903297620293));
#37882=CARTESIAN_POINT('Ctrl Pts',(-17.4285467632928,17.0295367820529,6.2160908019868));
#37883=CARTESIAN_POINT('Ctrl Pts',(-16.9596689585237,16.7538180319705,6.69133567597977));
#37884=CARTESIAN_POINT('Ctrl Pts',(-16.9402496119177,16.8481169540716,6.18027214203455));
#37885=CARTESIAN_POINT('Ctrl Pts',(-17.4342038179283,17.0111096783419,6.21245264308723));
#37886=CARTESIAN_POINT('Ctrl Pts',(-16.9845527746887,16.6939788697473,6.6840528001532));
#37887=CARTESIAN_POINT('Ctrl Pts',(-16.9613133035777,16.7857105312913,6.16795091749546));
#37888=CARTESIAN_POINT('Ctrl Pts',(-17.4435352591956,16.9887926775086,6.20804648157282));
#37889=CARTESIAN_POINT('Ctrl Pts',(-16.9898335783274,16.6821080424272,6.68260507125331));
#37890=CARTESIAN_POINT('Ctrl Pts',(-16.9658750845434,16.7732516839765,6.16549110248884));
#37891=CARTESIAN_POINT('Ctrl Pts',(-17.4455155553034,16.984365439009,6.2071723888559));
#37892=CARTESIAN_POINT('Ctrl Pts',(-17.0010129029441,16.6585634598165,6.6797280266418));
#37893=CARTESIAN_POINT('Ctrl Pts',(-16.9756875213553,16.7484542773758,6.16059522156661));
#37894=CARTESIAN_POINT('Ctrl Pts',(-17.4497078084659,16.9755844415616,6.20543871087201));
#37895=CARTESIAN_POINT('Ctrl Pts',(-17.0069205341199,16.6468728289804,6.67829663781084));
#37896=CARTESIAN_POINT('Ctrl Pts',(-16.9809474116785,16.7360985023473,6.15815575665741));
#37897=CARTESIAN_POINT('Ctrl Pts',(-17.4519231707424,16.9712243839561,6.20457788202832));
#37898=CARTESIAN_POINT('Ctrl Pts',(-17.0255319975721,16.6122139276746,6.67404499554267));
#37899=CARTESIAN_POINT('Ctrl Pts',(-16.9977536936298,16.6993085573344,6.15089212651984));
#37900=CARTESIAN_POINT('Ctrl Pts',(-17.4589024581334,16.9582981905475,6.20202579645239));
#37901=CARTESIAN_POINT('Ctrl Pts',(-17.0389887268156,16.5898976324254,6.67129663775293));
#37902=CARTESIAN_POINT('Ctrl Pts',(-17.0101778412151,16.6754791025347,6.14618735335466));
#37903=CARTESIAN_POINT('Ctrl Pts',(-17.4639487418597,16.9499751842962,6.20038254205175));
#37904=CARTESIAN_POINT('Ctrl Pts',(-17.0824066515609,16.5252426617237,6.66330736417787));
#37905=CARTESIAN_POINT('Ctrl Pts',(-17.051127346388,16.6058793480108,6.13244591192685));
#37906=CARTESIAN_POINT('Ctrl Pts',(-17.4802304556663,16.925861531581,6.19562165821438));
#37907=CARTESIAN_POINT('Ctrl Pts',(-17.1153868669716,16.4851763244393,6.65831969837799));
#37908=CARTESIAN_POINT('Ctrl Pts',(-17.0831880908469,16.5622697417389,6.12383584060727));
#37909=CARTESIAN_POINT('Ctrl Pts',(-17.4925980312227,16.9109182299925,6.19267132448229));
#37910=CARTESIAN_POINT('Ctrl Pts',(-17.1571321085461,16.443595731894,6.65311644401699));
#37911=CARTESIAN_POINT('Ctrl Pts',(-17.1247289364465,16.5166242121387,6.11482380635895));
#37912=CARTESIAN_POINT('Ctrl Pts',(-17.5082525086683,16.8954100189695,6.18960945774325));
#37913=CARTESIAN_POINT('Ctrl Pts',(-17.1618355598308,16.4390246579602,6.6525440228328));
#37914=CARTESIAN_POINT('Ctrl Pts',(-17.1294344256378,16.5115867952363,6.11382924294728));
#37915=CARTESIAN_POINT('Ctrl Pts',(-17.5100163000558,16.8937051501344,6.18927285662447));
#37916=CARTESIAN_POINT('Ctrl Pts',(-17.171374097915,16.4299815745484,6.65141081135807));
#37917=CARTESIAN_POINT('Ctrl Pts',(-17.1390037634447,16.5016077877741,6.11185903561698));
#37918=CARTESIAN_POINT('Ctrl Pts',(-17.5135932548913,16.8903323645726,6.18860695003381));
#37919=CARTESIAN_POINT('Ctrl Pts',(-17.1762161790489,16.425503359408,6.65084924015553));
#37920=CARTESIAN_POINT('Ctrl Pts',(-17.1438746821593,16.4966594486413,6.11088205929252));
#37921=CARTESIAN_POINT('Ctrl Pts',(-17.5154090352215,16.8886621272269,6.18827718639005));
#37922=CARTESIAN_POINT('Ctrl Pts',(-17.190879548413,16.4122753689571,6.64918933918175));
#37923=CARTESIAN_POINT('Ctrl Pts',(-17.1586695817608,16.4820186331741,6.10799144696816));
#37924=CARTESIAN_POINT('Ctrl Pts',(-17.5209077944372,16.8837284797184,6.18730311070934));
#37925=CARTESIAN_POINT('Ctrl Pts',(-17.2008371206551,16.4037311294511,6.64811568767107));
#37926=CARTESIAN_POINT('Ctrl Pts',(-17.1687645001098,16.4725403371964,6.10612009770977));
#37927=CARTESIAN_POINT('Ctrl Pts',(-17.5246418887157,16.8805417313108,6.18667393440136));
#37928=CARTESIAN_POINT('Ctrl Pts',(-17.2312453506019,16.3789058423747,6.64499241842953));
#37929=CARTESIAN_POINT('Ctrl Pts',(-17.1997603324787,16.4449156410009,6.100666010302));
#37930=CARTESIAN_POINT('Ctrl Pts',(-17.5360449694744,16.8712825880367,6.18484585360074));
#37931=CARTESIAN_POINT('Ctrl Pts',(-17.2522302391352,16.3634303224513,6.64304026443391));
#37932=CARTESIAN_POINT('Ctrl Pts',(-17.2213294853766,16.4276216694408,6.09725157157484));
#37933=CARTESIAN_POINT('Ctrl Pts',(-17.5439143065422,16.8655106243265,6.18370626479344));
#37934=CARTESIAN_POINT('Ctrl Pts',(-17.2956019395641,16.3345930464113,6.63939537781673));
#37935=CARTESIAN_POINT('Ctrl Pts',(-17.2662656597083,16.3952572162235,6.09086168929334));
#37936=CARTESIAN_POINT('Ctrl Pts',(-17.5601786937626,16.8547550179788,6.18158272950716));
#37937=CARTESIAN_POINT('Ctrl Pts',(-17.3179887637184,16.3212313140015,6.63770263755943));
#37938=CARTESIAN_POINT('Ctrl Pts',(-17.2896291828443,16.3801970928505,6.08788829082891));
#37939=CARTESIAN_POINT('Ctrl Pts',(-17.5685737507052,16.8497713855231,6.18059878503843));
#37940=CARTESIAN_POINT('Ctrl Pts',(-17.3526333624528,16.3027934739649,6.63536298725943));
#37941=CARTESIAN_POINT('Ctrl Pts',(-17.3260026650614,16.3593493456032,6.08377221168955));
#37942=CARTESIAN_POINT('Ctrl Pts',(-17.5815654787338,16.8428944620486,6.17924103827948));
#37943=CARTESIAN_POINT('Ctrl Pts',(-17.364359267792,16.296915463442,6.63461640073939));
#37944=CARTESIAN_POINT('Ctrl Pts',(-17.3383566078206,16.3526877545169,6.08245697912365));
#37945=CARTESIAN_POINT('Ctrl Pts',(-17.5859626904173,16.8407020762296,6.17880818414767));
#37946=CARTESIAN_POINT('Ctrl Pts',(-17.3822192836592,16.2885072643732,6.6335476194421));
#37947=CARTESIAN_POINT('Ctrl Pts',(-17.3572223204219,16.3431449083558,6.08057288538689));
#37948=CARTESIAN_POINT('Ctrl Pts',(-17.5926601988439,16.8375659857744,6.17818900950262));
#37949=CARTESIAN_POINT('Ctrl Pts',(-17.3882178337638,16.285772701414,6.63319987789834));
#37950=CARTESIAN_POINT('Ctrl Pts',(-17.3635686188785,16.3400380551801,6.07995948320997));
#37951=CARTESIAN_POINT('Ctrl Pts',(-17.5949096533811,16.8365460418669,6.17798763667366));
#37952=CARTESIAN_POINT('Ctrl Pts',(-17.4003064009864,16.2804414700918,6.6325216769544));
#37953=CARTESIAN_POINT('Ctrl Pts',(-17.3763747964082,16.3339762671101,6.07876267287232));
#37954=CARTESIAN_POINT('Ctrl Pts',(-17.5994428679428,16.8345575960637,6.17759504747957));
#37955=CARTESIAN_POINT('Ctrl Pts',(-17.4064014619839,16.2778429556048,6.63219098038768));
#37956=CARTESIAN_POINT('Ctrl Pts',(-17.3828399484087,16.3310193192068,6.07817886727278));
#37957=CARTESIAN_POINT('Ctrl Pts',(-17.6017285156952,16.8335883975106,6.17740369356977));
#37958=CARTESIAN_POINT('Ctrl Pts',(-17.4613673391331,16.2552073371804,6.6293092707837));
#37959=CARTESIAN_POINT('Ctrl Pts',(-17.4412943532773,16.305207075037,6.07308262169252));
#37960=CARTESIAN_POINT('Ctrl Pts',(-17.6223407123812,16.8251457010694,6.17573680811258));
#37961=CARTESIAN_POINT('Ctrl Pts',(-17.5114824250486,16.2401548090555,6.62738600694331));
#37962=CARTESIAN_POINT('Ctrl Pts',(-17.4949832638486,16.2879639917577,6.06967823010323));
#37963=CARTESIAN_POINT('Ctrl Pts',(-17.6411338750825,16.8195313396363,6.17462833554231));
#37964=CARTESIAN_POINT('Ctrl Pts',(-17.5884810370651,16.2249404862174,6.62544067878907));
#37965=CARTESIAN_POINT('Ctrl Pts',(-17.5778953266643,16.270488978075,6.06622804728844));
#37966=CARTESIAN_POINT('Ctrl Pts',(-17.6700083560242,16.8138566171136,6.17350794556827));
#37967=CARTESIAN_POINT('Ctrl Pts',(-17.61445379365,16.2211054438284,6.6249498806517));
#37968=CARTESIAN_POINT('Ctrl Pts',(-17.6059331605785,16.2660757431219,6.06535671936452));
#37969=CARTESIAN_POINT('Ctrl Pts',(-17.6797481384879,16.8124261864561,6.17322552820585));
#37970=CARTESIAN_POINT('Ctrl Pts',(-17.6538857988551,16.217259998137,6.62445766257136));
#37971=CARTESIAN_POINT('Ctrl Pts',(-17.6485546296303,16.2616476106312,6.06448245014227));
#37972=CARTESIAN_POINT('Ctrl Pts',(-17.6945351416054,16.8109918968226,6.17294234894575));
#37973=CARTESIAN_POINT('Ctrl Pts',(-17.6671432193907,16.2162960247729,6.6243342451152));
#37974=CARTESIAN_POINT('Ctrl Pts',(-17.6628934486627,16.2605370299517,6.06426318242413));
#37975=CARTESIAN_POINT('Ctrl Pts',(-17.6995066741152,16.810632347174,6.1728713611891));
#37976=CARTESIAN_POINT('Ctrl Pts',(-17.6935540371893,16.2150298143844,6.62417212417057));
#37977=CARTESIAN_POINT('Ctrl Pts',(-17.691468213857,16.2590779435578,6.06397510741069));
#37978=CARTESIAN_POINT('Ctrl Pts',(-17.7094107303948,16.8101600586753,6.17277811481509));
#37979=CARTESIAN_POINT('Ctrl Pts',(-17.7067266210675,16.2147239146772,6.62413295366647));
#37980=CARTESIAN_POINT('Ctrl Pts',(-17.7057234775305,16.2587254085436,6.06390550458979));
#37981=CARTESIAN_POINT('Ctrl Pts',(-17.7143504495434,16.8100459686567,6.1727555894295));
#37982=CARTESIAN_POINT('Ctrl Pts',(-17.7724284272708,16.2148007635293,6.6241427921321));
#37983=CARTESIAN_POINT('Ctrl Pts',(-17.7768280969853,16.2588139364961,6.06392298312376));
#37984=CARTESIAN_POINT('Ctrl Pts',(-17.7389886268855,16.8100746189498,6.17276124600583));
#37985=CARTESIAN_POINT('Ctrl Pts',(-17.8244788813812,16.2199564028495,6.62480342778294));
#37986=CARTESIAN_POINT('Ctrl Pts',(-17.8331128420917,16.2647554475499,6.06509604654469));
#37987=CARTESIAN_POINT('Ctrl Pts',(-17.7585075492867,16.8119976109921,6.17314091232356));
#37988=CARTESIAN_POINT('Ctrl Pts',(-17.8889031485325,16.2327695523612,6.62644171019872));
#37989=CARTESIAN_POINT('Ctrl Pts',(-17.90254892953,16.2794864647711,6.06800446787037));
#37990=CARTESIAN_POINT('Ctrl Pts',(-17.7826666468153,16.816776749508,6.17408448249046));
#37991=CARTESIAN_POINT('Ctrl Pts',(-17.9017557691567,16.2356534961519,6.62681033151498));
#37992=CARTESIAN_POINT('Ctrl Pts',(-17.9163762099596,16.2827975605751,6.06865819473137));
#37993=CARTESIAN_POINT('Ctrl Pts',(-17.7874863810826,16.81785241274,6.1742968562754));
#37994=CARTESIAN_POINT('Ctrl Pts',(-17.9273953632276,16.2420759339317,6.62763082558797));
#37995=CARTESIAN_POINT('Ctrl Pts',(-17.9439205439042,16.2901643089726,6.07011265017177));
#37996=CARTESIAN_POINT('Ctrl Pts',(-17.797101226854,16.82024789507,6.17476980880739));
#37997=CARTESIAN_POINT('Ctrl Pts',(-17.9401902056257,16.2456190784938,6.62808328938417));
#37998=CARTESIAN_POINT('Ctrl Pts',(-17.9576446533942,16.294224513599,6.07091427748269));
#37999=CARTESIAN_POINT('Ctrl Pts',(-17.8018992926118,16.8215694340713,6.17503072712393));
#38000=CARTESIAN_POINT('Ctrl Pts',(-17.9780466892305,16.2571128882123,6.62955018787334));
#38001=CARTESIAN_POINT('Ctrl Pts',(-17.9981679747951,16.3073767581212,6.07351099350535));
#38002=CARTESIAN_POINT('Ctrl Pts',(-17.8160954773958,16.8258564334959,6.17587713171108));
#38003=CARTESIAN_POINT('Ctrl Pts',(-18.0027258637711,16.2659587403489,6.63067809312904));
#38004=CARTESIAN_POINT('Ctrl Pts',(-18.0244924260245,16.317478878484,6.07550550765576));
#38005=CARTESIAN_POINT('Ctrl Pts',(-17.825350164657,16.8291557994221,6.17652854268134));
#38006=CARTESIAN_POINT('Ctrl Pts',(-18.0751331263037,16.2959506337827,6.63449608491444));
#38007=CARTESIAN_POINT('Ctrl Pts',(-18.1013159720922,16.3516027063543,6.08224275242306));
#38008=CARTESIAN_POINT('Ctrl Pts',(-17.852502890817,16.8403422289135,6.17873713762098));
#38009=CARTESIAN_POINT('Ctrl Pts',(-18.1212467327399,16.3205175212379,6.63761658916437));
#38010=CARTESIAN_POINT('Ctrl Pts',(-18.1497601127687,16.3794086658638,6.0877326275894));
#38011=CARTESIAN_POINT('Ctrl Pts',(-17.8697955008785,16.8495051762018,6.18054622594794));
#38012=CARTESIAN_POINT('Ctrl Pts',(-18.1706160636699,16.3534706885993,6.6417813765152));
#38013=CARTESIAN_POINT('Ctrl Pts',(-18.2009972681976,16.4164599843371,6.09504786204832));
#38014=CARTESIAN_POINT('Ctrl Pts',(-17.8883089893406,16.8617959232122,6.18297285203741));
#38015=CARTESIAN_POINT('Ctrl Pts',(-18.1760670536863,16.3572075290665,6.64225340483513));
#38016=CARTESIAN_POINT('Ctrl Pts',(-18.2066322253776,16.4206486705888,6.09587485615456));
#38017=CARTESIAN_POINT('Ctrl Pts',(-17.8903531105129,16.863189672331,6.18324802717289));
#38018=CARTESIAN_POINT('Ctrl Pts',(-18.1868377701863,16.3647884998207,6.64321046159106));
#38019=CARTESIAN_POINT('Ctrl Pts',(-18.2177440408947,16.4291367290659,6.09755069767437));
#38020=CARTESIAN_POINT('Ctrl Pts',(-17.8943921317318,16.8660171798007,6.18380627667459));
#38021=CARTESIAN_POINT('Ctrl Pts',(-18.1921652410117,16.3686376965469,6.64369613249193));
#38022=CARTESIAN_POINT('Ctrl Pts',(-18.2232288896621,16.4334416698043,6.09840064450838));
#38023=CARTESIAN_POINT('Ctrl Pts',(-17.8963899309271,16.8674528346187,6.18408972547016));
#38024=CARTESIAN_POINT('Ctrl Pts',(-18.2079758853082,16.380359521441,6.64517424754474));
#38025=CARTESIAN_POINT('Ctrl Pts',(-18.2394674114616,16.4465321648978,6.10098516902028));
#38026=CARTESIAN_POINT('Ctrl Pts',(-17.902318925834,16.8718247643677,6.18495289829289));
#38027=CARTESIAN_POINT('Ctrl Pts',(-18.2182873888224,16.3884062672933,6.64618778634462));
#38028=CARTESIAN_POINT('Ctrl Pts',(-18.250014828929,16.4555003709746,6.10275580857727));
#38029=CARTESIAN_POINT('Ctrl Pts',(-17.9061857359879,16.8748259873231,6.18554544534619));
#38030=CARTESIAN_POINT('Ctrl Pts',(-18.2485461467234,16.4132319441657,6.6493107176117));
#38031=CARTESIAN_POINT('Ctrl Pts',(-18.2808046004885,16.4830834508249,6.10820167945361));
#38032=CARTESIAN_POINT('Ctrl Pts',(-17.917532774601,16.884085261647,6.18737355202065));
#38033=CARTESIAN_POINT('Ctrl Pts',(-18.2678192302634,16.4306946934602,6.65150224599118));
#38034=CARTESIAN_POINT('Ctrl Pts',(-18.3002353052696,16.5024028462849,6.11201600815278));
#38035=CARTESIAN_POINT('Ctrl Pts',(-17.9247601784908,16.8905983462382,6.18865946417705));
#38036=CARTESIAN_POINT('Ctrl Pts',(-18.304585320563,16.4674258171909,6.65609825686814));
#38037=CARTESIAN_POINT('Ctrl Pts',(-18.3369000788844,16.5428190986578,6.11999559900783));
#38038=CARTESIAN_POINT('Ctrl Pts',(-17.9385474613616,16.9042978717687,6.19136423273484));
#38039=CARTESIAN_POINT('Ctrl Pts',(-18.32207835827,16.4866941560064,6.65850274672427));
#38040=CARTESIAN_POINT('Ctrl Pts',(-18.3541350222299,16.5639050113827,6.12415870039582));
#38041=CARTESIAN_POINT('Ctrl Pts',(-17.9451073556682,16.9114842972485,6.19278308608398));
#38042=CARTESIAN_POINT('Ctrl Pts',(-18.3469582555341,16.5169758809527,6.6622690907101));
#38043=CARTESIAN_POINT('Ctrl Pts',(-18.3783360711151,16.5968717741023,6.13066749977414));
#38044=CARTESIAN_POINT('Ctrl Pts',(-17.9544373101362,16.9227782767883,6.1950129151889));
#38045=CARTESIAN_POINT('Ctrl Pts',(-18.3550268290823,16.5273031516405,6.66355157018222));
#38046=CARTESIAN_POINT('Ctrl Pts',(-18.3861205298441,16.6080723020181,6.13287887823903));
#38047=CARTESIAN_POINT('Ctrl Pts',(-17.9574630272311,16.9266299573578,6.19577337251102));
#38048=CARTESIAN_POINT('Ctrl Pts',(-18.3706915223259,16.5484153134749,6.66616886023153));
#38049=CARTESIAN_POINT('Ctrl Pts',(-18.4011144492354,16.6308981776041,6.13738550954182));
#38050=CARTESIAN_POINT('Ctrl Pts',(-17.9633372878401,16.934503971749,6.19732798011414));
#38051=CARTESIAN_POINT('Ctrl Pts',(-18.3782309891514,16.5591238170816,6.66749420161781));
#38052=CARTESIAN_POINT('Ctrl Pts',(-18.4082702147513,16.6424396756498,6.13966420751237));
#38053=CARTESIAN_POINT('Ctrl Pts',(-17.9661645847443,16.9384978169065,6.19811650573006));
#38054=CARTESIAN_POINT('Ctrl Pts',(-18.4144652239087,16.6133698763481,6.67419609590586));
#38055=CARTESIAN_POINT('Ctrl Pts',(-18.4422698693699,16.7005708871118,6.15114135485145));
#38056=CARTESIAN_POINT('Ctrl Pts',(-17.9797524369468,16.9587293525346,6.20211092300537));
#38057=CARTESIAN_POINT('Ctrl Pts',(-18.4388454391431,16.6590429087733,6.67980148969806));
#38058=CARTESIAN_POINT('Ctrl Pts',(-18.4642277040733,16.7490077862942,6.16070450371041));
#38059=CARTESIAN_POINT('Ctrl Pts',(-17.9888950132745,16.975763316277,6.20547402703715));
#38060=CARTESIAN_POINT('Ctrl Pts',(-18.4636539969267,16.7189339970101,6.68708985334279));
#38061=CARTESIAN_POINT('Ctrl Pts',(-18.4853233274594,16.811806410725,6.17310316266067));
#38062=CARTESIAN_POINT('Ctrl Pts',(-17.9981982137564,16.9980996869273,6.20988401283525));
#38063=CARTESIAN_POINT('Ctrl Pts',(-18.4683298236966,16.7310534611065,6.68856175184365));
#38064=CARTESIAN_POINT('Ctrl Pts',(-18.4892098083346,16.8244336013383,6.17559621456002));
#38065=CARTESIAN_POINT('Ctrl Pts',(-17.9999516535622,17.0026196231967,6.21077640735487));
#38066=CARTESIAN_POINT('Ctrl Pts',(-18.4771016880877,16.7555788545222,6.69153398968095));
#38067=CARTESIAN_POINT('Ctrl Pts',(-18.4963362162636,16.8498937457125,6.18062294324687));
#38068=CARTESIAN_POINT('Ctrl Pts',(-18.0032410966494,17.0117663114213,6.21258228557033));
#38069=CARTESIAN_POINT('Ctrl Pts',(-18.4812032176816,16.768003161379,6.69303654757409));
#38070=CARTESIAN_POINT('Ctrl Pts',(-18.4995813969772,16.8627446305905,6.18316016026802));
#38071=CARTESIAN_POINT('Ctrl Pts',(-18.0047791706222,17.0163999130041,6.21349712162379));
#38072=CARTESIAN_POINT('Ctrl Pts',(-18.4925821723103,16.8055904468549,6.69757219653477));
#38073=CARTESIAN_POINT('Ctrl Pts',(-18.5082993306589,16.9014403837458,6.19080006401661));
#38074=CARTESIAN_POINT('Ctrl Pts',(-18.0090462865719,17.030417917443,6.21626476912844));
#38075=CARTESIAN_POINT('Ctrl Pts',(-18.4988883625265,16.8308948943173,6.70061244451219));
#38076=CARTESIAN_POINT('Ctrl Pts',(-18.5127456724536,16.9273229004005,6.19591018385897));
#38077=CARTESIAN_POINT('Ctrl Pts',(-18.0114111023906,17.0398550445677,6.21812799020613));
#38078=CARTESIAN_POINT('Ctrl Pts',(-18.5089809331914,16.8819886542203,6.70672283022605));
#38079=CARTESIAN_POINT('Ctrl Pts',(-18.5189743166287,16.979189821447,6.20615053976939));
#38080=CARTESIAN_POINT('Ctrl Pts',(-18.0151958167961,17.0589100232433,6.22189011372466));
#38081=CARTESIAN_POINT('Ctrl Pts',(-18.5127673002267,16.9077779664103,6.70979297341625));
#38082=CARTESIAN_POINT('Ctrl Pts',(-18.5207667892184,17.0051710504343,6.21128014890083));
#38083=CARTESIAN_POINT('Ctrl Pts',(-18.0166157093195,17.0685278759537,6.22378901639444));
#38084=CARTESIAN_POINT('Ctrl Pts',(-18.51653149759,16.9468304737568,6.71441949514766));
#38085=CARTESIAN_POINT('Ctrl Pts',(-18.5214756795303,17.0442515895124,6.21899602293492));
#38086=CARTESIAN_POINT('Ctrl Pts',(-18.0180272756984,17.0830920314624,6.22666449334457));
#38087=CARTESIAN_POINT('Ctrl Pts',(-18.5174610536025,16.9598642331123,6.71595985693076));
#38088=CARTESIAN_POINT('Ctrl Pts',(-18.5213812087045,17.0572310011096,6.22155861565454));
#38089=CARTESIAN_POINT('Ctrl Pts',(-18.0183758583191,17.0879528012551,6.22762418039891));
#38090=CARTESIAN_POINT('Ctrl Pts',(-18.5186722537819,16.9858429775025,6.71902258829226));
#38091=CARTESIAN_POINT('Ctrl Pts',(-18.5205481857505,17.0830017716537,6.22664667288122));
#38092=CARTESIAN_POINT('Ctrl Pts',(-18.0188300652425,17.0976412129467,6.22953701389521));
#38093=CARTESIAN_POINT('Ctrl Pts',(-18.5189557766232,16.9988067822409,6.7205471885435));
#38094=CARTESIAN_POINT('Ctrl Pts',(-18.5198112791957,17.0958122032461,6.22917590299987));
#38095=CARTESIAN_POINT('Ctrl Pts',(-18.0189363807851,17.1024758738013,6.23049154612614));
#38096=CARTESIAN_POINT('Ctrl Pts',(-18.5187872011184,17.0634999017462,6.72813660661715));
#38097=CARTESIAN_POINT('Ctrl Pts',(-18.5145769287806,17.1593013447143,6.24171089431925));
#38098=CARTESIAN_POINT('Ctrl Pts',(-18.0188731754452,17.1266021766945,6.23525492755391));
#38099=CARTESIAN_POINT('Ctrl Pts',(-18.5136215290469,17.1148550403912,6.73410108134611));
#38100=CARTESIAN_POINT('Ctrl Pts',(-18.5054607669974,17.2090806073982,6.25153907298411));
#38101=CARTESIAN_POINT('Ctrl Pts',(-18.0169360523498,17.1457541379813,6.23903619885366));
#38102=CARTESIAN_POINT('Ctrl Pts',(-18.5008049385582,17.178543935026,6.74142244098528));
#38103=CARTESIAN_POINT('Ctrl Pts',(-18.4879750956344,17.2700726310465,6.26358104534826));
#38104=CARTESIAN_POINT('Ctrl Pts',(-18.0121298155278,17.1695056335805,6.24372558012852));
#38105=CARTESIAN_POINT('Ctrl Pts',(-18.4979208133035,17.1912562328885,6.74287997549926));
#38106=CARTESIAN_POINT('Ctrl Pts',(-18.4841868810595,17.2821639022754,6.26596828789697));
#38107=CARTESIAN_POINT('Ctrl Pts',(-18.0110482760138,17.1742464268863,6.24466157960121));
#38108=CARTESIAN_POINT('Ctrl Pts',(-18.4914973495927,17.2166287983916,6.74578145608233));
#38109=CARTESIAN_POINT('Ctrl Pts',(-18.4759981394833,17.3062060478485,6.27071505370745));
#38110=CARTESIAN_POINT('Ctrl Pts',(-18.0086394683647,17.1837085953516,6.24652974472097));
#38111=CARTESIAN_POINT('Ctrl Pts',(-18.4879753251126,17.2292171975606,6.74721717444261));
#38112=CARTESIAN_POINT('Ctrl Pts',(-18.4716211015665,17.3180893500614,6.27306123585199));
#38113=CARTESIAN_POINT('Ctrl Pts',(-18.0073187104683,17.1884031726981,6.24745661953651));
#38114=CARTESIAN_POINT('Ctrl Pts',(-18.4765353931923,17.2665465103297,6.75146357848355));
#38115=CARTESIAN_POINT('Ctrl Pts',(-18.4577271501903,17.3531629274733,6.27998599460963));
#38116=CARTESIAN_POINT('Ctrl Pts',(-18.0030287452838,17.2023243430448,6.25020514858282));
#38117=CARTESIAN_POINT('Ctrl Pts',(-18.4677297456344,17.2909162449736,6.75422091139731));
#38118=CARTESIAN_POINT('Ctrl Pts',(-18.4474068235007,17.3759132514684,6.28447770936899));
#38119=CARTESIAN_POINT('Ctrl Pts',(-17.9997266201643,17.2114124977806,6.25199947022725));
#38120=CARTESIAN_POINT('Ctrl Pts',(-18.4378487844442,17.3625079863937,6.76228026019661));
#38121=CARTESIAN_POINT('Ctrl Pts',(-18.4134691558281,17.4421491186173,6.29755500102144));
#38122=CARTESIAN_POINT('Ctrl Pts',(-17.9885212630024,17.2381110500616,6.25727070422638));
#38123=CARTESIAN_POINT('Ctrl Pts',(-18.413342249397,17.4082296127105,6.76737146292247));
#38124=CARTESIAN_POINT('Ctrl Pts',(-18.3868137642132,17.483931249389,6.30580426435083));
#38125=CARTESIAN_POINT('Ctrl Pts',(-17.979331323364,17.2551619032087,6.26063714282115));
#38126=CARTESIAN_POINT('Ctrl Pts',(-18.3693951615143,17.4736551525738,6.77458729194665));
#38127=CARTESIAN_POINT('Ctrl Pts',(-18.3405991802905,17.5430486220348,6.31747611462008));
#38128=CARTESIAN_POINT('Ctrl Pts',(-17.9628511456172,17.279560906992,6.26545436500358));
#38129=CARTESIAN_POINT('Ctrl Pts',(-18.3537632469114,17.4945975063259,6.77688492238546));
#38130=CARTESIAN_POINT('Ctrl Pts',(-18.3244286783927,17.5618163081471,6.32118151647404));
#38131=CARTESIAN_POINT('Ctrl Pts',(-17.9569891815114,17.2873709068913,6.26699633389272));
#38132=CARTESIAN_POINT('Ctrl Pts',(-18.3206591277799,17.5347184100098,6.78126667754031));
#38133=CARTESIAN_POINT('Ctrl Pts',(-18.2906282613387,17.5975559035035,6.32823777061752));
#38134=CARTESIAN_POINT('Ctrl Pts',(-17.9445751422903,17.3023331556006,6.26995040845338));
#38135=CARTESIAN_POINT('Ctrl Pts',(-18.3031766385638,17.5539118752031,6.78335243318941));
#38136=CARTESIAN_POINT('Ctrl Pts',(-18.2729880315817,17.6145513152006,6.33159326311853));
#38137=CARTESIAN_POINT('Ctrl Pts',(-17.9380192073362,17.3094909634119,6.27136361166745));
#38138=CARTESIAN_POINT('Ctrl Pts',(-18.2663596953146,17.590573120573,6.78731950209393));
#38139=CARTESIAN_POINT('Ctrl Pts',(-18.2362359266378,17.6468363652653,6.33796746842275));
#38140=CARTESIAN_POINT('Ctrl Pts',(-17.9242128511607,17.3231630449985,6.2740629618247));
#38141=CARTESIAN_POINT('Ctrl Pts',(-18.2470253297619,17.6080409781332,6.78920081264864));
#38142=CARTESIAN_POINT('Ctrl Pts',(-18.2171237375768,17.6621351487866,6.3409879868012));
#38143=CARTESIAN_POINT('Ctrl Pts',(-17.9169624698265,17.3296773557345,6.27534911606522));
#38144=CARTESIAN_POINT('Ctrl Pts',(-18.2166010903152,17.6329170950227,6.79186951328928));
#38145=CARTESIAN_POINT('Ctrl Pts',(-18.1872989485619,17.683828532514,6.34527102434781));
#38146=CARTESIAN_POINT('Ctrl Pts',(-17.9055533732547,17.3389544402554,6.27718073909949));
#38147=CARTESIAN_POINT('Ctrl Pts',(-18.2062168750825,17.6409916724233,6.79273390499216));
#38148=CARTESIAN_POINT('Ctrl Pts',(-18.1771687996823,17.6908479022576,6.34665689501433));
#38149=CARTESIAN_POINT('Ctrl Pts',(-17.9016592934025,17.3419657104848,6.27777526983833));
#38150=CARTESIAN_POINT('Ctrl Pts',(-18.1849835178449,17.656672005178,6.79440927725295));
#38151=CARTESIAN_POINT('Ctrl Pts',(-18.1565384222284,17.7044471017748,6.34934185568567));
#38152=CARTESIAN_POINT('Ctrl Pts',(-17.8936967872377,17.3478134207786,6.27892981368751));
#38153=CARTESIAN_POINT('Ctrl Pts',(-18.1742117514745,17.6642209160496,6.79521418404731));
#38154=CARTESIAN_POINT('Ctrl Pts',(-18.1461128939455,17.7109787537895,6.35063143370503));
#38155=CARTESIAN_POINT('Ctrl Pts',(-17.8896573717566,17.3506286544074,6.27948563990098));
#38156=CARTESIAN_POINT('Ctrl Pts',(-18.1196129973381,17.7005236924937,6.7990781174034));
#38157=CARTESIAN_POINT('Ctrl Pts',(-18.0935526247991,17.7422665507531,6.35680874614416));
#38158=CARTESIAN_POINT('Ctrl Pts',(-17.8691828474184,17.3641671857882,6.2821586225467));
#38159=CARTESIAN_POINT('Ctrl Pts',(-18.073566038191,17.7250092175285,6.8016618385873));
#38160=CARTESIAN_POINT('Ctrl Pts',(-18.0497217046225,17.7632251779753,6.36094671689349));
#38161=CARTESIAN_POINT('Ctrl Pts',(-17.8519152345038,17.3732987063331,6.2839615061283));
#38162=CARTESIAN_POINT('Ctrl Pts',(-18.0130701585827,17.7499642230801,6.80428434438707));
#38163=CARTESIAN_POINT('Ctrl Pts',(-17.9926453915806,17.7844819967742,6.36514356115633));
#38164=CARTESIAN_POINT('Ctrl Pts',(-17.8292292752308,17.3826053354479,6.28579896230536));
#38165=CARTESIAN_POINT('Ctrl Pts',(-18.0008227990897,17.7546700742571,6.80477818859267));
#38166=CARTESIAN_POINT('Ctrl Pts',(-17.9811297306172,17.7884796711135,6.36593284278751));
#38167=CARTESIAN_POINT('Ctrl Pts',(-17.8246365175473,17.3843603279786,6.28614545960597));
#38168=CARTESIAN_POINT('Ctrl Pts',(-17.9760268452319,17.7635021372388,6.80570402970065));
#38169=CARTESIAN_POINT('Ctrl Pts',(-17.9578627436139,17.7959726092415,6.36741221252255));
#38170=CARTESIAN_POINT('Ctrl Pts',(-17.8153380323659,17.3876541288755,6.28679577184356));
#38171=CARTESIAN_POINT('Ctrl Pts',(-17.9634548231814,17.7676353220123,6.80613675524105));
#38172=CARTESIAN_POINT('Ctrl Pts',(-17.9460886325703,17.7994744891973,6.36810360689066));
#38173=CARTESIAN_POINT('Ctrl Pts',(-17.8106235240595,17.3891955494437,6.28710010252115));
#38174=CARTESIAN_POINT('Ctrl Pts',(-17.9254344120959,17.7790973746866,6.80733565050496));
#38175=CARTESIAN_POINT('Ctrl Pts',(-17.9105547741728,17.8091716890774,6.37001817548471));
#38176=CARTESIAN_POINT('Ctrl Pts',(-17.7963658737417,17.3934701994542,6.28794406889925));
#38177=CARTESIAN_POINT('Ctrl Pts',(-17.8999087430931,17.7854283478246,6.80799626184293));
#38178=CARTESIAN_POINT('Ctrl Pts',(-17.886766663715,17.8145173455381,6.37107359623513));
#38179=CARTESIAN_POINT('Ctrl Pts',(-17.7867937446671,17.3958312544259,6.28841022425892));
#38180=CARTESIAN_POINT('Ctrl Pts',(-17.8228126864582,17.8006160211639,6.80957942969772));
#38181=CARTESIAN_POINT('Ctrl Pts',(-17.8151219476809,17.8273163816643,6.37360057648762));
#38182=CARTESIAN_POINT('Ctrl Pts',(-17.7578827253461,17.4014953443393,6.28952851498163));
#38183=CARTESIAN_POINT('Ctrl Pts',(-17.7707282072719,17.8057036316249,6.81010758629701));
#38184=CARTESIAN_POINT('Ctrl Pts',(-17.7668735570122,17.8315930628393,6.37444494388912));
#38185=CARTESIAN_POINT('Ctrl Pts',(-17.7383510443547,17.4033927296949,6.28990312563806));
#38186=CARTESIAN_POINT('Ctrl Pts',(-17.7113425373793,17.8056309224566,6.81010002580354));
#38187=CARTESIAN_POINT('Ctrl Pts',(-17.7119066821582,17.8315319119423,6.37443287054956));
#38188=CARTESIAN_POINT('Ctrl Pts',(-17.7160814181658,17.4033655966885,6.28989776862753));
#38189=CARTESIAN_POINT('Ctrl Pts',(-17.7047330456674,17.8055415663399,6.81009073748399));
#38190=CARTESIAN_POINT('Ctrl Pts',(-17.7057888706203,17.8314568157848,6.37441804392472));
#38191=CARTESIAN_POINT('Ctrl Pts',(-17.7136028587132,17.4033322762928,6.28989119000853));
#38192=CARTESIAN_POINT('Ctrl Pts',(-17.6914916361947,17.8051984797874,6.81005506963536));
#38193=CARTESIAN_POINT('Ctrl Pts',(-17.6935317272033,17.8311684204133,6.37436110452697));
#38194=CARTESIAN_POINT('Ctrl Pts',(-17.7086373302776,17.4032043210795,6.28986592714545));
#38195=CARTESIAN_POINT('Ctrl Pts',(-17.6848569462331,17.8049443436771,6.81002864903746));
#38196=CARTESIAN_POINT('Ctrl Pts',(-17.6873896796574,17.8309547927005,6.37431892689686));
#38197=CARTESIAN_POINT('Ctrl Pts',(-17.7061493215936,17.4031095435898,6.28984721473285));
#38198=CARTESIAN_POINT('Ctrl Pts',(-17.6650316986901,17.8039394480878,6.80992416632294));
#38199=CARTESIAN_POINT('Ctrl Pts',(-17.669033565516,17.8301099792034,6.37415213097543));
#38200=CARTESIAN_POINT('Ctrl Pts',(-17.6987148534351,17.402734784112,6.28977322402055));
#38201=CARTESIAN_POINT('Ctrl Pts',(-17.65188297285,17.8029458235526,6.80982084423287));
#38202=CARTESIAN_POINT('Ctrl Pts',(-17.6568553794863,17.8292744610696,6.37398717028588));
#38203=CARTESIAN_POINT('Ctrl Pts',(-17.6937840817574,17.4023642144883,6.28970006053293));
#38204=CARTESIAN_POINT('Ctrl Pts',(-17.6126371335032,17.7990126660086,6.80941167670247));
#38205=CARTESIAN_POINT('Ctrl Pts',(-17.6204837103719,17.825965596934,6.37333388403476));
#38206=CARTESIAN_POINT('Ctrl Pts',(-17.6790668911251,17.4008973914905,6.28941045804156));
#38207=CARTESIAN_POINT('Ctrl Pts',(-17.5867398984557,17.7951231176127,6.80900689352775));
#38208=CARTESIAN_POINT('Ctrl Pts',(-17.596453210412,17.8226910680451,6.37268737676991));
#38209=CARTESIAN_POINT('Ctrl Pts',(-17.6693554286528,17.3994468177432,6.28912406372419));
#38210=CARTESIAN_POINT('Ctrl Pts',(-17.5354697949089,17.7848516081068,6.80793609188225));
#38211=CARTESIAN_POINT('Ctrl Pts',(-17.5487818608033,17.8140306147149,6.37097749843788));
#38212=CARTESIAN_POINT('Ctrl Pts',(-17.6501291396514,17.3956161693061,6.28836775888534));
#38213=CARTESIAN_POINT('Ctrl Pts',(-17.5100969352081,17.7784696191355,6.80727007507948));
#38214=CARTESIAN_POINT('Ctrl Pts',(-17.5251318472474,17.8086411999732,6.36991343826254));
#38215=CARTESIAN_POINT('Ctrl Pts',(-17.6406143159052,17.3932360814621,6.28789784576675));
#38216=CARTESIAN_POINT('Ctrl Pts',(-17.4724356982661,17.7670045961486,6.80607073498154));
#38217=CARTESIAN_POINT('Ctrl Pts',(-17.4899271035391,17.7989402787506,6.36799813494449));
#38218=CARTESIAN_POINT('Ctrl Pts',(-17.6264913542181,17.3889603296644,6.28705366185705));
#38219=CARTESIAN_POINT('Ctrl Pts',(-17.4599484159706,17.7628670210704,6.80563750504227));
#38220=CARTESIAN_POINT('Ctrl Pts',(-17.4782302202683,17.7954342534171,6.36730592213287));
#38221=CARTESIAN_POINT('Ctrl Pts',(-17.6218086213275,17.3874172771144,6.28674900896883));
#38222=CARTESIAN_POINT('Ctrl Pts',(-17.4351090516651,17.7539492007634,6.8047025599668));
#38223=CARTESIAN_POINT('Ctrl Pts',(-17.454917776984,17.7878675018479,6.36581197902636));
#38224=CARTESIAN_POINT('Ctrl Pts',(-17.6124938623285,17.384091480323,6.28609237961543));
#38225=CARTESIAN_POINT('Ctrl Pts',(-17.4227335316578,17.7491576061505,6.804199652638));
#38226=CARTESIAN_POINT('Ctrl Pts',(-17.4432789672747,17.7837963825994,6.36500819678485));
#38227=CARTESIAN_POINT('Ctrl Pts',(-17.6078530426073,17.38230451645,6.28573957004644));
#38228=CARTESIAN_POINT('Ctrl Pts',(-17.3618547466598,17.7238403969658,6.8015386718093));
#38229=CARTESIAN_POINT('Ctrl Pts',(-17.3858250678238,17.7622268875734,6.36074961922872));
#38230=CARTESIAN_POINT('Ctrl Pts',(-17.5850234902864,17.3728628177143,6.28387544637182));
#38231=CARTESIAN_POINT('Ctrl Pts',(-17.3158627238175,17.6991343295047,6.79893094285691));
#38232=CARTESIAN_POINT('Ctrl Pts',(-17.3420267744581,17.7410737731548,6.35657324986094));
#38233=CARTESIAN_POINT('Ctrl Pts',(-17.5677764852266,17.3636490384775,6.28205632202897));
#38234=CARTESIAN_POINT('Ctrl Pts',(-17.2508193911024,17.6555966201116,6.7942958684358));
#38235=CARTESIAN_POINT('Ctrl Pts',(-17.2793471455071,17.7035182827478,6.34915847411566));
#38236=CARTESIAN_POINT('Ctrl Pts',(-17.5433852397352,17.3474123674201,6.27885063163761));
#38237=CARTESIAN_POINT('Ctrl Pts',(-17.2298005184759,17.6399964301089,6.79262936990691));
#38238=CARTESIAN_POINT('Ctrl Pts',(-17.2589173832124,17.6899870750125,6.34648693741537));
#38239=CARTESIAN_POINT('Ctrl Pts',(-17.5355031559793,17.3415945569023,6.27770199105668));
#38240=CARTESIAN_POINT('Ctrl Pts',(-17.204378613571,17.619097401045,6.79038682430432));
#38241=CARTESIAN_POINT('Ctrl Pts',(-17.2340263963876,17.6717874399427,6.34289368883238));
#38242=CARTESIAN_POINT('Ctrl Pts',(-17.5259699480092,17.3338006396197,6.27616319744218));
#38243=CARTESIAN_POINT('Ctrl Pts',(-17.1993309492766,17.6148421450605,6.78992974985876));
#38244=CARTESIAN_POINT('Ctrl Pts',(-17.2290682897225,17.6680734413416,6.34216041477718));
#38245=CARTESIAN_POINT('Ctrl Pts',(-17.5240770741103,17.3322137206402,6.27584988377669));
#38246=CARTESIAN_POINT('Ctrl Pts',(-17.1893716918988,17.6062334486389,6.78900404892269));
#38247=CARTESIAN_POINT('Ctrl Pts',(-17.2192636543449,17.6605500551435,6.34067503352136));
#38248=CARTESIAN_POINT('Ctrl Pts',(-17.5203423496229,17.3290032721058,6.27521602822943));
#38249=CARTESIAN_POINT('Ctrl Pts',(-17.1844557566987,17.6018767026284,6.78853506940883));
#38250=CARTESIAN_POINT('Ctrl Pts',(-17.2144128912708,17.6567376554324,6.33992233162338));
#38251=CARTESIAN_POINT('Ctrl Pts',(-17.5184988766973,17.3273785031339,6.27489524164313));
#38252=CARTESIAN_POINT('Ctrl Pts',(-17.169896855944,17.5886510409319,6.78710983089398));
#38253=CARTESIAN_POINT('Ctrl Pts',(-17.2000081285538,17.6451450983018,6.33763355279219));
#38254=CARTESIAN_POINT('Ctrl Pts',(-17.5130392850471,17.3224462500153,6.27392144126411));
#38255=CARTESIAN_POINT('Ctrl Pts',(-17.1604426857215,17.5796268087842,6.78613528430944));
#38256=CARTESIAN_POINT('Ctrl Pts',(-17.1906117770433,17.6372170607117,6.33606827910802));
#38257=CARTESIAN_POINT('Ctrl Pts',(-17.5094939755331,17.3190808343234,6.27325698974518));
#38258=CARTESIAN_POINT('Ctrl Pts',(-17.1144092624932,17.5334875838914,6.78114111890133));
#38259=CARTESIAN_POINT('Ctrl Pts',(-17.1445255959529,17.5964801911601,6.32802538713625));
#38260=CARTESIAN_POINT('Ctrl Pts',(-17.4922314331161,17.3018741366695,6.26985978195909));
#38261=CARTESIAN_POINT('Ctrl Pts',(-17.0815070486393,17.4933474524288,6.77676052830464));
#38262=CARTESIAN_POINT('Ctrl Pts',(-17.1109009441881,17.5607248183131,6.32096601796079));
#38263=CARTESIAN_POINT('Ctrl Pts',(-17.4798931004167,17.2869047271829,6.26690429360894));
#38264=CARTESIAN_POINT('Ctrl Pts',(-17.0453050933139,17.4391198002594,6.77077798629523));
#38265=CARTESIAN_POINT('Ctrl Pts',(-17.0729618602987,17.5119192000139,6.31133007096938));
#38266=CARTESIAN_POINT('Ctrl Pts',(-17.4663173790063,17.2666817095338,6.26291155808251));
#38267=CARTESIAN_POINT('Ctrl Pts',(-17.0383132060228,17.4280698300166,6.76955593094628));
#38268=CARTESIAN_POINT('Ctrl Pts',(-17.065556626733,17.5019159878677,6.30935508478244));
#38269=CARTESIAN_POINT('Ctrl Pts',(-17.4636954152817,17.2625608716606,6.2620979596344));
#38270=CARTESIAN_POINT('Ctrl Pts',(-17.0248360913008,17.4055530530904,6.76705920363801));
#38271=CARTESIAN_POINT('Ctrl Pts',(-17.0511605700457,17.4814635711966,6.30531705781432));
#38272=CARTESIAN_POINT('Ctrl Pts',(-17.4586415045071,17.2541637364834,6.26044006957447));
#38273=CARTESIAN_POINT('Ctrl Pts',(-17.018385745669,17.3941425328792,6.76579076471037));
#38274=CARTESIAN_POINT('Ctrl Pts',(-17.044207273457,17.4710642956499,6.30326387477087));
#38275=CARTESIAN_POINT('Ctrl Pts',(-17.4562226243632,17.2499084384684,6.25959992396146));
#38276=CARTESIAN_POINT('Ctrl Pts',(-16.9999748915757,17.3596229038005,6.76194338591157));
#38277=CARTESIAN_POINT('Ctrl Pts',(-17.0241507155953,17.4394666729185,6.29702539181943));
#38278=CARTESIAN_POINT('Ctrl Pts',(-17.449318544805,17.237035119937,6.25705827774745));
#38279=CARTESIAN_POINT('Ctrl Pts',(-16.9889119861745,17.3361594967524,6.75931504519851));
#38280=CARTESIAN_POINT('Ctrl Pts',(-17.0118468913603,17.4178612762011,6.29275972600569));
#38281=CARTESIAN_POINT('Ctrl Pts',(-17.4451699630122,17.2282849645212,6.25533068906623));
#38282=CARTESIAN_POINT('Ctrl Pts',(-16.969151536231,17.2883531218114,6.75393133468145));
#38283=CARTESIAN_POINT('Ctrl Pts',(-16.9893185039968,17.3735255531602,6.28400629367688));
#38284=CARTESIAN_POINT('Ctrl Pts',(-17.4377597911824,17.2104566385494,6.25181074996914));
#38285=CARTESIAN_POINT('Ctrl Pts',(-16.9604540998271,17.2640101175317,6.75117596780138));
#38286=CARTESIAN_POINT('Ctrl Pts',(-16.979100694343,17.3507885344851,6.27951720585606));
#38287=CARTESIAN_POINT('Ctrl Pts',(-17.4344982506951,17.2013784496697,6.25001839593549));
#38288=CARTESIAN_POINT('Ctrl Pts',(-16.9454368141968,17.2144400485736,6.74553518479638));
#38289=CARTESIAN_POINT('Ctrl Pts',(-16.9607944578447,17.3041453864073,6.27030820660447));
#38290=CARTESIAN_POINT('Ctrl Pts',(-17.4288667753564,17.1828923505283,6.24636858926135));
#38291=CARTESIAN_POINT('Ctrl Pts',(-16.9391152612491,17.1892056047591,6.74264892813991));
#38292=CARTESIAN_POINT('Ctrl Pts',(-16.9527111071462,17.2802251876746,6.26558551739275));
#38293=CARTESIAN_POINT('Ctrl Pts',(-17.4264961901478,17.173481691707,6.24451059395842));
#38294=CARTESIAN_POINT('Ctrl Pts',(-16.9340264307573,17.163528852123,6.73969634090002));
#38295=CARTESIAN_POINT('Ctrl Pts',(-16.9457712867961,17.2557485214382,6.26075296190838));
#38296=CARTESIAN_POINT('Ctrl Pts',(-17.4245878781802,17.16390605946,6.24262002709426));
#38297=CARTESIAN_POINT('',(-18.0133068931633,17.0493818775139,6.22000892237058));
#38298=CARTESIAN_POINT('Origin',(-18.0133034595933,16.9525344893951,6.71053984230837));
#38299=CARTESIAN_POINT('',(-17.424587878778,17.1639060593454,6.24262002707162));
#38300=CARTESIAN_POINT('Ctrl Pts',(-17.4245878781802,17.16390605946,6.24262002709426));
#38301=CARTESIAN_POINT('Ctrl Pts',(-17.4239963526266,17.1609378701589,6.24203400204708));
#38302=CARTESIAN_POINT('Ctrl Pts',(-17.423450686133,17.1579624057897,6.24144654064541));
#38303=CARTESIAN_POINT('Ctrl Pts',(-17.4229521590767,17.1549871578456,6.24085912197364));
#38304=CARTESIAN_POINT('Ctrl Pts',(-17.4217671914954,17.1479151798734,6.23946286459101));
#38305=CARTESIAN_POINT('Ctrl Pts',(-17.4208459359997,17.140831572302,6.23806431111613));
#38306=CARTESIAN_POINT('Ctrl Pts',(-17.4201854095159,17.1337362792114,6.23666345050844));
#38307=CARTESIAN_POINT('Ctrl Pts',(-17.4193357250156,17.1246090743057,6.23486141898593));
#38308=CARTESIAN_POINT('Ctrl Pts',(-17.418917461125,17.115461497848,6.23305536540196));
#38309=CARTESIAN_POINT('Ctrl Pts',(-17.4189248391062,17.1062963840515,6.23124584933002));
#38310=CARTESIAN_POINT('Ctrl Pts',(-17.4189325800007,17.0966804501252,6.22934732549576));
#38311=CARTESIAN_POINT('Ctrl Pts',(-17.4194120469241,17.0870438617571,6.22744472374767));
#38312=CARTESIAN_POINT('Ctrl Pts',(-17.4203763301195,17.0773875052259,6.22553821906834));
#38313=CARTESIAN_POINT('Ctrl Pts',(-17.4204307036815,17.0768430069889,6.22543071595024));
#38314=CARTESIAN_POINT('Ctrl Pts',(-17.4204866297116,17.0762983905452,6.22532318949395));
#38315=CARTESIAN_POINT('Ctrl Pts',(-17.42054410957,17.0757536753193,6.22521564353459));
#38316=CARTESIAN_POINT('Ctrl Pts',(-17.4209972115288,17.0714597966854,6.22436788074937));
#38317=CARTESIAN_POINT('Ctrl Pts',(-17.4215449020002,17.0671774008785,6.2235223850784));
#38318=CARTESIAN_POINT('Ctrl Pts',(-17.4221870883531,17.0629071178979,6.22267928090569));
#38319=CARTESIAN_POINT('Ctrl Pts',(-17.4222707183068,17.0623510120782,6.22256948604217));
#38320=CARTESIAN_POINT('Ctrl Pts',(-17.4223558880511,17.0617955245123,6.2224598132437));
#38321=CARTESIAN_POINT('Ctrl Pts',(-17.4224425947226,17.0612406342997,6.22235025838381));
#38322=CARTESIAN_POINT('Ctrl Pts',(-17.42310851407,17.0569789999625,6.22150886175776));
#38323=CARTESIAN_POINT('Ctrl Pts',(-17.4238662074175,17.0527464735124,6.2206732120532));
#38324=CARTESIAN_POINT('Ctrl Pts',(-17.4247139972883,17.0485425419806,6.21984320799205));
#38325=CARTESIAN_POINT('Ctrl Pts',(-17.4248242481398,17.0479958416164,6.2197352700965));
#38326=CARTESIAN_POINT('Ctrl Pts',(-17.4249360094247,17.0474496203497,6.21962742679168));
#38327=CARTESIAN_POINT('Ctrl Pts',(-17.4250492807261,17.0469038779886,6.21951967803966));
#38328=CARTESIAN_POINT('Ctrl Pts',(-17.4270178554423,17.0374192636091,6.21764708130632));
#38329=CARTESIAN_POINT('Ctrl Pts',(-17.4294421208925,17.0280792618812,6.21580303620074));
#38330=CARTESIAN_POINT('Ctrl Pts',(-17.4323202517924,17.0188829947148,6.21398736935701));
#38331=CARTESIAN_POINT('Ctrl Pts',(-17.4350337261126,17.0102128418741,6.21227557600019));
#38332=CARTESIAN_POINT('Ctrl Pts',(-17.4381502171147,17.0016706838313,6.21058905332191));
#38333=CARTESIAN_POINT('Ctrl Pts',(-17.4416688286559,16.9932560204131,6.20892770257016));
#38334=CARTESIAN_POINT('Ctrl Pts',(-17.4418823418398,16.992745409464,6.2088268899955));
#38335=CARTESIAN_POINT('Ctrl Pts',(-17.4420973488182,16.9922352722248,6.20872617094784));
#38336=CARTESIAN_POINT('Ctrl Pts',(-17.4423138525004,16.9917256096056,6.20862554560688));
#38337=CARTESIAN_POINT('Ctrl Pts',(-17.4439898422823,16.9877802294007,6.20784658867852));
#38338=CARTESIAN_POINT('Ctrl Pts',(-17.4457556853019,16.9838624646562,6.20707308401416));
#38339=CARTESIAN_POINT('Ctrl Pts',(-17.4476116630671,16.9799749316384,6.20630554815676));
#38340=CARTESIAN_POINT('Ctrl Pts',(-17.4478510911231,16.9794734253754,6.20620653316761));
#38341=CARTESIAN_POINT('Ctrl Pts',(-17.4480920630631,16.9789723398839,6.20610760125357));
#38342=CARTESIAN_POINT('Ctrl Pts',(-17.4483345640874,16.978471710916,6.20600875947336));
#38343=CARTESIAN_POINT('Ctrl Pts',(-17.4502147381132,16.974590203261,6.20524241323467));
#38344=CARTESIAN_POINT('Ctrl Pts',(-17.4521887529142,16.9707323959116,6.20448074627054));
#38345=CARTESIAN_POINT('Ctrl Pts',(-17.4542495612884,16.9669156327685,6.20372718287749));
#38346=CARTESIAN_POINT('Ctrl Pts',(-17.4545149485985,16.966424116664,6.20363014029728));
#38347=CARTESIAN_POINT('Ctrl Pts',(-17.4547816091611,16.9659335710049,6.20353328931717));
#38348=CARTESIAN_POINT('Ctrl Pts',(-17.4550495371491,16.9654439997817,6.20343663072499));
#38349=CARTESIAN_POINT('Ctrl Pts',(-17.4594793107355,16.9573496991847,6.20183853087085));
#38350=CARTESIAN_POINT('Ctrl Pts',(-17.4642582686348,16.9495167468061,6.20029203035437));
#38351=CARTESIAN_POINT('Ctrl Pts',(-17.4693759748133,16.9419372968202,6.19879558013341));
#38352=CARTESIAN_POINT('Ctrl Pts',(-17.4751109733341,16.9334436215403,6.19711862965902));
#38353=CARTESIAN_POINT('Ctrl Pts',(-17.4812683755285,16.9252660518675,6.19550408955828));
#38354=CARTESIAN_POINT('Ctrl Pts',(-17.4878532971521,16.9174083701159,6.1939527065931));
#38355=CARTESIAN_POINT('Ctrl Pts',(-17.4937314913045,16.9103940149625,6.19256782598321));
#38356=CARTESIAN_POINT('Ctrl Pts',(-17.4999501245273,16.9036348244842,6.19123332386186));
#38357=CARTESIAN_POINT('Ctrl Pts',(-17.5065131208216,16.8971331521054,6.1899496648779));
#38358=CARTESIAN_POINT('Ctrl Pts',(-17.5069065081345,16.8967434405603,6.1898727221012));
#38359=CARTESIAN_POINT('Ctrl Pts',(-17.5073011442382,16.8963546628821,6.18979596370271));
#38360=CARTESIAN_POINT('Ctrl Pts',(-17.5076970324673,16.8959668214413,6.18971939015042));
#38361=CARTESIAN_POINT('Ctrl Pts',(-17.5090515851221,16.8946398013009,6.18945738966409));
#38362=CARTESIAN_POINT('Ctrl Pts',(-17.5104207888425,16.8933237461276,6.18919755404825));
#38363=CARTESIAN_POINT('Ctrl Pts',(-17.5118047748885,16.8920187547148,6.18893990280817));
#38364=CARTESIAN_POINT('Ctrl Pts',(-17.5135932512801,16.8903323603036,6.18860694919096));
#38365=CARTESIAN_POINT('Ctrl Pts',(-17.5154090302819,16.8886621211746,6.18827718519512));
#38366=CARTESIAN_POINT('Ctrl Pts',(-17.5172419503642,16.8870175731272,6.1879524935231));
#38367=CARTESIAN_POINT('Ctrl Pts',(-17.5176558878116,16.8866461766722,6.18787916678986));
#38368=CARTESIAN_POINT('Ctrl Pts',(-17.5180706956164,16.8862760853643,6.18780609773861));
#38369=CARTESIAN_POINT('Ctrl Pts',(-17.5184863718957,16.8859072963858,6.18773328581301));
#38370=CARTESIAN_POINT('Ctrl Pts',(-17.5217519345969,16.8830100814304,6.18716127359994));
#38371=CARTESIAN_POINT('Ctrl Pts',(-17.5250710692817,16.8801931952623,6.18660512111705));
#38372=CARTESIAN_POINT('Ctrl Pts',(-17.5284428907987,16.8774553207796,6.18606456832203));
#38373=CARTESIAN_POINT('Ctrl Pts',(-17.5288714663989,16.8771073230598,6.18599586132275));
#38374=CARTESIAN_POINT('Ctrl Pts',(-17.5293008917546,16.8767605997055,6.18592740592809));
#38375=CARTESIAN_POINT('Ctrl Pts',(-17.5297311661369,16.876415149672,6.18585920193176));
#38376=CARTESIAN_POINT('Ctrl Pts',(-17.5369330750402,16.870633026045,6.18471760719924));
#38377=CARTESIAN_POINT('Ctrl Pts',(-17.5443727527964,16.8652074307487,6.18364640370889));
#38378=CARTESIAN_POINT('Ctrl Pts',(-17.5520464878964,16.8601328033148,6.18264449362848));
#38379=CARTESIAN_POINT('Ctrl Pts',(-17.5601786799816,16.8547549990883,6.18158272577751));
#38380=CARTESIAN_POINT('Ctrl Pts',(-17.5685737386504,16.8497713618965,6.18059878037371));
#38381=CARTESIAN_POINT('Ctrl Pts',(-17.5772348972466,16.8451867599133,6.17969361856599));
#38382=CARTESIAN_POINT('Ctrl Pts',(-17.5777203263771,16.8449298082215,6.17964288725742));
#38383=CARTESIAN_POINT('Ctrl Pts',(-17.5782065927925,16.8446741120996,6.17959240384255));
#38384=CARTESIAN_POINT('Ctrl Pts',(-17.5786936981234,16.8444196739979,6.17954216880515));
#38385=CARTESIAN_POINT('Ctrl Pts',(-17.582552127317,16.8424042343437,6.17914425007471));
#38386=CARTESIAN_POINT('Ctrl Pts',(-17.586463186836,16.8404677179035,6.17876191356478));
#38387=CARTESIAN_POINT('Ctrl Pts',(-17.5904276953827,16.8386113479185,6.17839540078621));
#38388=CARTESIAN_POINT('Ctrl Pts',(-17.5909274567178,16.8383773360778,6.17834919861174));
#38389=CARTESIAN_POINT('Ctrl Pts',(-17.5914280675634,16.8381445980764,6.17830324793798));
#38390=CARTESIAN_POINT('Ctrl Pts',(-17.5919295301886,16.8379131373121,6.17825754943576));
#38391=CARTESIAN_POINT('Ctrl Pts',(-17.5936681678983,16.8371106320145,6.17809910664215));
#38392=CARTESIAN_POINT('Ctrl Pts',(-17.5954170352532,16.8363234502043,6.17794368924433));
#38393=CARTESIAN_POINT('Ctrl Pts',(-17.5971762338363,16.8355517601033,6.1777913304552));
#38394=CARTESIAN_POINT('Ctrl Pts',(-17.5994428292503,16.8345574952939,6.17759502758407));
#38395=CARTESIAN_POINT('Ctrl Pts',(-17.6017284628056,16.8335882506517,6.17740366457469));
#38396=CARTESIAN_POINT('Ctrl Pts',(-17.6040187012687,16.8326501826568,6.17721845693285));
#38397=CARTESIAN_POINT('Ctrl Pts',(-17.6045306328368,16.8324404985443,6.17717705790824));
#38398=CARTESIAN_POINT('Ctrl Pts',(-17.6050429326839,16.8322322929262,6.17713595079046));
#38399=CARTESIAN_POINT('Ctrl Pts',(-17.6055556005716,16.8320255651881,6.17709513545823));
#38400=CARTESIAN_POINT('Ctrl Pts',(-17.6147282126709,16.8283268093328,6.17636487085756));
#38401=CARTESIAN_POINT('Ctrl Pts',(-17.6240182691166,16.8250999643395,6.17572777807219));
#38402=CARTESIAN_POINT('Ctrl Pts',(-17.6334245013524,16.8223376299444,6.17518239602947));
#38403=CARTESIAN_POINT('Ctrl Pts',(-17.6423072352983,16.8197290316356,6.17466736690166));
#38404=CARTESIAN_POINT('Ctrl Pts',(-17.6512948852706,16.8175343889948,6.17423406719378));
#38405=CARTESIAN_POINT('Ctrl Pts',(-17.6603835260784,16.815748176766,6.17388140602583));
#38406=CARTESIAN_POINT('Ctrl Pts',(-17.6700101964278,16.8138562243097,6.17350786801496));
#38407=CARTESIAN_POINT('Ctrl Pts',(-17.6797510047685,16.8124258453062,6.17322546085085));
#38408=CARTESIAN_POINT('Ctrl Pts',(-17.6896061275879,16.8114698645862,6.17303671660658));
#38409=CARTESIAN_POINT('Ctrl Pts',(-17.6901520189626,16.8114169112502,6.17302626175413));
#38410=CARTESIAN_POINT('Ctrl Pts',(-17.6906984201744,16.8113654130281,6.17301609419237));
#38411=CARTESIAN_POINT('Ctrl Pts',(-17.691245246391,16.81131537637,6.17300621519479));
#38412=CARTESIAN_POINT('Ctrl Pts',(-17.6956341166443,16.8109137782137,6.17292692558263));
#38413=CARTESIAN_POINT('Ctrl Pts',(-17.7000547883742,16.8106061648172,6.17286619187026));
#38414=CARTESIAN_POINT('Ctrl Pts',(-17.704458698247,16.8103961220267,6.17282472203));
#38415=CARTESIAN_POINT('Ctrl Pts',(-17.7050064698865,16.8103699962687,6.17281956388575));
#38416=CARTESIAN_POINT('Ctrl Pts',(-17.7055540701931,16.8103453624145,6.17281470029583));
#38417=CARTESIAN_POINT('Ctrl Pts',(-17.7061014900395,16.8103222168314,6.17281013054302));
#38418=CARTESIAN_POINT('Ctrl Pts',(-17.7105033630717,16.8101361002363,6.17277338457593));
#38419=CARTESIAN_POINT('Ctrl Pts',(-17.7148955099544,16.8100464048699,6.17275567555338));
#38420=CARTESIAN_POINT('Ctrl Pts',(-17.7192780851963,16.8100515461297,6.17275669061902));
#38421=CARTESIAN_POINT('Ctrl Pts',(-17.7198223171621,16.8100521845758,6.17275681667074));
#38422=CARTESIAN_POINT('Ctrl Pts',(-17.7203664028382,16.8100542724886,6.17275722889823));
#38423=CARTESIAN_POINT('Ctrl Pts',(-17.7209103422184,16.8100578098489,6.17275792729767));
#38424=CARTESIAN_POINT('Ctrl Pts',(-17.7307586592126,16.810121855673,6.17277057219769));
#38425=CARTESIAN_POINT('Ctrl Pts',(-17.740559079287,16.8106606220985,6.17287694365447));
#38426=CARTESIAN_POINT('Ctrl Pts',(-17.7503117673952,16.8116743046869,6.17307708027865));
#38427=CARTESIAN_POINT('Ctrl Pts',(-17.7595290142826,16.8126323341633,6.17326622901958));
#38428=CARTESIAN_POINT('Ctrl Pts',(-17.7687032606477,16.8140145017524,6.17353911755344));
#38429=CARTESIAN_POINT('Ctrl Pts',(-17.7778348290988,16.8158209130995,6.17389576673834));
#38430=CARTESIAN_POINT('Ctrl Pts',(-17.7783652931537,16.8159258497589,6.17391648492863));
#38431=CARTESIAN_POINT('Ctrl Pts',(-17.7788956118845,16.8160322309445,6.17393748831926));
#38432=CARTESIAN_POINT('Ctrl Pts',(-17.7794257850525,16.8161400596518,6.1739587775016));
#38433=CARTESIAN_POINT('Ctrl Pts',(-17.7837247873403,16.8170144076703,6.17413140457718));
#38434=CARTESIAN_POINT('Ctrl Pts',(-17.7880141653873,16.8179839070022,6.17432281787131));
#38435=CARTESIAN_POINT('Ctrl Pts',(-17.7922938185966,16.8190500973935,6.17453332138404));
#38436=CARTESIAN_POINT('Ctrl Pts',(-17.7928208008302,16.819181384525,6.17455924208506));
#38437=CARTESIAN_POINT('Ctrl Pts',(-17.793347671119,16.8193141584276,6.17458545632702));
#38438=CARTESIAN_POINT('Ctrl Pts',(-17.7938743549672,16.8194483975145,6.17461195984794));
#38439=CARTESIAN_POINT('Ctrl Pts',(-17.7981523653082,16.8205387597953,6.17482723574251));
#38440=CARTESIAN_POINT('Ctrl Pts',(-17.8024180418494,16.8217260125767,6.17506164123241));
#38441=CARTESIAN_POINT('Ctrl Pts',(-17.8066313677461,16.822998390726,6.17531285346629));
#38442=CARTESIAN_POINT('Ctrl Pts',(-17.8071493194822,16.8231548064621,6.17534373543837));
#38443=CARTESIAN_POINT('Ctrl Pts',(-17.8076666436156,16.8233125431413,6.17537487821111));
#38444=CARTESIAN_POINT('Ctrl Pts',(-17.8081833410617,16.8234715983733,6.17540628131259));
#38445=CARTESIAN_POINT('Ctrl Pts',(-17.8171078324416,16.8262188289972,6.17594868133921));
#38446=CARTESIAN_POINT('Ctrl Pts',(-17.8258454839216,16.829359850349,6.17656882951683));
#38447=CARTESIAN_POINT('Ctrl Pts',(-17.8344010756028,16.8328846040527,6.17726473996791));
#38448=CARTESIAN_POINT('Ctrl Pts',(-17.8439443772991,16.8368162769577,6.17804099059274));
#38449=CARTESIAN_POINT('Ctrl Pts',(-17.8532627983433,16.8412219375003,6.17891082306143));
#38450=CARTESIAN_POINT('Ctrl Pts',(-17.8623523860865,16.8461099313546,6.17987588510378));
#38451=CARTESIAN_POINT('Ctrl Pts',(-17.8705041290683,16.8504935921676,6.18074137405146));
#38452=CARTESIAN_POINT('Ctrl Pts',(-17.8784700287685,16.8552640274904,6.18168322590168));
#38453=CARTESIAN_POINT('Ctrl Pts',(-17.8862519595826,16.8604302491132,6.18270321989906));
#38454=CARTESIAN_POINT('Ctrl Pts',(-17.8866982213105,16.8607265106765,6.18276171235995));
#38455=CARTESIAN_POINT('Ctrl Pts',(-17.8871438840282,16.8610241014696,6.1828204672576));
#38456=CARTESIAN_POINT('Ctrl Pts',(-17.8875888292958,16.8613229394795,6.18287946839972));
#38457=CARTESIAN_POINT('Ctrl Pts',(-17.8891949126272,16.8624016311327,6.18309244010161));
#38458=CARTESIAN_POINT('Ctrl Pts',(-17.8907913791061,16.8634963971031,6.18330858543951));
#38459=CARTESIAN_POINT('Ctrl Pts',(-17.8923726652077,16.8646033654539,6.18352713995682));
#38460=CARTESIAN_POINT('Ctrl Pts',(-17.8943923022893,16.8660171983633,6.18380628033951));
#38461=CARTESIAN_POINT('Ctrl Pts',(-17.8963900764334,16.867452833543,6.1840897252578));
#38462=CARTESIAN_POINT('Ctrl Pts',(-17.8983663167529,16.8689100738024,6.18437743577929));
#38463=CARTESIAN_POINT('Ctrl Pts',(-17.9023190460032,16.8718247376421,6.18495289301631));
#38464=CARTESIAN_POINT('Ctrl Pts',(-17.9061856528232,16.874825808707,6.1855454100811));
#38465=CARTESIAN_POINT('Ctrl Pts',(-17.9099681280811,16.8779123579719,6.18615480355134));
#38466=CARTESIAN_POINT('Ctrl Pts',(-17.9103771355834,16.8782461134415,6.18622069862909));
#38467=CARTESIAN_POINT('Ctrl Pts',(-17.9107851609273,16.8785808668023,6.1862867907257));
#38468=CARTESIAN_POINT('Ctrl Pts',(-17.9111922053572,16.8789166181642,6.18635307986288));
#38469=CARTESIAN_POINT('Ctrl Pts',(-17.9183132823679,16.8847904519018,6.18751278139937));
#38470=CARTESIAN_POINT('Ctrl Pts',(-17.9251329124577,16.8909686819571,6.18873258148364));
#38471=CARTESIAN_POINT('Ctrl Pts',(-17.9316538269046,16.8974481022438,6.19001184712136));
#38472=CARTESIAN_POINT('Ctrl Pts',(-17.9385476266958,16.9042980351151,6.19136426498516));
#38473=CARTESIAN_POINT('Ctrl Pts',(-17.9451075853853,16.9114845746872,6.19278314086014));
#38474=CARTESIAN_POINT('Ctrl Pts',(-17.9513273259246,16.9190136164559,6.19426963872467));
#38475=CARTESIAN_POINT('Ctrl Pts',(-17.9516615723884,16.9194182242641,6.19434952254805));
#38476=CARTESIAN_POINT('Ctrl Pts',(-17.9519948445867,16.919823836157,6.19442960461311));
#38477=CARTESIAN_POINT('Ctrl Pts',(-17.9523271371351,16.9202304499703,6.1945098844925));
#38478=CARTESIAN_POINT('Ctrl Pts',(-17.9550864843114,16.9236069586604,6.19517652615973));
#38479=CARTESIAN_POINT('Ctrl Pts',(-17.9577784017783,16.9270526915071,6.19585683511218));
#38480=CARTESIAN_POINT('Ctrl Pts',(-17.9604002187094,16.9305669206281,6.19655066764019));
#38481=CARTESIAN_POINT('Ctrl Pts',(-17.9607154832163,16.9309894946446,6.19663409862548));
#38482=CARTESIAN_POINT('Ctrl Pts',(-17.9610294892565,16.9314127309544,6.19671766037079));
#38483=CARTESIAN_POINT('Ctrl Pts',(-17.9613422375567,16.931836625018,6.19680135197987));
#38484=CARTESIAN_POINT('Ctrl Pts',(-17.963943627082,16.9353625069371,6.19749748518041));
#38485=CARTESIAN_POINT('Ctrl Pts',(-17.9664564881878,16.938932118167,6.19820225208616));
#38486=CARTESIAN_POINT('Ctrl Pts',(-17.9688822689746,16.9425440504763,6.19891537466263));
#38487=CARTESIAN_POINT('Ctrl Pts',(-17.9691734405987,16.9429775983889,6.19900097228131));
#38488=CARTESIAN_POINT('Ctrl Pts',(-17.9694633772217,16.9434117629754,6.1990866916531));
#38489=CARTESIAN_POINT('Ctrl Pts',(-17.9697520814202,16.9438465470988,6.19917253334329));
#38490=CARTESIAN_POINT('Ctrl Pts',(-17.9751399386372,16.9519605779618,6.2007745286464));
#38491=CARTESIAN_POINT('Ctrl Pts',(-17.9800962739498,16.9602865087157,6.20241836044683));
#38492=CARTESIAN_POINT('Ctrl Pts',(-17.9846245725303,16.9688229597914,6.204103756369));
#38493=CARTESIAN_POINT('Ctrl Pts',(-17.9889117260424,16.976904820022,6.20569940005691));
#38494=CARTESIAN_POINT('Ctrl Pts',(-17.9928153343569,16.9851749215112,6.20733220919538));
#38495=CARTESIAN_POINT('Ctrl Pts',(-17.9963377138694,16.9936323565903,6.20900200457843));
#38496=CARTESIAN_POINT('Ctrl Pts',(-17.9965358417055,16.9941080728797,6.20909592771898));
#38497=CARTESIAN_POINT('Ctrl Pts',(-17.9967327525697,16.9945843870955,6.20918996891125));
#38498=CARTESIAN_POINT('Ctrl Pts',(-17.996928444502,16.9950613002111,6.20928412834743));
#38499=CARTESIAN_POINT('Ctrl Pts',(-17.9985704225849,16.9990629004521,6.21007418508978));
#38500=CARTESIAN_POINT('Ctrl Pts',(-18.000127055299,17.003107344624,6.21087270073222));
#38501=CARTESIAN_POINT('Ctrl Pts',(-18.0015963946161,17.0071929605557,6.21167934512926));
#38502=CARTESIAN_POINT('Ctrl Pts',(-18.0017712541485,17.0076791715238,6.2117753402888));
#38503=CARTESIAN_POINT('Ctrl Pts',(-18.0019449012453,17.0081660427692,6.21187146581032));
#38504=CARTESIAN_POINT('Ctrl Pts',(-18.0021173239188,17.0086535449126,6.21196771589332));
#38505=CARTESIAN_POINT('Ctrl Pts',(-18.00356647107,17.0127508154623,6.2127766613222));
#38506=CARTESIAN_POINT('Ctrl Pts',(-18.004930376233,17.0168964776297,6.21359516095978));
#38507=CARTESIAN_POINT('Ctrl Pts',(-18.0062015761076,17.0210725713349,6.21441966885408));
#38508=CARTESIAN_POINT('Ctrl Pts',(-18.0063525764999,17.0215686316325,6.21451760861796));
#38509=CARTESIAN_POINT('Ctrl Pts',(-18.0065022211477,17.0220649394007,6.21461559724126));
#38510=CARTESIAN_POINT('Ctrl Pts',(-18.0066505099709,17.0225614895283,6.21471363371481));
#38511=CARTESIAN_POINT('Ctrl Pts',(-18.0092960000388,17.0314200022727,6.21646261594682));
#38512=CARTESIAN_POINT('Ctrl Pts',(-18.011514751731,17.0403601479657,6.21822771540715));
#38513=CARTESIAN_POINT('Ctrl Pts',(-18.0133068931633,17.0493818775115,6.22000892238259));
#38514=CARTESIAN_POINT('Origin',(-17.4245878781802,17.0670580149496,6.73315081743725));
#38515=CARTESIAN_POINT('Ctrl Pts',(-36.918942728626,17.5305480494939,-3.00047863991406));
#38516=CARTESIAN_POINT('Ctrl Pts',(-36.9184636408495,17.5305448701384,-2.5));
#38517=CARTESIAN_POINT('Ctrl Pts',(-37.418931489881,17.5338661095488,-2.5));
#38518=CARTESIAN_POINT('Ctrl Pts',(-36.918766523927,17.5567617326884,-2.99813492793641));
#38519=CARTESIAN_POINT('Ctrl Pts',(-36.9206303865991,17.5567282897711,-2.5));
#38520=CARTESIAN_POINT('Ctrl Pts',(-37.4188654127938,17.5438230235078,-2.5));
#38521=CARTESIAN_POINT('Ctrl Pts',(-36.9198840261816,17.5827769733229,-2.99578898700793));
#38522=CARTESIAN_POINT('Ctrl Pts',(-36.9240615386413,17.5825477668969,-2.5));
#38523=CARTESIAN_POINT('Ctrl Pts',(-37.4192844801969,17.5537061882809,-2.5));
#38524=CARTESIAN_POINT('Ctrl Pts',(-36.9246169309371,17.6343825999131,-2.99109602673912));
#38525=CARTESIAN_POINT('Ctrl Pts',(-36.9333093941054,17.6333273268776,-2.5));
#38526=CARTESIAN_POINT('Ctrl Pts',(-37.4210593120151,17.5733143538484,-2.5));
#38527=CARTESIAN_POINT('Ctrl Pts',(-36.9282325359345,17.6599800335755,-2.98874837352374));
#38528=CARTESIAN_POINT('Ctrl Pts',(-36.9391161778231,17.6582989890867,-2.5));
#38529=CARTESIAN_POINT('Ctrl Pts',(-37.4224151662337,17.5830420307807,-2.5));
#38530=CARTESIAN_POINT('Ctrl Pts',(-36.9379460863992,17.710766834452,-2.98405135826386));
#38531=CARTESIAN_POINT('Ctrl Pts',(-36.9530417639778,17.7074272412772,-2.5));
#38532=CARTESIAN_POINT('Ctrl Pts',(-37.4260577504339,17.6023455517275,-2.5));
#38533=CARTESIAN_POINT('Ctrl Pts',(-36.9440439356691,17.7359562130125,-2.98170199150478));
#38534=CARTESIAN_POINT('Ctrl Pts',(-36.961150208635,17.7315882072703,-2.5));
#38535=CARTESIAN_POINT('Ctrl Pts',(-37.4283444361295,17.6119214029654,-2.5));
#38536=CARTESIAN_POINT('Ctrl Pts',(-36.9550940181883,17.7734276473997,-2.97817796458518));
#38537=CARTESIAN_POINT('Ctrl Pts',(-36.9750602300798,17.7672721065816,-2.5));
#38538=CARTESIAN_POINT('Ctrl Pts',(-37.4324882266632,17.6261687598122,-2.5));
#38539=CARTESIAN_POINT('Ctrl Pts',(-36.9590977423692,17.7858733013829,-2.97700260220075));
#38540=CARTESIAN_POINT('Ctrl Pts',(-36.9799820522302,17.7790613692586,-2.5));
#38541=CARTESIAN_POINT('Ctrl Pts',(-37.4339896230655,17.6309012462933,-2.5));
#38542=CARTESIAN_POINT('Ctrl Pts',(-36.9677444087214,17.8106277669609,-2.97465510692309));
#38543=CARTESIAN_POINT('Ctrl Pts',(-36.9903966889781,17.8024136686443,-2.5));
#38544=CARTESIAN_POINT('Ctrl Pts',(-37.437232116886,17.6403150006157,-2.5));
#38545=CARTESIAN_POINT('Ctrl Pts',(-36.9723569013568,17.8228504435788,-2.97349114599914));
#38546=CARTESIAN_POINT('Ctrl Pts',(-36.9958519245572,17.8138964486576,-2.5));
#38547=CARTESIAN_POINT('Ctrl Pts',(-37.4389618074377,17.6449635078328,-2.5));
#38548=CARTESIAN_POINT('Ctrl Pts',(-36.9968316404772,17.8831937506765,-2.96772154502321));
#38549=CARTESIAN_POINT('Ctrl Pts',(-37.0242345246282,17.8701746208594,-2.5));
#38550=CARTESIAN_POINT('Ctrl Pts',(-37.4481398206947,17.6679151360551,-2.5));
#38551=CARTESIAN_POINT('Ctrl Pts',(-37.0208955392833,17.9290397288272,-2.96326313438592));
#38552=CARTESIAN_POINT('Ctrl Pts',(-37.0507916007085,17.9123870158746,-2.5));
#38553=CARTESIAN_POINT('Ctrl Pts',(-37.4571637864037,17.6853590086553,-2.5));
#38554=CARTESIAN_POINT('Ctrl Pts',(-37.0636620936595,17.9942014163556,-2.95683590040463));
#38555=CARTESIAN_POINT('Ctrl Pts',(-37.0962159645972,17.9716354404605,-2.5));
#38556=CARTESIAN_POINT('Ctrl Pts',(-37.4732012555054,17.7101600273524,-2.5));
#38557=CARTESIAN_POINT('Ctrl Pts',(-37.0790511866489,18.0153339916105,-2.95473552840589));
#38558=CARTESIAN_POINT('Ctrl Pts',(-37.1122588011471,17.9906733177174,-2.5));
#38559=CARTESIAN_POINT('Ctrl Pts',(-37.4789721679196,17.7182046074472,-2.5));
#38560=CARTESIAN_POINT('Ctrl Pts',(-37.1121011063091,18.0562700748877,-2.95063882870761));
#38561=CARTESIAN_POINT('Ctrl Pts',(-37.1461872334036,18.0272996809472,-2.5));
#38562=CARTESIAN_POINT('Ctrl Pts',(-37.4913658752322,17.733790264152,-2.5));
#38563=CARTESIAN_POINT('Ctrl Pts',(-37.1295103581676,18.0757653348942,-2.94867340342006));
#38564=CARTESIAN_POINT('Ctrl Pts',(-37.1638134804818,18.0446236356694,-2.5));
#38565=CARTESIAN_POINT('Ctrl Pts',(-37.4978943532022,17.7412139562433,-2.5));
#38566=CARTESIAN_POINT('Ctrl Pts',(-37.1843057553075,18.1314233942583,-2.94302770433399));
#38567=CARTESIAN_POINT('Ctrl Pts',(-37.2185148052678,18.0936922878623,-2.5));
#38568=CARTESIAN_POINT('Ctrl Pts',(-37.5184426204004,17.7624112761694,-2.5));
#38569=CARTESIAN_POINT('Ctrl Pts',(-37.2242361969918,18.1647864737446,-2.93959528754205));
#38570=CARTESIAN_POINT('Ctrl Pts',(-37.2575873678388,18.1227938260313,-2.5));
#38571=CARTESIAN_POINT('Ctrl Pts',(-37.5334165320212,17.7751217694643,-2.5));
#38572=CARTESIAN_POINT('Ctrl Pts',(-37.278501267837,18.2017080527822,-2.93576187067611));
#38573=CARTESIAN_POINT('Ctrl Pts',(-37.3098415222596,18.154743770369,-2.5));
#38574=CARTESIAN_POINT('Ctrl Pts',(-37.5537659442094,17.7891910078983,-2.5));
#38575=CARTESIAN_POINT('Ctrl Pts',(-37.2895908939828,18.2088614252754,-2.9350171685076));
#38576=CARTESIAN_POINT('Ctrl Pts',(-37.3204553852497,18.1609059986669,-2.5));
#38577=CARTESIAN_POINT('Ctrl Pts',(-37.5579245541323,17.7919170308987,-2.5));
#38578=CARTESIAN_POINT('Ctrl Pts',(-37.3121456740118,18.222628713375,-2.93358056573866));
#38579=CARTESIAN_POINT('Ctrl Pts',(-37.3419594345533,18.1727383129417,-2.5));
#38580=CARTESIAN_POINT('Ctrl Pts',(-37.5663825921581,17.7971638038772,-2.5));
#38581=CARTESIAN_POINT('Ctrl Pts',(-37.3235504689819,18.2292070024891,-2.93289238561845));
#38582=CARTESIAN_POINT('Ctrl Pts',(-37.3527929576584,18.1783789941509,-2.5));
#38583=CARTESIAN_POINT('Ctrl Pts',(-37.5706593939047,17.7996709619125,-2.5));
#38584=CARTESIAN_POINT('Ctrl Pts',(-37.3581397345302,18.2480437180578,-2.93091764257171));
#38585=CARTESIAN_POINT('Ctrl Pts',(-37.3855178350711,18.1944875128524,-2.5));
#38586=CARTESIAN_POINT('Ctrl Pts',(-37.5836303643146,17.8068505202015,-2.5));
#38587=CARTESIAN_POINT('Ctrl Pts',(-37.3816981781207,18.2594061256977,-2.92972067272748));
#38588=CARTESIAN_POINT('Ctrl Pts',(-37.4076765730136,18.2041692805068,-2.5));
#38589=CARTESIAN_POINT('Ctrl Pts',(-37.5924647836065,17.811181769741,-2.5));
#38590=CARTESIAN_POINT('Ctrl Pts',(-37.4297964715305,18.2797809159781,-2.92756741754469));
#38591=CARTESIAN_POINT('Ctrl Pts',(-37.4526661261266,18.2214705311287,-2.5));
#38592=CARTESIAN_POINT('Ctrl Pts',(-37.6105016433052,17.8189490809156,-2.5));
#38593=CARTESIAN_POINT('Ctrl Pts',(-37.4543363298823,18.2887932678948,-2.92661112217483));
#38594=CARTESIAN_POINT('Ctrl Pts',(-37.4755052012686,18.2290974806186,-2.5));
#38595=CARTESIAN_POINT('Ctrl Pts',(-37.6197040888717,17.8223851300001,-2.5));
#38596=CARTESIAN_POINT('Ctrl Pts',(-37.4918913116176,18.3005282374446,-2.92536297515959));
#38597=CARTESIAN_POINT('Ctrl Pts',(-37.5103223388011,18.2390056374751,-2.5));
#38598=CARTESIAN_POINT('Ctrl Pts',(-37.633787209243,17.8268594543971,-2.5));
#38599=CARTESIAN_POINT('Ctrl Pts',(-37.5045340558524,18.3041421023044,-2.92497802297482));
#38600=CARTESIAN_POINT('Ctrl Pts',(-37.5220166849113,18.2420518473036,-2.5));
#38601=CARTESIAN_POINT('Ctrl Pts',(-37.6385282366181,17.8282374131812,-2.5));
#38602=CARTESIAN_POINT('Ctrl Pts',(-37.5236880380742,18.3091085696021,-2.92444842107095));
#38603=CARTESIAN_POINT('Ctrl Pts',(-37.5397059345923,18.2462341178242,-2.5));
#38604=CARTESIAN_POINT('Ctrl Pts',(-37.6457109814105,17.8301311528227,-2.5));
#38605=CARTESIAN_POINT('Ctrl Pts',(-37.530104354971,18.310688300037,-2.92427986194296));
#38606=CARTESIAN_POINT('Ctrl Pts',(-37.5456258343898,18.2475634797771,-2.5));
#38607=CARTESIAN_POINT('Ctrl Pts',(-37.6481170992389,17.8307335274115,-2.5));
#38608=CARTESIAN_POINT('Ctrl Pts',(-37.5430010389201,18.3136945178689,-2.9239589307846));
#38609=CARTESIAN_POINT('Ctrl Pts',(-37.5575155990342,18.2500919427414,-2.5));
#38610=CARTESIAN_POINT('Ctrl Pts',(-37.6529533567628,17.8318798449285,-2.5));
#38611=CARTESIAN_POINT('Ctrl Pts',(-37.5494894557846,18.3151225191071,-2.92380639706833));
#38612=CARTESIAN_POINT('Ctrl Pts',(-37.5634930070409,18.2512923999885,-2.5));
#38613=CARTESIAN_POINT('Ctrl Pts',(-37.6553865130038,17.8324243739287,-2.5));
#38614=CARTESIAN_POINT('Ctrl Pts',(-37.6078715508142,18.3272151542962,-2.92251412976417));
#38615=CARTESIAN_POINT('Ctrl Pts',(-37.6171933811497,18.261444733944,-2.5));
#38616=CARTESIAN_POINT('Ctrl Pts',(-37.6772797946946,17.8370356375276,-2.5));
#38617=CARTESIAN_POINT('Ctrl Pts',(-37.6600314084477,18.3327140130362,-2.92192313396902));
#38618=CARTESIAN_POINT('Ctrl Pts',(-37.6650031743221,18.2660494018553,-2.5));
#38619=CARTESIAN_POINT('Ctrl Pts',(-37.6968397447769,17.8391327868468,-2.5));
#38620=CARTESIAN_POINT('Ctrl Pts',(-37.7386551922739,18.3333477986367,-2.92185513454714));
#38621=CARTESIAN_POINT('Ctrl Pts',(-37.7369884997638,18.2665799642824,-2.5));
#38622=CARTESIAN_POINT('Ctrl Pts',(-37.7263236637676,17.8393744833388,-2.5));
#38623=CARTESIAN_POINT('Ctrl Pts',(-37.7649275847458,18.332280602678,-2.92196969819476));
#38624=CARTESIAN_POINT('Ctrl Pts',(-37.7610453062294,18.2656866234871,-2.5));
#38625=CARTESIAN_POINT('Ctrl Pts',(-37.7361758116312,17.8389674969796,-2.5));
#38626=CARTESIAN_POINT('Ctrl Pts',(-37.8044355425913,18.3287092953001,-2.9223525645861));
#38627=CARTESIAN_POINT('Ctrl Pts',(-37.7972513234411,18.2626950729203,-2.5));
#38628=CARTESIAN_POINT('Ctrl Pts',(-37.7509912947654,17.8376055413245,-2.5));
#38629=CARTESIAN_POINT('Ctrl Pts',(-37.8176556209491,18.3271839572083,-2.92251604054704));
#38630=CARTESIAN_POINT('Ctrl Pts',(-37.8093757241164,18.2614166995762,-2.5));
#38631=CARTESIAN_POINT('Ctrl Pts',(-37.7559488239131,17.8370238468006,-2.5));
#38632=CARTESIAN_POINT('Ctrl Pts',(-37.8438653515097,18.3235000632348,-2.92291055095015));
#38633=CARTESIAN_POINT('Ctrl Pts',(-37.8334337540048,18.2583273875558,-2.5));
#38634=CARTESIAN_POINT('Ctrl Pts',(-37.7657774740514,17.8356190137894,-2.5));
#38635=CARTESIAN_POINT('Ctrl Pts',(-37.8568746743686,18.321341537448,-2.92314158144293));
#38636=CARTESIAN_POINT('Ctrl Pts',(-37.8453867146324,18.256516085823,-2.5));
#38637=CARTESIAN_POINT('Ctrl Pts',(-37.7706559690046,17.8347958710238,-2.5));
#38638=CARTESIAN_POINT('Ctrl Pts',(-37.9214525991908,18.3089956020391,-2.92446167772975));
#38639=CARTESIAN_POINT('Ctrl Pts',(-37.9048311581349,18.2461405986857,-2.5));
#38640=CARTESIAN_POINT('Ctrl Pts',(-37.7948726934621,17.8300879827949,-2.5));
#38641=CARTESIAN_POINT('Ctrl Pts',(-37.971628515283,18.2941930137726,-2.92604160841261));
#38642=CARTESIAN_POINT('Ctrl Pts',(-37.951260778169,18.233665691823,-2.5));
#38643=CARTESIAN_POINT('Ctrl Pts',(-37.8136886637651,17.8244435332827,-2.5));
#38644=CARTESIAN_POINT('Ctrl Pts',(-38.0324952429552,18.2695437413729,-2.9286496092432));
#38645=CARTESIAN_POINT('Ctrl Pts',(-38.0080199920834,18.2127861786537,-2.5));
#38646=CARTESIAN_POINT('Ctrl Pts',(-37.8365136817825,17.8150464189915,-2.5));
#38647=CARTESIAN_POINT('Ctrl Pts',(-38.044575088039,18.264303794869,-2.92920311231327));
#38648=CARTESIAN_POINT('Ctrl Pts',(-38.0193295823946,18.208334158798,-2.5));
#38649=CARTESIAN_POINT('Ctrl Pts',(-37.8410436263355,17.8130488679072,-2.5));
#38650=CARTESIAN_POINT('Ctrl Pts',(-38.0685444585904,18.2531925029883,-2.93037437162195));
#38651=CARTESIAN_POINT('Ctrl Pts',(-38.0418344218168,18.1988760473144,-2.5));
#38652=CARTESIAN_POINT('Ctrl Pts',(-37.850032136943,17.8088132624928,-2.5));
#38653=CARTESIAN_POINT('Ctrl Pts',(-38.0804306041699,18.2473200654554,-2.93099223718261));
#38654=CARTESIAN_POINT('Ctrl Pts',(-38.0530277696176,18.1938679552602,-2.5));
#38655=CARTESIAN_POINT('Ctrl Pts',(-37.8544894413598,17.8065748058377,-2.5));
#38656=CARTESIAN_POINT('Ctrl Pts',(-38.1154058739446,18.2289535054552,-2.93292028761117));
#38657=CARTESIAN_POINT('Ctrl Pts',(-38.0860884329982,18.1781636427194,-2.5));
#38658=CARTESIAN_POINT('Ctrl Pts',(-37.8676051730758,17.7995742349009,-2.5));
#38659=CARTESIAN_POINT('Ctrl Pts',(-38.1379498775984,18.2156512801827,-2.93431116406502));
#38660=CARTESIAN_POINT('Ctrl Pts',(-38.107532686332,18.1667488029368,-2.5));
#38661=CARTESIAN_POINT('Ctrl Pts',(-37.8760591693826,17.7945044510302,-2.5));
#38662=CARTESIAN_POINT('Ctrl Pts',(-38.2033280576451,18.17265741314,-2.93878236806526));
#38663=CARTESIAN_POINT('Ctrl Pts',(-38.1702794467489,18.1296291178422,-2.5));
#38664=CARTESIAN_POINT('Ctrl Pts',(-37.9005759909892,17.7781206666248,-2.5));
#38665=CARTESIAN_POINT('Ctrl Pts',(-38.2439301407294,18.1399084455847,-2.94215865140722));
#38666=CARTESIAN_POINT('Ctrl Pts',(-38.2098765411374,18.1011163150348,-2.5));
#38667=CARTESIAN_POINT('Ctrl Pts',(-37.9158017810326,17.7656435334912,-2.5));
#38668=CARTESIAN_POINT('Ctrl Pts',(-38.2908370693989,18.0936969886663,-2.94685549765066));
#38669=CARTESIAN_POINT('Ctrl Pts',(-38.2564928085569,18.0604885105553,-2.5));
#38670=CARTESIAN_POINT('Ctrl Pts',(-37.9333918647676,17.7480431201017,-2.5));
#38671=CARTESIAN_POINT('Ctrl Pts',(-38.2999735282245,18.0842373184233,-2.94781393656573));
#38672=CARTESIAN_POINT('Ctrl Pts',(-38.2656503724343,18.0521248196139,-2.5));
#38673=CARTESIAN_POINT('Ctrl Pts',(-37.9368180370691,17.744440511481,-2.5));
#38674=CARTESIAN_POINT('Ctrl Pts',(-38.3176873507553,18.0649722522993,-2.94975921175979));
#38675=CARTESIAN_POINT('Ctrl Pts',(-38.2835158468797,18.035036707545,-2.5));
#38676=CARTESIAN_POINT('Ctrl Pts',(-37.9434607258409,17.7371042069719,-2.5));
#38677=CARTESIAN_POINT('Ctrl Pts',(-38.3262776360071,18.0551541758763,-2.95074733976652));
#38678=CARTESIAN_POINT('Ctrl Pts',(-38.292236426,18.0262999067001,-2.5));
#38679=CARTESIAN_POINT('Ctrl Pts',(-37.9466820784148,17.7333656728621,-2.5));
#38680=CARTESIAN_POINT('Ctrl Pts',(-38.3512613834271,18.0251519219321,-2.95375629684687));
#38681=CARTESIAN_POINT('Ctrl Pts',(-38.3177954315766,17.9994877930366,-2.5));
#38682=CARTESIAN_POINT('Ctrl Pts',(-37.9560509888996,17.721942323421,-2.5));
#38683=CARTESIAN_POINT('Ctrl Pts',(-38.3668695803311,18.0044210131818,-2.95582157994119));
#38684=CARTESIAN_POINT('Ctrl Pts',(-38.3339844060987,17.9808535987548,-2.5));
#38685=CARTESIAN_POINT('Ctrl Pts',(-37.9619040598854,17.7140502257561,-2.5));
#38686=CARTESIAN_POINT('Ctrl Pts',(-38.3960122766866,17.96151412598,-2.96006384799544));
#38687=CARTESIAN_POINT('Ctrl Pts',(-38.3647032001448,17.9420087393569,-2.5));
#38688=CARTESIAN_POINT('Ctrl Pts',(-37.9728325697887,17.6977186737315,-2.5));
#38689=CARTESIAN_POINT('Ctrl Pts',(-38.4095468146066,17.9393381811376,-2.96224084544494));
#38690=CARTESIAN_POINT('Ctrl Pts',(-38.3792301089262,17.921787539762,-2.5));
#38691=CARTESIAN_POINT('Ctrl Pts',(-37.9779080274105,17.6892792325375,-2.5));
#38692=CARTESIAN_POINT('Ctrl Pts',(-38.4282645108262,17.904969535058,-2.96558787871309));
#38693=CARTESIAN_POINT('Ctrl Pts',(-38.399714653804,17.8902405113807,-2.5));
#38694=CARTESIAN_POINT('Ctrl Pts',(-37.9849271555627,17.6762019272695,-2.5));
#38695=CARTESIAN_POINT('Ctrl Pts',(-38.4342446366122,17.89331766282,-2.96671826104229));
#38696=CARTESIAN_POINT('Ctrl Pts',(-38.4063407380303,17.8794930259532,-2.5));
#38697=CARTESIAN_POINT('Ctrl Pts',(-37.9871697012262,17.6717687488141,-2.5));
#38698=CARTESIAN_POINT('Ctrl Pts',(-38.4456424175336,17.8696845533725,-2.96900170083772));
#38699=CARTESIAN_POINT('Ctrl Pts',(-38.4191252098151,17.8576079915772,-2.5));
#38700=CARTESIAN_POINT('Ctrl Pts',(-37.991443877371,17.6627778699454,-2.5));
#38701=CARTESIAN_POINT('Ctrl Pts',(-38.4510249910641,17.8577775263316,-2.9701475957582));
#38702=CARTESIAN_POINT('Ctrl Pts',(-38.4252432488303,17.8465380939854,-2.5));
#38703=CARTESIAN_POINT('Ctrl Pts',(-37.9934623353037,17.6582483931711,-2.5));
#38704=CARTESIAN_POINT('Ctrl Pts',(-38.4763900971177,17.7977995570222,-2.97589627219185));
#38705=CARTESIAN_POINT('Ctrl Pts',(-38.4545812226388,17.790369539723,-2.5));
#38706=CARTESIAN_POINT('Ctrl Pts',(-38.002974265032,17.6354345524181,-2.5));
#38707=CARTESIAN_POINT('Ctrl Pts',(-38.4917731732021,17.7484124059281,-2.98055544920644));
#38708=CARTESIAN_POINT('Ctrl Pts',(-38.473661265785,17.7435263663243,-2.5));
#38709=CARTESIAN_POINT('Ctrl Pts',(-38.0087429143111,17.6166554164039,-2.5));
#38710=CARTESIAN_POINT('Ctrl Pts',(-38.5049497227733,17.6849440597232,-2.9864412217583));
#38711=CARTESIAN_POINT('Ctrl Pts',(-38.4919775578133,17.6825071777955,-2.5));
#38712=CARTESIAN_POINT('Ctrl Pts',(-38.0136841107577,17.5925304537987,-2.5));
#38713=CARTESIAN_POINT('Ctrl Pts',(-38.5072797054594,17.6721629059777,-2.9876215411643));
#38714=CARTESIAN_POINT('Ctrl Pts',(-38.4953743016544,17.6701248728446,-2.5));
#38715=CARTESIAN_POINT('Ctrl Pts',(-38.0145578594488,17.5876726194739,-2.5));
#38716=CARTESIAN_POINT('Ctrl Pts',(-38.5113201026512,17.646423044551,-2.98998846097813));
#38717=CARTESIAN_POINT('Ctrl Pts',(-38.501596520551,17.645080935214,-2.5));
#38718=CARTESIAN_POINT('Ctrl Pts',(-38.0160730018852,17.5778902994518,-2.5));
#38719=CARTESIAN_POINT('Ctrl Pts',(-38.5130325575213,17.6334445126556,-2.99117686889631));
#38720=CARTESIAN_POINT('Ctrl Pts',(-38.5044245550668,17.6323990130624,-2.5));
#38721=CARTESIAN_POINT('Ctrl Pts',(-38.0167151730816,17.5729582831273,-2.5));
#38722=CARTESIAN_POINT('Ctrl Pts',(-38.5172060896891,17.5943721213219,-2.99473928414168));
#38723=CARTESIAN_POINT('Ctrl Pts',(-38.5120043473919,17.5940082770842,-2.5));
#38724=CARTESIAN_POINT('Ctrl Pts',(-38.0182802555498,17.5581115117232,-2.5));
#38725=CARTESIAN_POINT('Ctrl Pts',(-38.5186917422194,17.5683120165936,-2.99709499970835));
#38726=CARTESIAN_POINT('Ctrl Pts',(-38.5157988525533,17.5682102346573,-2.5));
#38727=CARTESIAN_POINT('Ctrl Pts',(-38.0188373699573,17.5482108332471,-2.5));
#38728=CARTESIAN_POINT('Ctrl Pts',(-38.5191072198307,17.5161686034308,-3.00176886678129));
#38729=CARTESIAN_POINT('Ctrl Pts',(-38.5208771553493,17.5161399120222,-2.5));
#38730=CARTESIAN_POINT('Ctrl Pts',(-38.0189931741039,17.5284038967669,-2.5));
#38731=CARTESIAN_POINT('Ctrl Pts',(-38.5180370412835,17.4900852974077,-3.00408701695548));
#38732=CARTESIAN_POINT('Ctrl Pts',(-38.5221491625175,17.4898665253747,-2.5));
#38733=CARTESIAN_POINT('Ctrl Pts',(-38.0185918623631,17.5184976387542,-2.5));
#38734=CARTESIAN_POINT('Ctrl Pts',(-38.5144871859473,17.4509429730902,-3.00753674366307));
#38735=CARTESIAN_POINT('Ctrl Pts',(-38.5220957984724,17.4501405073408,-2.5));
#38736=CARTESIAN_POINT('Ctrl Pts',(-38.0172606587587,17.5036340064431,-2.5));
#38737=CARTESIAN_POINT('Ctrl Pts',(-38.512979645677,17.4379142878159,-3.00868013835556));
#38738=CARTESIAN_POINT('Ctrl Pts',(-38.5217466988597,17.4368445410147,-2.5));
#38739=CARTESIAN_POINT('Ctrl Pts',(-38.0166953304505,17.4986869777819,-2.5));
#38740=CARTESIAN_POINT('Ctrl Pts',(-38.5093456409823,17.4120774324436,-3.01093824610606));
#38741=CARTESIAN_POINT('Ctrl Pts',(-38.5203938380985,17.4103637207151,-2.5));
#38742=CARTESIAN_POINT('Ctrl Pts',(-38.0153325853393,17.4888774005165,-2.5));
#38743=CARTESIAN_POINT('Ctrl Pts',(-38.5072169868592,17.3992427493601,-3.01205529745571));
#38744=CARTESIAN_POINT('Ctrl Pts',(-38.5193887795888,17.3971525411347,-2.5));
#38745=CARTESIAN_POINT('Ctrl Pts',(-38.014534334724,17.4840047859771,-2.5));
#38746=CARTESIAN_POINT('Ctrl Pts',(-38.4950383810716,17.335482072003,-3.01758225181016));
#38747=CARTESIAN_POINT('Ctrl Pts',(-38.512708363373,17.3310164313404,-2.5));
#38748=CARTESIAN_POINT('Ctrl Pts',(-38.0099673675257,17.4598001953765,-2.5));
#38749=CARTESIAN_POINT('Ctrl Pts',(-38.4804258988967,17.2857825382543,-3.02181836676292));
#38750=CARTESIAN_POINT('Ctrl Pts',(-38.5021474563194,17.2787657562271,-2.5));
#38751=CARTESIAN_POINT('Ctrl Pts',(-38.0044876905449,17.4409392110453,-2.5));
#38752=CARTESIAN_POINT('Ctrl Pts',(-38.4559979025521,17.2253187773268,-3.02689693274587));
#38753=CARTESIAN_POINT('Ctrl Pts',(-38.482188384964,17.2143685236006,-2.5));
#38754=CARTESIAN_POINT('Ctrl Pts',(-37.9953271771502,17.4179991279534,-2.5));
#38755=CARTESIAN_POINT('Ctrl Pts',(-38.4508014471794,17.2133098047403,-3.02790174447839));
#38756=CARTESIAN_POINT('Ctrl Pts',(-38.4778364738777,17.2014855815011,-2.5));
#38757=CARTESIAN_POINT('Ctrl Pts',(-37.9933785134793,17.4134431981463,-2.5));
#38758=CARTESIAN_POINT('Ctrl Pts',(-38.4425304868847,17.1954247892708,-3.02939268814916));
#38759=CARTESIAN_POINT('Ctrl Pts',(-38.4707770006933,17.1822327898589,-2.5));
#38760=CARTESIAN_POINT('Ctrl Pts',(-37.9902768971576,17.4066584740223,-2.5));
#38761=CARTESIAN_POINT('Ctrl Pts',(-38.4396936273783,17.1894842833032,-3.02988697260699));
#38762=CARTESIAN_POINT('Ctrl Pts',(-38.4683326604495,17.1758218953105,-2.5));
#38763=CARTESIAN_POINT('Ctrl Pts',(-37.9892130751568,17.4044050008767,-2.5));
#38764=CARTESIAN_POINT('Ctrl Pts',(-38.433892526343,17.1777122168892,-3.03086468827693));
#38765=CARTESIAN_POINT('Ctrl Pts',(-38.4632915541776,17.1630927437411,-2.5));
#38766=CARTESIAN_POINT('Ctrl Pts',(-37.9870376657812,17.3999395207739,-2.5));
#38767=CARTESIAN_POINT('Ctrl Pts',(-38.4309245022383,17.1718722889636,-3.03134881683581));
#38768=CARTESIAN_POINT('Ctrl Pts',(-38.4606914472883,17.1567656550912,-2.5));
#38769=CARTESIAN_POINT('Ctrl Pts',(-37.9859246535537,17.3977243429034,-2.5));
#38770=CARTESIAN_POINT('Ctrl Pts',(-38.4157502976598,17.1429009507965,-3.03374623521863));
#38771=CARTESIAN_POINT('Ctrl Pts',(-38.4472751802113,17.1252685427155,-2.5));
#38772=CARTESIAN_POINT('Ctrl Pts',(-37.9802343339963,17.3867353766995,-2.5));
#38773=CARTESIAN_POINT('Ctrl Pts',(-38.4025443177972,17.1204528053856,-3.03559000380591));
#38774=CARTESIAN_POINT('Ctrl Pts',(-38.4352923297066,17.1007128648909,-2.5));
#38775=CARTESIAN_POINT('Ctrl Pts',(-37.9752820848364,17.3782217794531,-2.5));
#38776=CARTESIAN_POINT('Ctrl Pts',(-38.3597927098826,17.0552514733911,-3.04091068696068));
#38777=CARTESIAN_POINT('Ctrl Pts',(-38.3955062069388,17.0287324610293,-2.5));
#38778=CARTESIAN_POINT('Ctrl Pts',(-37.9592502348198,17.3534964507582,-2.5));
#38779=CARTESIAN_POINT('Ctrl Pts',(-38.3271443327293,17.0146202226201,-3.04417881485026));
#38780=CARTESIAN_POINT('Ctrl Pts',(-38.3640171485458,16.9833146484955,-2.5));
#38781=CARTESIAN_POINT('Ctrl Pts',(-37.9470071050743,17.3380921508149,-2.5));
#38782=CARTESIAN_POINT('Ctrl Pts',(-38.2809131555838,16.9675438780044,-3.0479256286666));
#38783=CARTESIAN_POINT('Ctrl Pts',(-38.3181512189723,16.9301557601742,-2.5));
#38784=CARTESIAN_POINT('Ctrl Pts',(-37.9296703965765,17.3202474359949,-2.5));
#38785=CARTESIAN_POINT('Ctrl Pts',(-38.2714380751677,16.9583630961748,-3.04865416425237));
#38786=CARTESIAN_POINT('Ctrl Pts',(-38.3086648857525,16.9197304651529,-2.5));
#38787=CARTESIAN_POINT('Ctrl Pts',(-37.9261172426642,17.3167675393722,-2.5));
#38788=CARTESIAN_POINT('Ctrl Pts',(-38.2521347050763,16.9405580024456,-3.05006336142326));
#38789=CARTESIAN_POINT('Ctrl Pts',(-38.2892172779821,16.8994516379931,-2.5));
#38790=CARTESIAN_POINT('Ctrl Pts',(-37.9188784832198,17.3100189529994,-2.5));
#38791=CARTESIAN_POINT('Ctrl Pts',(-38.2422914181653,16.9319183323786,-3.05074524347667));
#38792=CARTESIAN_POINT('Ctrl Pts',(-38.2792412041749,16.8895824979303,-2.5));
#38793=CARTESIAN_POINT('Ctrl Pts',(-37.9151872472733,17.3067444493034,-2.5));
#38794=CARTESIAN_POINT('Ctrl Pts',(-38.2121946005029,16.9067773575311,-3.05272459995863));
#38795=CARTESIAN_POINT('Ctrl Pts',(-38.2485441235301,16.860762254136,-2.5));
#38796=CARTESIAN_POINT('Ctrl Pts',(-37.9039009442048,17.2972161773508,-2.5));
#38797=CARTESIAN_POINT('Ctrl Pts',(-38.1913754559341,16.8910522598471,-3.05395594589729));
#38798=CARTESIAN_POINT('Ctrl Pts',(-38.227102342556,16.842648790628,-2.5));
#38799=CARTESIAN_POINT('Ctrl Pts',(-37.8960937635255,17.2912569793141,-2.5));
#38800=CARTESIAN_POINT('Ctrl Pts',(-38.1482366444428,16.861662216655,-3.05624785925289));
#38801=CARTESIAN_POINT('Ctrl Pts',(-38.1822556751584,16.8086281750341,-2.5));
#38802=CARTESIAN_POINT('Ctrl Pts',(-37.8799167074083,17.280120019,-2.5));
#38803=CARTESIAN_POINT('Ctrl Pts',(-38.1259170445788,16.8479971821675,-3.05730841943199));
#38804=CARTESIAN_POINT('Ctrl Pts',(-38.1588541824173,16.7927328735794,-2.5));
#38805=CARTESIAN_POINT('Ctrl Pts',(-37.8715468617295,17.274942215395,-2.5));
#38806=CARTESIAN_POINT('Ctrl Pts',(-38.0912859803399,16.829081464749,-3.05877140147105));
#38807=CARTESIAN_POINT('Ctrl Pts',(-38.1222868782628,16.7706491428746,-2.5));
#38808=CARTESIAN_POINT('Ctrl Pts',(-37.8585602075906,17.2677752860875,-2.5));
#38809=CARTESIAN_POINT('Ctrl Pts',(-38.0795482163152,16.8230394748505,-3.05923777409933));
#38810=CARTESIAN_POINT('Ctrl Pts',(-38.1098421306826,16.7635765111134,-2.5));
#38811=CARTESIAN_POINT('Ctrl Pts',(-37.854158548831,17.2654861133914,-2.5));
#38812=CARTESIAN_POINT('Ctrl Pts',(-38.0556863997546,16.8114994618048,-3.06012706376275));
#38813=CARTESIAN_POINT('Ctrl Pts',(-38.0844586622232,16.7500420272248,-2.5));
#38814=CARTESIAN_POINT('Ctrl Pts',(-37.8452103654877,17.2611139901796,-2.5));
#38815=CARTESIAN_POINT('Ctrl Pts',(-38.0436500462945,16.8060440839517,-3.06054669237718));
#38816=CARTESIAN_POINT('Ctrl Pts',(-38.0716141384825,16.7436315079723,-2.5));
#38817=CARTESIAN_POINT('Ctrl Pts',(-37.8406967327678,17.2590471876283,-2.5));
#38818=CARTESIAN_POINT('Ctrl Pts',(-37.983033732995,16.7803474050268,-3.06252042955387));
#38819=CARTESIAN_POINT('Ctrl Pts',(-38.006651933923,16.7133430503521,-2.5));
#38820=CARTESIAN_POINT('Ctrl Pts',(-37.817965621475,17.2493120442009,-2.5));
#38821=CARTESIAN_POINT('Ctrl Pts',(-37.9330756082843,16.7647592929747,-3.06370859239269));
#38822=CARTESIAN_POINT('Ctrl Pts',(-37.9526360706556,16.6948699048902,-2.5));
#38823=CARTESIAN_POINT('Ctrl Pts',(-37.7992313215639,17.2434072153618,-2.5));
#38824=CARTESIAN_POINT('Ctrl Pts',(-37.8688152137882,16.7514251465279,-3.06472324864037));
#38825=CARTESIAN_POINT('Ctrl Pts',(-37.8827461609207,16.6790214482703,-2.5));
#38826=CARTESIAN_POINT('Ctrl Pts',(-37.7751336713641,17.2383563320521,-2.5));
#38827=CARTESIAN_POINT('Ctrl Pts',(-37.8558716761049,16.7490686581359,-3.06490240337987));
#38828=CARTESIAN_POINT('Ctrl Pts',(-37.8686399794402,16.6762161508003,-2.5));
#38829=CARTESIAN_POINT('Ctrl Pts',(-37.7702798457447,17.2374637147322,-2.5));
#38830=CARTESIAN_POINT('Ctrl Pts',(-37.836316999401,16.7460068446618,-3.06513506367886));
#38831=CARTESIAN_POINT('Ctrl Pts',(-37.8473067499512,16.6725690712863,-2.5));
#38832=CARTESIAN_POINT('Ctrl Pts',(-37.762946841142,17.2363039481978,-2.5));
#38833=CARTESIAN_POINT('Ctrl Pts',(-37.829775537342,16.7450650975492,-3.06520660039349));
#38834=CARTESIAN_POINT('Ctrl Pts',(-37.8401659882031,16.6714468083953,-2.5));
#38835=CARTESIAN_POINT('Ctrl Pts',(-37.7604937934312,17.23594722548,-2.5));
#38836=CARTESIAN_POINT('Ctrl Pts',(-37.8166456311835,16.7433410180028,-3.0653375358751));
#38837=CARTESIAN_POINT('Ctrl Pts',(-37.82582654984,16.669391703467,-2.5));
#38838=CARTESIAN_POINT('Ctrl Pts',(-37.7555700780584,17.2352941782029,-2.5));
#38839=CARTESIAN_POINT('Ctrl Pts',(-37.8100479347227,16.7425577604292,-3.06539700330435));
#38840=CARTESIAN_POINT('Ctrl Pts',(-37.818617934926,16.668457783908,-2.5));
#38841=CARTESIAN_POINT('Ctrl Pts',(-37.7530959419294,17.2349974951212,-2.5));
#38842=CARTESIAN_POINT('Ctrl Pts',(-37.777067284866,16.7390579643222,-3.06566266886128));
#38843=CARTESIAN_POINT('Ctrl Pts',(-37.7825632243643,16.6642830215665,-2.5));
#38844=CARTESIAN_POINT('Ctrl Pts',(-37.7407281994226,17.2336718308661,-2.5));
#38845=CARTESIAN_POINT('Ctrl Pts',(-37.7507569280122,16.7375882697876,-3.06577409663493));
#38846=CARTESIAN_POINT('Ctrl Pts',(-37.7537706577765,16.6625286572503,-2.5));
#38847=CARTESIAN_POINT('Ctrl Pts',(-37.7308618146269,17.2331151625715,-2.5));
#38848=CARTESIAN_POINT('Ctrl Pts',(-37.6720409935013,16.7370385868534,-3.06581578422071));
#38849=CARTESIAN_POINT('Ctrl Pts',(-37.6675998077381,16.6618723975768,-2.5));
#38850=CARTESIAN_POINT('Ctrl Pts',(-37.7013433392571,17.2329069461004,-2.5));
#38851=CARTESIAN_POINT('Ctrl Pts',(-37.6198485285534,16.7417812990776,-3.06545669284864));
#38852=CARTESIAN_POINT('Ctrl Pts',(-37.6105054868964,16.6675345545024,-2.5));
#38853=CARTESIAN_POINT('Ctrl Pts',(-37.6817711620469,17.2347033137879,-2.5));
#38854=CARTESIAN_POINT('Ctrl Pts',(-37.5549716201007,16.7542328279335,-3.06450964654665));
#38855=CARTESIAN_POINT('Ctrl Pts',(-37.539791579201,16.6823618030451,-2.5));
#38856=CARTESIAN_POINT('Ctrl Pts',(-37.6574423248857,17.2394198627989,-2.5));
#38857=CARTESIAN_POINT('Ctrl Pts',(-37.5419780772432,16.7570618699045,-3.06429433377577));
#38858=CARTESIAN_POINT('Ctrl Pts',(-37.5256575742345,16.6857256023118,-2.5));
#38859=CARTESIAN_POINT('Ctrl Pts',(-37.6525697466396,17.2404914902659,-2.5));
#38860=CARTESIAN_POINT('Ctrl Pts',(-37.5162549007385,16.7633361071356,-3.06381631649363));
#38861=CARTESIAN_POINT('Ctrl Pts',(-37.4977213282955,16.6931780113973,-2.5));
#38862=CARTESIAN_POINT('Ctrl Pts',(-37.642923553396,17.2428681687046,-2.5));
#38863=CARTESIAN_POINT('Ctrl Pts',(-37.5035214136028,16.7667796187423,-3.0635537446777));
#38864=CARTESIAN_POINT('Ctrl Pts',(-37.4839161235599,16.6972638969602,-2.5));
#38865=CARTESIAN_POINT('Ctrl Pts',(-37.6381484975799,17.2441725977466,-2.5));
#38866=CARTESIAN_POINT('Ctrl Pts',(-37.4656977945507,16.7780114577165,-3.06269625818825));
#38867=CARTESIAN_POINT('Ctrl Pts',(-37.4430016133797,16.7105699687229,-2.5));
#38868=CARTESIAN_POINT('Ctrl Pts',(-37.6239646379375,17.2484273528784,-2.5));
#38869=CARTESIAN_POINT('Ctrl Pts',(-37.4409836224016,16.7866989403601,-3.06203177270948));
#38870=CARTESIAN_POINT('Ctrl Pts',(-37.4163729269822,16.720839368388,-2.5));
#38871=CARTESIAN_POINT('Ctrl Pts',(-37.6146968252125,17.2517183816627,-2.5));
#38872=CARTESIAN_POINT('Ctrl Pts',(-37.3925416751236,16.80643246839,-3.06051737328866));
#38873=CARTESIAN_POINT('Ctrl Pts',(-37.3644453567216,16.7440900855917,-2.5));
#38874=CARTESIAN_POINT('Ctrl Pts',(-37.5965310946519,17.2591942841924,-2.5));
#38875=CARTESIAN_POINT('Ctrl Pts',(-37.3688139142769,16.8174785426132,-3.05966746752498));
#38876=CARTESIAN_POINT('Ctrl Pts',(-37.3391549609578,16.7570619950295,-2.5));
#38877=CARTESIAN_POINT('Ctrl Pts',(-37.5876331822018,17.2633791709517,-2.5));
#38878=CARTESIAN_POINT('Ctrl Pts',(-37.3339711607475,16.8358377670208,-3.05824914363553));
#38879=CARTESIAN_POINT('Ctrl Pts',(-37.3022443333108,16.7785464121055,-2.5));
#38880=CARTESIAN_POINT('Ctrl Pts',(-37.5745671530757,17.270335145276,-2.5));
#38881=CARTESIAN_POINT('Ctrl Pts',(-37.3224819496572,16.8422563904187,-3.05775241081752));
#38882=CARTESIAN_POINT('Ctrl Pts',(-37.2901231475283,16.7860382908692,-2.5));
#38883=CARTESIAN_POINT('Ctrl Pts',(-37.570258695808,17.2727671020922,-2.5));
#38884=CARTESIAN_POINT('Ctrl Pts',(-37.2997579173503,16.8557016280555,-3.05670968389331));
#38885=CARTESIAN_POINT('Ctrl Pts',(-37.2662411766355,16.8016967416051,-2.5));
#38886=CARTESIAN_POINT('Ctrl Pts',(-37.5617371876123,17.2778615635871,-2.5));
#38887=CARTESIAN_POINT('Ctrl Pts',(-37.2885084984505,16.8627400253605,-3.0561627663965));
#38888=CARTESIAN_POINT('Ctrl Pts',(-37.2544661462563,16.8098753233558,-2.5));
#38889=CARTESIAN_POINT('Ctrl Pts',(-37.5575186558127,17.2805285214769,-2.5));
#38890=CARTESIAN_POINT('Ctrl Pts',(-37.2335131076936,16.8990718659001,-3.05333313807168));
#38891=CARTESIAN_POINT('Ctrl Pts',(-37.1972561950466,16.8519104255022,-2.5));
#38892=CARTESIAN_POINT('Ctrl Pts',(-37.5368953730412,17.2942956929266,-2.5));
#38893=CARTESIAN_POINT('Ctrl Pts',(-37.1930113241315,16.9320140399769,-3.05074799765065));
#38894=CARTESIAN_POINT('Ctrl Pts',(-37.1558511506002,16.8897253205875,-2.5));
#38895=CARTESIAN_POINT('Ctrl Pts',(-37.5217072095524,17.3067799280439,-2.5));
#38896=CARTESIAN_POINT('Ctrl Pts',(-37.1373488654157,16.987068334806,-3.04637357495642));
#38897=CARTESIAN_POINT('Ctrl Pts',(-37.1001829683923,16.9522623708449,-2.5));
#38898=CARTESIAN_POINT('Ctrl Pts',(-37.5008337929987,17.3276482177729,-2.5));
#38899=CARTESIAN_POINT('Ctrl Pts',(-37.119649230241,17.0063667438965,-3.04483205480724));
#38900=CARTESIAN_POINT('Ctrl Pts',(-37.08275128213,16.9740145507512,-2.5));
#38901=CARTESIAN_POINT('Ctrl Pts',(-37.4941964218283,17.334963880511,-2.5));
#38902=CARTESIAN_POINT('Ctrl Pts',(-37.09862407612,17.0317074280592,-3.04279459962286));
#38903=CARTESIAN_POINT('Ctrl Pts',(-37.0623359323734,17.0024240843538,-2.5));
#38904=CARTESIAN_POINT('Ctrl Pts',(-37.4863119967309,17.344571096994,-2.5));
#38905=CARTESIAN_POINT('Ctrl Pts',(-37.0944707116322,17.0368412601703,-3.04238118958153));
#38906=CARTESIAN_POINT('Ctrl Pts',(-37.0583251973171,17.0081622414672,-2.5));
#38907=CARTESIAN_POINT('Ctrl Pts',(-37.4847544852643,17.3465174947961,-2.5));
#38908=CARTESIAN_POINT('Ctrl Pts',(-37.086318602129,17.0471765103316,-3.04154758456322));
#38909=CARTESIAN_POINT('Ctrl Pts',(-37.0504867079477,17.0196942280984,-2.5));
#38910=CARTESIAN_POINT('Ctrl Pts',(-37.4816974406886,17.350436015139,-2.5));
#38911=CARTESIAN_POINT('Ctrl Pts',(-37.0823147848581,17.0523838124048,-3.04112691976143));
#38912=CARTESIAN_POINT('Ctrl Pts',(-37.0466539524108,17.0254945229426,-2.5));
#38913=CARTESIAN_POINT('Ctrl Pts',(-37.4801960124776,17.3524103736432,-2.5));
#38914=CARTESIAN_POINT('Ctrl Pts',(-37.0705176170079,17.0681234054201,-3.03985333807572));
#38915=CARTESIAN_POINT('Ctrl Pts',(-37.0354170178543,17.0429878142689,-2.5));
#38916=CARTESIAN_POINT('Ctrl Pts',(-37.475772070005,17.3583782202939,-2.5));
#38917=CARTESIAN_POINT('Ctrl Pts',(-37.0629384235517,17.0787733000584,-3.03898884786155));
#38918=CARTESIAN_POINT('Ctrl Pts',(-37.0282631566779,17.0547884840968,-2.5));
#38919=CARTESIAN_POINT('Ctrl Pts',(-37.4729298774794,17.3624164681974,-2.5));
#38920=CARTESIAN_POINT('Ctrl Pts',(-37.026446523552,17.132793523799,-3.03458889787333));
#38921=CARTESIAN_POINT('Ctrl Pts',(-36.9942613247177,17.1142615428478,-2.5));
#38922=CARTESIAN_POINT('Ctrl Pts',(-37.4592454049732,17.3829010974121,-2.5));
#38923=CARTESIAN_POINT('Ctrl Pts',(-37.0017062809529,17.1784542255603,-3.03082304423241));
#38924=CARTESIAN_POINT('Ctrl Pts',(-36.9722499558993,17.1639506562642,-2.5));
#38925=CARTESIAN_POINT('Ctrl Pts',(-37.4499678115662,17.4002194094609,-2.5));
#38926=CARTESIAN_POINT('Ctrl Pts',(-36.9763738972329,17.2385950219028,-3.02578307239997));
#38927=CARTESIAN_POINT('Ctrl Pts',(-36.9511407639783,17.2285709769479,-2.5));
#38928=CARTESIAN_POINT('Ctrl Pts',(-37.4404681807179,17.4230360661467,-2.5));
#38929=CARTESIAN_POINT('Ctrl Pts',(-36.9715895606736,17.2507777927924,-3.02475831530062));
#38930=CARTESIAN_POINT('Ctrl Pts',(-36.9472559919366,17.2415671008265,-2.5));
#38931=CARTESIAN_POINT('Ctrl Pts',(-37.4386740479595,17.4276583514805,-2.5));
#38932=CARTESIAN_POINT('Ctrl Pts',(-36.9625961480096,17.2754584703774,-3.02267407819011));
#38933=CARTESIAN_POINT('Ctrl Pts',(-36.9401413648218,17.2677878485332,-2.5));
#38934=CARTESIAN_POINT('Ctrl Pts',(-37.4353015260892,17.4370231465561,-2.5));
#38935=CARTESIAN_POINT('Ctrl Pts',(-36.9584132845463,17.2878868497566,-3.02162045942486));
#38936=CARTESIAN_POINT('Ctrl Pts',(-36.9369311676226,17.2809375542772,-2.5));
#38937=CARTESIAN_POINT('Ctrl Pts',(-37.4337329516611,17.441739269899,-2.5));
#38938=CARTESIAN_POINT('Ctrl Pts',(-36.9468363797903,17.3252899977778,-3.01843695447992));
#38939=CARTESIAN_POINT('Ctrl Pts',(-36.9283615872827,17.3203042842923,-2.5));
#38940=CARTESIAN_POINT('Ctrl Pts',(-37.4293916024477,17.4559334232034,-2.5));
#38941=CARTESIAN_POINT('Ctrl Pts',(-36.9403896403824,17.3504426477826,-3.01627937557837));
#38942=CARTESIAN_POINT('Ctrl Pts',(-36.9240158817722,17.3465871928938,-2.5));
#38943=CARTESIAN_POINT('Ctrl Pts',(-37.4269740834161,17.4654799598295,-2.5));
#38944=CARTESIAN_POINT('Ctrl Pts',(-36.9299795767171,17.401171550854,-3.01189204818851));
#38945=CARTESIAN_POINT('Ctrl Pts',(-36.9179681053284,17.3991512563075,-2.5));
#38946=CARTESIAN_POINT('Ctrl Pts',(-37.4230703062887,17.4847366734944,-2.5));
#38947=CARTESIAN_POINT('Ctrl Pts',(-36.9260163611498,17.4267478207179,-3.0096623048872));
#38948=CARTESIAN_POINT('Ctrl Pts',(-36.9162547401427,17.4254293823291,-2.5));
#38949=CARTESIAN_POINT('Ctrl Pts',(-37.421584098594,17.4944468593896,-2.5));
#38950=CARTESIAN_POINT('Ctrl Pts',(-36.9205861826877,17.4783255467987,-3.0051277827859));
#38951=CARTESIAN_POINT('Ctrl Pts',(-36.91541973322,17.4779707405914,-2.5));
#38952=CARTESIAN_POINT('Ctrl Pts',(-37.4195477886376,17.5140317228638,-2.5));
#38953=CARTESIAN_POINT('Ctrl Pts',(-36.919118933325,17.5043343662994,-3.00282235189172));
#38954=CARTESIAN_POINT('Ctrl Pts',(-36.9162867050069,17.5042383112405,-2.5));
#38955=CARTESIAN_POINT('Ctrl Pts',(-37.4189975669682,17.5239091955899,-2.5));
#38956=CARTESIAN_POINT('Ctrl Pts',(-36.918942728626,17.5305480494939,-3.00047863991406));
#38957=CARTESIAN_POINT('Ctrl Pts',(-36.9184636408495,17.5305448701384,-2.5));
#38958=CARTESIAN_POINT('Ctrl Pts',(-37.418931489881,17.5338661095488,-2.5));
#38959=CARTESIAN_POINT('',(-38.0189154695161,17.5383073665604,-2.5));
#38960=CARTESIAN_POINT('Origin',(-38.0189152720306,17.538307365007,-3.));
#38961=CARTESIAN_POINT('',(-37.4189314692081,17.5338661094116,-2.5));
#38962=CARTESIAN_POINT('Ctrl Pts',(-37.4189314692081,17.5338661094116,-2.5));
#38963=CARTESIAN_POINT('Ctrl Pts',(-37.418924080912,17.5349752987399,-2.5));
#38964=CARTESIAN_POINT('Ctrl Pts',(-37.4189227173758,17.5360840623156,-2.5));
#38965=CARTESIAN_POINT('Ctrl Pts',(-37.418927375124,17.5371921369015,-2.50000000000001));
#38966=CARTESIAN_POINT('Ctrl Pts',(-37.4189482673457,17.5421623797679,-2.50000000000001));
#38967=CARTESIAN_POINT('Ctrl Pts',(-37.4190900906852,17.547112870658,-2.5));
#38968=CARTESIAN_POINT('Ctrl Pts',(-37.4193504503231,17.5520440628482,-2.5));
#38969=CARTESIAN_POINT('Ctrl Pts',(-37.4195528629438,17.5558777428411,-2.5));
#38970=CARTESIAN_POINT('Ctrl Pts',(-37.4198270040927,17.5596999384012,-2.5));
#38971=CARTESIAN_POINT('Ctrl Pts',(-37.4201718933211,17.5635102713167,-2.5));
#38972=CARTESIAN_POINT('Ctrl Pts',(-37.4207142534576,17.5695022609473,-2.5));
#38973=CARTESIAN_POINT('Ctrl Pts',(-37.4214316067083,17.5754659138134,-2.5));
#38974=CARTESIAN_POINT('Ctrl Pts',(-37.4223232424291,17.5814010980502,-2.5));
#38975=CARTESIAN_POINT('Ctrl Pts',(-37.4228904665252,17.5851768322829,-2.5));
#38976=CARTESIAN_POINT('Ctrl Pts',(-37.4235282497785,17.5889410563489,-2.5));
#38977=CARTESIAN_POINT('Ctrl Pts',(-37.424236403788,17.5926938015469,-2.5));
#38978=CARTESIAN_POINT('Ctrl Pts',(-37.4253492854007,17.5985913338245,-2.5));
#38979=CARTESIAN_POINT('Ctrl Pts',(-37.4266359441733,17.6044605190523,-2.5));
#38980=CARTESIAN_POINT('Ctrl Pts',(-37.4280987205395,17.610300986808,-2.5));
#38981=CARTESIAN_POINT('Ctrl Pts',(-37.4290298839969,17.6140188689625,-2.5));
#38982=CARTESIAN_POINT('Ctrl Pts',(-37.4300325085037,17.6177254059074,-2.5));
#38983=CARTESIAN_POINT('Ctrl Pts',(-37.4311069581255,17.6214196423252,-2.5));
#38984=CARTESIAN_POINT('Ctrl Pts',(-37.4314134572077,17.6224734656487,-2.5));
#38985=CARTESIAN_POINT('Ctrl Pts',(-37.4317258579008,17.6235264245972,-2.5));
#38986=CARTESIAN_POINT('Ctrl Pts',(-37.4320441492926,17.6245784015581,-2.5));
#38987=CARTESIAN_POINT('Ctrl Pts',(-37.4331601682326,17.628266927994,-2.5));
#38988=CARTESIAN_POINT('Ctrl Pts',(-37.4343492641677,17.6319454076607,-2.5));
#38989=CARTESIAN_POINT('Ctrl Pts',(-37.4356108634578,17.6356081256996,-2.5));
#38990=CARTESIAN_POINT('Ctrl Pts',(-37.4359704139135,17.6366519848316,-2.5));
#38991=CARTESIAN_POINT('Ctrl Pts',(-37.4363352907883,17.63769295271,-2.5));
#38992=CARTESIAN_POINT('Ctrl Pts',(-37.4367054529537,17.638730998124,-2.5));
#38993=CARTESIAN_POINT('Ctrl Pts',(-37.4380045061287,17.6423739317277,-2.5));
#38994=CARTESIAN_POINT('Ctrl Pts',(-37.4393688887006,17.6459815111093,-2.5));
#38995=CARTESIAN_POINT('Ctrl Pts',(-37.440797406153,17.6495538350512,-2.5));
#38996=CARTESIAN_POINT('Ctrl Pts',(-37.4467102048854,17.6643400964579,-2.5));
#38997=CARTESIAN_POINT('Ctrl Pts',(-37.4537132952356,17.6785310992158,-2.49999999999996));
#38998=CARTESIAN_POINT('Ctrl Pts',(-37.461799572854,17.6921314373255,-2.50000000000007));
#38999=CARTESIAN_POINT('Ctrl Pts',(-37.4637549480288,17.6954201895505,-2.5000000000001));
#39000=CARTESIAN_POINT('Ctrl Pts',(-37.4657735120508,17.6986739789099,-2.50000000000008));
#39001=CARTESIAN_POINT('Ctrl Pts',(-37.4678552376092,17.7018931471268,-2.50000000000005));
#39002=CARTESIAN_POINT('Ctrl Pts',(-37.4711178370673,17.706938411829,-2.50000000000001));
#39003=CARTESIAN_POINT('Ctrl Pts',(-37.4745386091628,17.7119005181788,-2.5));
#39004=CARTESIAN_POINT('Ctrl Pts',(-37.4781182518123,17.7167738292873,-2.5));
#39005=CARTESIAN_POINT('Ctrl Pts',(-37.4804030608609,17.7198843591383,-2.5));
#39006=CARTESIAN_POINT('Ctrl Pts',(-37.4827540352099,17.7229605353768,-2.49999999999995));
#39007=CARTESIAN_POINT('Ctrl Pts',(-37.4851688194139,17.725997596559,-2.50000000000007));
#39008=CARTESIAN_POINT('Ctrl Pts',(-37.4858526471977,17.7268576431063,-2.5000000000001));
#39009=CARTESIAN_POINT('Ctrl Pts',(-37.4865404402418,17.7277131251369,-2.50000000000015));
#39010=CARTESIAN_POINT('Ctrl Pts',(-37.4872321232356,17.728563994922,-2.50000000000025));
#39011=CARTESIAN_POINT('Ctrl Pts',(-37.4903663293432,17.7324195202151,-2.50000000000068));
#39012=CARTESIAN_POINT('Ctrl Pts',(-37.4935839883218,17.7361819881709,-2.5));
#39013=CARTESIAN_POINT('Ctrl Pts',(-37.4968822816754,17.7398546535842,-2.5));
#39014=CARTESIAN_POINT('Ctrl Pts',(-37.4994535903269,17.7427178180573,-2.5));
#39015=CARTESIAN_POINT('Ctrl Pts',(-37.5020742944106,17.7455259637112,-2.5));
#39016=CARTESIAN_POINT('Ctrl Pts',(-37.5047437562526,17.7482797483086,-2.5));
#39017=CARTESIAN_POINT('Ctrl Pts',(-37.5157710837796,17.7596554062098,-2.5));
#39018=CARTESIAN_POINT('Ctrl Pts',(-37.5276248076514,17.7701102809069,-2.5));
#39019=CARTESIAN_POINT('Ctrl Pts',(-37.5403203589352,17.7796263513267,-2.5));
#39020=CARTESIAN_POINT('Ctrl Pts',(-37.5433960495854,17.7819317643145,-2.5));
#39021=CARTESIAN_POINT('Ctrl Pts',(-37.5465218144476,17.7841825394691,-2.5));
#39022=CARTESIAN_POINT('Ctrl Pts',(-37.5496960494136,17.786377178086,-2.5));
#39023=CARTESIAN_POINT('Ctrl Pts',(-37.5505903348199,17.7869954792855,-2.5));
#39024=CARTESIAN_POINT('Ctrl Pts',(-37.5514888101488,17.787609476892,-2.5));
#39025=CARTESIAN_POINT('Ctrl Pts',(-37.5523912367608,17.7882189895587,-2.5));
#39026=CARTESIAN_POINT('Ctrl Pts',(-37.5555951317451,17.7903829489877,-2.5));
#39027=CARTESIAN_POINT('Ctrl Pts',(-37.5588532093185,17.7924931481196,-2.5));
#39028=CARTESIAN_POINT('Ctrl Pts',(-37.5621535646477,17.7945404310863,-2.5));
#39029=CARTESIAN_POINT('Ctrl Pts',(-37.5630823747426,17.7951165924074,-2.5));
#39030=CARTESIAN_POINT('Ctrl Pts',(-37.5640134395123,17.7956871178347,-2.5));
#39031=CARTESIAN_POINT('Ctrl Pts',(-37.564946673507,17.7962519914256,-2.5));
#39032=CARTESIAN_POINT('Ctrl Pts',(-37.5682633047709,17.7982595023205,-2.5));
#39033=CARTESIAN_POINT('Ctrl Pts',(-37.5716089097383,17.800196530261,-2.5));
#39034=CARTESIAN_POINT('Ctrl Pts',(-37.5749830496898,17.8020641498484,-2.5));
#39035=CARTESIAN_POINT('Ctrl Pts',(-37.5802548890879,17.8049821647094,-2.5));
#39036=CARTESIAN_POINT('Ctrl Pts',(-37.58559627027,17.8077310264052,-2.5));
#39037=CARTESIAN_POINT('Ctrl Pts',(-37.5910065014943,17.8103124473042,-2.5));
#39038=CARTESIAN_POINT('Ctrl Pts',(-37.5944705744368,17.8119652842937,-2.5));
#39039=CARTESIAN_POINT('Ctrl Pts',(-37.5979628694577,17.8135494693829,-2.5));
#39040=CARTESIAN_POINT('Ctrl Pts',(-37.6014832022656,17.8150654513137,-2.5));
#39041=CARTESIAN_POINT('Ctrl Pts',(-37.6105016362735,17.8189491133836,-2.5));
#39042=CARTESIAN_POINT('Ctrl Pts',(-37.6197040838036,17.8223851534601,-2.5));
#39043=CARTESIAN_POINT('Ctrl Pts',(-37.629092831199,17.8253680273689,-2.5));
#39044=CARTESIAN_POINT('Ctrl Pts',(-37.6337872059174,17.8268594646476,-2.5));
#39045=CARTESIAN_POINT('Ctrl Pts',(-37.6385282342954,17.8282374191786,-2.5));
#39046=CARTESIAN_POINT('Ctrl Pts',(-37.6433167322283,17.8294999097575,-2.5));
#39047=CARTESIAN_POINT('Ctrl Pts',(-37.644363925716,17.8297760029982,-2.5));
#39048=CARTESIAN_POINT('Ctrl Pts',(-37.6454133898735,17.8300465731124,-2.5));
#39049=CARTESIAN_POINT('Ctrl Pts',(-37.6464651365387,17.830311591346,-2.5));
#39050=CARTESIAN_POINT('Ctrl Pts',(-37.6478180462502,17.830652496389,-2.5));
#39051=CARTESIAN_POINT('Ctrl Pts',(-37.6491747302882,17.8309842382055,-2.5));
#39052=CARTESIAN_POINT('Ctrl Pts',(-37.6505352154912,17.8313067389472,-2.5));
#39053=CARTESIAN_POINT('Ctrl Pts',(-37.6529533369025,17.8318799505828,-2.50000000000001));
#39054=CARTESIAN_POINT('Ctrl Pts',(-37.6553864837853,17.8324245544573,-2.50000000000003));
#39055=CARTESIAN_POINT('Ctrl Pts',(-37.6578190611257,17.832936920446,-2.50000000000004));
#39056=CARTESIAN_POINT('Ctrl Pts',(-37.6588822778756,17.8331608623912,-2.50000000000004));
#39057=CARTESIAN_POINT('Ctrl Pts',(-37.6599457907485,17.8333788156395,-2.50000000000003));
#39058=CARTESIAN_POINT('Ctrl Pts',(-37.6610095988213,17.833590783111,-2.50000000000002));
#39059=CARTESIAN_POINT('Ctrl Pts',(-37.6658767167307,17.8345605733419,-2.49999999999998));
#39060=CARTESIAN_POINT('Ctrl Pts',(-37.6707498784643,17.8354056443311,-2.5));
#39061=CARTESIAN_POINT('Ctrl Pts',(-37.6756293102449,17.8361269204229,-2.5));
#39062=CARTESIAN_POINT('Ctrl Pts',(-37.6853881738059,17.8375694726066,-2.5));
#39063=CARTESIAN_POINT('Ctrl Pts',(-37.6951719386941,17.8385167826839,-2.49999999999996));
#39064=CARTESIAN_POINT('Ctrl Pts',(-37.7049796194108,17.8389772004795,-2.50000000000004));
#39065=CARTESIAN_POINT('Ctrl Pts',(-37.7088146288424,17.8391572335209,-2.50000000000008));
#39066=CARTESIAN_POINT('Ctrl Pts',(-37.7126533284138,17.8392626978782,-2.50000000000008));
#39067=CARTESIAN_POINT('Ctrl Pts',(-37.716495688883,17.8392941481056,-2.50000000000005));
#39068=CARTESIAN_POINT('Ctrl Pts',(-37.7224798087271,17.839343128916,-2.50000000000002));
#39069=CARTESIAN_POINT('Ctrl Pts',(-37.7284728705124,17.8392112724852,-2.5));
#39070=CARTESIAN_POINT('Ctrl Pts',(-37.7344750534382,17.8388957842887,-2.5));
#39071=CARTESIAN_POINT('Ctrl Pts',(-37.7383305288519,17.8386931318538,-2.5));
#39072=CARTESIAN_POINT('Ctrl Pts',(-37.7421906430535,17.8384145663926,-2.5));
#39073=CARTESIAN_POINT('Ctrl Pts',(-37.7460528064355,17.838059592336,-2.5));
#39074=CARTESIAN_POINT('Ctrl Pts',(-37.7471272624033,17.837960838359,-2.50000000000001));
#39075=CARTESIAN_POINT('Ctrl Pts',(-37.7482024838803,17.8378560565892,-2.50000000000001));
#39076=CARTESIAN_POINT('Ctrl Pts',(-37.7492777731307,17.8377453314094,-2.50000000000002));
#39077=CARTESIAN_POINT('Ctrl Pts',(-37.7531438406325,17.8373472329264,-2.50000000000005));
#39078=CARTESIAN_POINT('Ctrl Pts',(-37.757017212452,17.8368712456081,-2.50000000000001));
#39079=CARTESIAN_POINT('Ctrl Pts',(-37.7608631543582,17.8363214679065,-2.5));
#39080=CARTESIAN_POINT('Ctrl Pts',(-37.7619319418431,17.8361686846505,-2.5));
#39081=CARTESIAN_POINT('Ctrl Pts',(-37.7629989602928,17.8360102070827,-2.5));
#39082=CARTESIAN_POINT('Ctrl Pts',(-37.7640641141128,17.8358460852665,-2.5));
#39083=CARTESIAN_POINT('Ctrl Pts',(-37.7678975817809,17.835255414075,-2.5));
#39084=CARTESIAN_POINT('Ctrl Pts',(-37.7717092081801,17.8345911184888,-2.5));
#39085=CARTESIAN_POINT('Ctrl Pts',(-37.7754993148818,17.8338542984479,-2.5));
#39086=CARTESIAN_POINT('Ctrl Pts',(-37.79107968017,17.830825379662,-2.5));
#39087=CARTESIAN_POINT('Ctrl Pts',(-37.8062996088011,17.8265817597102,-2.49999999999996));
#39088=CARTESIAN_POINT('Ctrl Pts',(-37.8211596455932,17.8211262245503,-2.50000000000007));
#39089=CARTESIAN_POINT('Ctrl Pts',(-37.8247778021374,17.8197978980787,-2.5000000000001));
#39090=CARTESIAN_POINT('Ctrl Pts',(-37.8283738571345,17.8183979213105,-2.50000000000008));
#39091=CARTESIAN_POINT('Ctrl Pts',(-37.8319487721061,17.8169260699933,-2.50000000000006));
#39092=CARTESIAN_POINT('Ctrl Pts',(-37.836512836464,17.8150469695978,-2.50000000000003));
#39093=CARTESIAN_POINT('Ctrl Pts',(-37.8410421353742,17.8130496817546,-2.50000000000001));
#39094=CARTESIAN_POINT('Ctrl Pts',(-37.8455379349741,17.8109311783838,-2.50000000000002));
#39095=CARTESIAN_POINT('Ctrl Pts',(-37.8465112351386,17.8104725414643,-2.50000000000002));
#39096=CARTESIAN_POINT('Ctrl Pts',(-37.8474829057772,17.8100082029157,-2.50000000000002));
#39097=CARTESIAN_POINT('Ctrl Pts',(-37.8484524731366,17.8095384110422,-2.50000000000003));
#39098=CARTESIAN_POINT('Ctrl Pts',(-37.8519612366045,17.807838283096,-2.50000000000004));
#39099=CARTESIAN_POINT('Ctrl Pts',(-37.8554370944497,17.8060691333991,-2.50000000000001));
#39100=CARTESIAN_POINT('Ctrl Pts',(-37.8588613828517,17.8042413401211,-2.5));
#39101=CARTESIAN_POINT('Ctrl Pts',(-37.8598073158636,17.803736426458,-2.5));
#39102=CARTESIAN_POINT('Ctrl Pts',(-37.8607499173818,17.8032267705866,-2.5));
#39103=CARTESIAN_POINT('Ctrl Pts',(-37.8616892897569,17.8027123372952,-2.5));
#39104=CARTESIAN_POINT('Ctrl Pts',(-37.8660292009529,17.8003356495616,-2.5));
#39105=CARTESIAN_POINT('Ctrl Pts',(-37.8702969136781,17.7978586386703,-2.5));
#39106=CARTESIAN_POINT('Ctrl Pts',(-37.8744934438381,17.7952826854476,-2.5));
#39107=CARTESIAN_POINT('Ctrl Pts',(-37.8777830267203,17.7932634430489,-2.5));
#39108=CARTESIAN_POINT('Ctrl Pts',(-37.8810288717245,17.7911833904253,-2.5));
#39109=CARTESIAN_POINT('Ctrl Pts',(-37.8842314572436,17.7890432104997,-2.5));
#39110=CARTESIAN_POINT('Ctrl Pts',(-37.8973710612388,17.780262456158,-2.5));
#39111=CARTESIAN_POINT('Ctrl Pts',(-37.909787707558,17.770476851842,-2.5));
#39112=CARTESIAN_POINT('Ctrl Pts',(-37.9214627815581,17.7596617340041,-2.5));
#39113=CARTESIAN_POINT('Ctrl Pts',(-37.9243104333541,17.7570238329738,-2.5));
#39114=CARTESIAN_POINT('Ctrl Pts',(-37.9271138062512,17.7543248652812,-2.49999999999999));
#39115=CARTESIAN_POINT('Ctrl Pts',(-37.9298738983267,17.7515632530563,-2.5));
#39116=CARTESIAN_POINT('Ctrl Pts',(-37.9306323609192,17.7508043727326,-2.50000000000001));
#39117=CARTESIAN_POINT('Ctrl Pts',(-37.9313866370695,17.7500415820386,-2.50000000000001));
#39118=CARTESIAN_POINT('Ctrl Pts',(-37.9321366200852,17.7492750237347,-2.50000000000002));
#39119=CARTESIAN_POINT('Ctrl Pts',(-37.9348664680114,17.7464848437543,-2.50000000000006));
#39120=CARTESIAN_POINT('Ctrl Pts',(-37.9375346700091,17.7436492082643,-2.50000000000001));
#39121=CARTESIAN_POINT('Ctrl Pts',(-37.9401394064799,17.7407723818853,-2.5));
#39122=CARTESIAN_POINT('Ctrl Pts',(-37.9408544316472,17.7399826654261,-2.5));
#39123=CARTESIAN_POINT('Ctrl Pts',(-37.9415648944728,17.7391896173097,-2.5));
#39124=CARTESIAN_POINT('Ctrl Pts',(-37.9422708937099,17.7383931600166,-2.5));
#39125=CARTESIAN_POINT('Ctrl Pts',(-37.9448433738321,17.735491073942,-2.5));
#39126=CARTESIAN_POINT('Ctrl Pts',(-37.9473544995132,17.7325458015199,-2.5));
#39127=CARTESIAN_POINT('Ctrl Pts',(-37.9498050507074,17.7295578914628,-2.5));
#39128=CARTESIAN_POINT('Ctrl Pts',(-37.953599486724,17.7249314084242,-2.5));
#39129=CARTESIAN_POINT('Ctrl Pts',(-37.9572489362766,17.720202871343,-2.5));
#39130=CARTESIAN_POINT('Ctrl Pts',(-37.9607543179931,17.7153729233453,-2.5));
#39131=CARTESIAN_POINT('Ctrl Pts',(-37.963019073585,17.7122523925099,-2.5));
#39132=CARTESIAN_POINT('Ctrl Pts',(-37.9652236695998,17.7090895187778,-2.5));
#39133=CARTESIAN_POINT('Ctrl Pts',(-37.9673683607455,17.7058844804642,-2.5));
#39134=CARTESIAN_POINT('Ctrl Pts',(-37.9706870703085,17.7009249825326,-2.5));
#39135=CARTESIAN_POINT('Ctrl Pts',(-37.9738623463162,17.6958645281885,-2.5));
#39136=CARTESIAN_POINT('Ctrl Pts',(-37.9768926058306,17.6907019898296,-2.5));
#39137=CARTESIAN_POINT('Ctrl Pts',(-37.9788516386036,17.6873644598956,-2.5));
#39138=CARTESIAN_POINT('Ctrl Pts',(-37.9807502945889,17.6839838181975,-2.5));
#39139=CARTESIAN_POINT('Ctrl Pts',(-37.9825874564246,17.6805610345249,-2.5));
#39140=CARTESIAN_POINT('Ctrl Pts',(-37.983089397607,17.6796258767994,-2.5));
#39141=CARTESIAN_POINT('Ctrl Pts',(-37.9835868344571,17.6786873721866,-2.5));
#39142=CARTESIAN_POINT('Ctrl Pts',(-37.9840796736073,17.6777456651142,-2.5));
#39143=CARTESIAN_POINT('Ctrl Pts',(-37.9858839189027,17.6742981497245,-2.5));
#39144=CARTESIAN_POINT('Ctrl Pts',(-37.9876280092296,17.6708047329094,-2.5));
#39145=CARTESIAN_POINT('Ctrl Pts',(-37.9893067995452,17.6672733142509,-2.5));
#39146=CARTESIAN_POINT('Ctrl Pts',(-37.9897649997402,17.6663094674242,-2.5));
#39147=CARTESIAN_POINT('Ctrl Pts',(-37.9902177317802,17.6653440883829,-2.5));
#39148=CARTESIAN_POINT('Ctrl Pts',(-37.9906650024386,17.6643772306817,-2.5));
#39149=CARTESIAN_POINT('Ctrl Pts',(-37.9923040383024,17.6608341535369,-2.5));
#39150=CARTESIAN_POINT('Ctrl Pts',(-37.9938701991613,17.6572701642616,-2.5));
#39151=CARTESIAN_POINT('Ctrl Pts',(-37.9953647259209,17.6536856269683,-2.5));
#39152=CARTESIAN_POINT('Ctrl Pts',(-38.0014785926123,17.6390218660013,-2.5));
#39153=CARTESIAN_POINT('Ctrl Pts',(-38.00640415232,17.6240172077284,-2.49999999999996));
#39154=CARTESIAN_POINT('Ctrl Pts',(-38.0101545839031,17.6086755353485,-2.50000000000007));
#39155=CARTESIAN_POINT('Ctrl Pts',(-38.011072015426,17.6049226515687,-2.50000000000009));
#39156=CARTESIAN_POINT('Ctrl Pts',(-38.0119191589871,17.6011490664917,-2.50000000000008));
#39157=CARTESIAN_POINT('Ctrl Pts',(-38.0126960956751,17.5973554922411,-2.50000000000005));
#39158=CARTESIAN_POINT('Ctrl Pts',(-38.0136844102185,17.5925298164031,-2.50000000000002));
#39159=CARTESIAN_POINT('Ctrl Pts',(-38.0145581006726,17.5876715036185,-2.5));
#39160=CARTESIAN_POINT('Ctrl Pts',(-38.0153154860037,17.5827814680338,-2.5));
#39161=CARTESIAN_POINT('Ctrl Pts',(-38.015477177083,17.5817375144489,-2.5));
#39162=CARTESIAN_POINT('Ctrl Pts',(-38.0156336037888,17.5806917722016,-2.5));
#39163=CARTESIAN_POINT('Ctrl Pts',(-38.0157847183714,17.5796444881076,-2.5));
#39164=CARTESIAN_POINT('Ctrl Pts',(-38.0163414467211,17.5757861394604,-2.50000000000001));
#39165=CARTESIAN_POINT('Ctrl Pts',(-38.0168265261798,17.5719026151513,-2.5));
#39166=CARTESIAN_POINT('Ctrl Pts',(-38.0172369355354,17.5680093665256,-2.5));
#39167=CARTESIAN_POINT('Ctrl Pts',(-38.0173482325746,17.5669535742082,-2.5));
#39168=CARTESIAN_POINT('Ctrl Pts',(-38.0174539918432,17.5658978049004,-2.50000000000001));
#39169=CARTESIAN_POINT('Ctrl Pts',(-38.0175542183555,17.5648421351762,-2.50000000000001));
#39170=CARTESIAN_POINT('Ctrl Pts',(-38.0180240315044,17.5598936688902,-2.50000000000001));
#39171=CARTESIAN_POINT('Ctrl Pts',(-38.0183723928837,17.5549445094189,-2.5));
#39172=CARTESIAN_POINT('Ctrl Pts',(-38.0186003857153,17.5499946296404,-2.5));
#39173=CARTESIAN_POINT('Ctrl Pts',(-38.0187798053734,17.5460993065656,-2.5));
#39174=CARTESIAN_POINT('Ctrl Pts',(-38.0188847752909,17.5422035509477,-2.50000000000002));
#39175=CARTESIAN_POINT('Ctrl Pts',(-38.0189154695161,17.5383073665604,-2.50000000000004));
#39176=CARTESIAN_POINT('Origin',(-37.418931489881,17.5338661095487,-2.99999999999999));
#39177=CARTESIAN_POINT('Origin',(-37.718924746634,25.7501158975689,-1.15479289890034));
#39178=CARTESIAN_POINT('',(-37.718924746634,25.0506850112887,-0.766467731910881));
#39179=CARTESIAN_POINT('Origin',(-17.718924746634,24.9242463227439,7.77478435608303));
#39180=CARTESIAN_POINT('',(-17.718924746634,24.1393970581951,7.61982748486642));
#39181=CARTESIAN_POINT('Origin',(-17.718924746634,17.0757536772561,6.22521564391699));
#39182=CARTESIAN_POINT('Ctrl Pts',(-18.0133068931633,17.0493818775115,6.22000892238259));
#39183=CARTESIAN_POINT('Ctrl Pts',(-18.0151995259403,17.0589094855094,6.2218900075713));
#39184=CARTESIAN_POINT('Ctrl Pts',(-18.0166154517927,17.0685214343805,6.22378774460121));
#39185=CARTESIAN_POINT('Ctrl Pts',(-18.0175568383944,17.0782373050469,6.22570599946563));
#39186=CARTESIAN_POINT('Ctrl Pts',(-18.0176064793518,17.0787496398519,6.22580715239014));
#39187=CARTESIAN_POINT('Ctrl Pts',(-18.0176547742521,17.079262076957,6.22590832551228));
#39188=CARTESIAN_POINT('Ctrl Pts',(-18.0177017242961,17.0797745926913,6.22600951415857));
#39189=CARTESIAN_POINT('Ctrl Pts',(-18.0180997249336,17.0841192443959,6.22686730133517));
#39190=CARTESIAN_POINT('Ctrl Pts',(-18.0183999920715,17.0884652630194,6.22772535838965));
#39191=CARTESIAN_POINT('Ctrl Pts',(-18.0186030723344,17.0927970021125,6.22858059616219));
#39192=CARTESIAN_POINT('Ctrl Pts',(-18.0188302270038,17.0976422526911,6.22953721917737));
#39193=CARTESIAN_POINT('Ctrl Pts',(-18.0189364808522,17.1024766655667,6.2304917024485));
#39194=CARTESIAN_POINT('Ctrl Pts',(-18.0189238263079,17.1073011345983,6.23144422245482));
#39195=CARTESIAN_POINT('Ctrl Pts',(-18.0188971857286,17.1174576955315,6.23344948509009));
#39196=CARTESIAN_POINT('Ctrl Pts',(-18.0183483687477,17.1275705647777,6.23544612144843));
#39197=CARTESIAN_POINT('Ctrl Pts',(-18.0172736561345,17.1376463417085,6.23743543447808));
#39198=CARTESIAN_POINT('Ctrl Pts',(-18.0163062039052,17.1467165179889,6.23922620654257));
#39199=CARTESIAN_POINT('Ctrl Pts',(-18.0149127944694,17.1557527788852,6.24101028251644));
#39200=CARTESIAN_POINT('Ctrl Pts',(-18.0130910712219,17.164755336083,6.24278770419385));
#39201=CARTESIAN_POINT('Ctrl Pts',(-18.0129906098694,17.1652517940787,6.24288572247734));
#39202=CARTESIAN_POINT('Ctrl Pts',(-18.012888834453,17.1657481486638,6.24298372034392));
#39203=CARTESIAN_POINT('Ctrl Pts',(-18.0127857420086,17.1662443996692,6.24308169776025));
#39204=CARTESIAN_POINT('Ctrl Pts',(-18.0119023898804,17.1704965481556,6.24392122154546));
#39205=CARTESIAN_POINT('Ctrl Pts',(-18.01092307448,17.1747382382048,6.24475868046705));
#39206=CARTESIAN_POINT('Ctrl Pts',(-18.0098438883496,17.1789775150786,6.24559566294285));
#39207=CARTESIAN_POINT('Ctrl Pts',(-18.0097181622568,17.1794713944035,6.24569317210597));
#39208=CARTESIAN_POINT('Ctrl Pts',(-18.0095911499154,17.1799649488279,6.24579061712228));
#39209=CARTESIAN_POINT('Ctrl Pts',(-18.0094628549034,17.1804581707779,6.24588799649643));
#39210=CARTESIAN_POINT('Ctrl Pts',(-18.0083614518184,17.184692444338,6.246723991142));
#39211=CARTESIAN_POINT('Ctrl Pts',(-18.0071692721591,17.1888882609517,6.2475523930327));
#39212=CARTESIAN_POINT('Ctrl Pts',(-18.005888759018,17.1930435737714,6.24837279804873));
#39213=CARTESIAN_POINT('Ctrl Pts',(-18.005739794034,17.1935269706909,6.24846823761601));
#39214=CARTESIAN_POINT('Ctrl Pts',(-18.0055896174112,17.1940098841075,6.24856358172282));
#39215=CARTESIAN_POINT('Ctrl Pts',(-18.0054382246546,17.1944923306919,6.24865883366051));
#39216=CARTESIAN_POINT('Ctrl Pts',(-18.0026835667137,17.2032706589575,6.25039198465394));
#39217=CARTESIAN_POINT('Ctrl Pts',(-17.9995320635773,17.2118760854732,6.25209099875588));
#39218=CARTESIAN_POINT('Ctrl Pts',(-17.9959915059306,17.2203120171548,6.2537565486114));
#39219=CARTESIAN_POINT('Ctrl Pts',(-17.9920630646076,17.2296721422883,6.2556045667856));
#39220=CARTESIAN_POINT('Ctrl Pts',(-17.9876590484585,17.2388253614501,6.25741173443796));
#39221=CARTESIAN_POINT('Ctrl Pts',(-17.9827682254716,17.2477663515645,6.25917700060597));
#39222=CARTESIAN_POINT('Ctrl Pts',(-17.978358783995,17.2558273205992,6.26076851963648));
#39223=CARTESIAN_POINT('Ctrl Pts',(-17.9735560484698,17.263712298677,6.26232529185723));
#39224=CARTESIAN_POINT('Ctrl Pts',(-17.9683445575794,17.2714279183298,6.26384862676358));
#39225=CARTESIAN_POINT('Ctrl Pts',(-17.9680609879744,17.2718477435321,6.2639315150362));
#39226=CARTESIAN_POINT('Ctrl Pts',(-17.9677764219516,17.272266728987,6.26401423751312));
#39227=CARTESIAN_POINT('Ctrl Pts',(-17.9674908612731,17.2726848753105,6.26409679431597));
#39228=CARTESIAN_POINT('Ctrl Pts',(-17.962241876116,17.2803709610012,6.26561429817859));
#39229=CARTESIAN_POINT('Ctrl Pts',(-17.9566686125952,17.287757411178,6.26707264344373));
#39230=CARTESIAN_POINT('Ctrl Pts',(-17.9507822138997,17.2948520727703,6.26847337937143));
#39231=CARTESIAN_POINT('Ctrl Pts',(-17.9504629875019,17.2952368247013,6.26854934294571));
#39232=CARTESIAN_POINT('Ctrl Pts',(-17.9501428289144,17.295620732202,6.26862513979976));
#39233=CARTESIAN_POINT('Ctrl Pts',(-17.9498217365886,17.2960037971992,6.26870077031396));
#39234=CARTESIAN_POINT('Ctrl Pts',(-17.9439000104084,17.3030684506987,6.27009558158786));
#39235=CARTESIAN_POINT('Ctrl Pts',(-17.9376641923768,17.3098425498617,6.27143302720835));
#39236=CARTESIAN_POINT('Ctrl Pts',(-17.9311160363576,17.3163270111148,6.27271328811027));
#39237=CARTESIAN_POINT('Ctrl Pts',(-17.9242125826885,17.3231633139913,6.27406301493335));
#39238=CARTESIAN_POINT('Ctrl Pts',(-17.9169620149873,17.3296777303634,6.27534919003014));
#39239=CARTESIAN_POINT('Ctrl Pts',(-17.9093564103244,17.3358620845237,6.27657019922831));
#39240=CARTESIAN_POINT('Ctrl Pts',(-17.9089677439614,17.3361781212552,6.27663259600348));
#39241=CARTESIAN_POINT('Ctrl Pts',(-17.9085781282527,17.33649330971,6.27669482529897));
#39242=CARTESIAN_POINT('Ctrl Pts',(-17.9081875674216,17.3368076431069,6.27675688577594));
#39243=CARTESIAN_POINT('Ctrl Pts',(-17.9047568553611,17.3395687683655,6.27730202909254));
#39244=CARTESIAN_POINT('Ctrl Pts',(-17.9012526549201,17.3422643567528,6.27783423312387));
#39245=CARTESIAN_POINT('Ctrl Pts',(-17.8976780873748,17.3448896272997,6.27835255393837));
#39246=CARTESIAN_POINT('Ctrl Pts',(-17.8972718062779,17.3451880124286,6.27841146566585));
#39247=CARTESIAN_POINT('Ctrl Pts',(-17.8968649183223,17.3454852683764,6.27847015445325));
#39248=CARTESIAN_POINT('Ctrl Pts',(-17.8964574268529,17.3457813960457,6.27852862047875));
#39249=CARTESIAN_POINT('Ctrl Pts',(-17.8928715423093,17.3483872901855,6.27904311570846));
#39250=CARTESIAN_POINT('Ctrl Pts',(-17.8892395463305,17.3509051559847,6.27954023104512));
#39251=CARTESIAN_POINT('Ctrl Pts',(-17.8855625443911,17.3533364734939,6.28002025870288));
#39252=CARTESIAN_POINT('Ctrl Pts',(-17.8851453833495,17.3536123098849,6.28007471851579));
#39253=CARTESIAN_POINT('Ctrl Pts',(-17.8847276428159,17.3538870458274,6.28012896106144));
#39254=CARTESIAN_POINT('Ctrl Pts',(-17.884309321612,17.3541606824097,6.28018298655469));
#39255=CARTESIAN_POINT('Ctrl Pts',(-17.8760982231813,17.3595318108423,6.28124343636894));
#39256=CARTESIAN_POINT('Ctrl Pts',(-17.8676653792537,17.3644784082662,6.28222006881877));
#39257=CARTESIAN_POINT('Ctrl Pts',(-17.8590112984533,17.3690021459286,6.28311321386716));
#39258=CARTESIAN_POINT('Ctrl Pts',(-17.8507952450643,17.373296914028,6.28396115226419));
#39259=CARTESIAN_POINT('Ctrl Pts',(-17.8423802671056,17.3772106561903,6.28473386272934));
#39260=CARTESIAN_POINT('Ctrl Pts',(-17.8337665264467,17.3807441488957,6.28543149856692));
#39261=CARTESIAN_POINT('Ctrl Pts',(-17.8333072968939,17.3809325321242,6.28546869204724));
#39262=CARTESIAN_POINT('Ctrl Pts',(-17.8328474973904,17.3811198248295,6.2855056702199));
#39263=CARTESIAN_POINT('Ctrl Pts',(-17.8323871269169,17.3813060250783,6.28554243270319));
#39264=CARTESIAN_POINT('Ctrl Pts',(-17.8282990371385,17.382959483277,6.28586888355269));
#39265=CARTESIAN_POINT('Ctrl Pts',(-17.8241650495164,17.3845273373272,6.28617843313006));
#39266=CARTESIAN_POINT('Ctrl Pts',(-17.8199872841232,17.3860072533335,6.28647062064218));
#39267=CARTESIAN_POINT('Ctrl Pts',(-17.819517535096,17.3861736554741,6.28650347428202));
#39268=CARTESIAN_POINT('Ctrl Pts',(-17.8190471432221,17.3863389729831,6.28653611377741));
#39269=CARTESIAN_POINT('Ctrl Pts',(-17.8185761407676,17.3865031933171,6.28656853665184));
#39270=CARTESIAN_POINT('Ctrl Pts',(-17.8143864015698,17.3879639932853,6.28685694998517));
#39271=CARTESIAN_POINT('Ctrl Pts',(-17.8101435756898,17.3893394993071,6.28712852329117));
#39272=CARTESIAN_POINT('Ctrl Pts',(-17.8058709862739,17.3906204723322,6.28738143245607));
#39273=CARTESIAN_POINT('Ctrl Pts',(-17.8053915126047,17.3907642242298,6.28740981414068));
#39274=CARTESIAN_POINT('Ctrl Pts',(-17.8049118810369,17.3909067288397,6.28743794956678));
#39275=CARTESIAN_POINT('Ctrl Pts',(-17.8044320969961,17.3910479869729,6.2874658388945));
#39276=CARTESIAN_POINT('Ctrl Pts',(-17.7954000423655,17.3937072066784,6.28799086246787));
#39277=CARTESIAN_POINT('Ctrl Pts',(-17.78630765222,17.3959264977103,6.28842902863579));
#39278=CARTESIAN_POINT('Ctrl Pts',(-17.7771567393255,17.397719289795,6.2887829888989));
#39279=CARTESIAN_POINT('Ctrl Pts',(-17.7670367925117,17.3997019292053,6.28917443170665));
#39280=CARTESIAN_POINT('Ctrl Pts',(-17.7568457798152,17.4011666604281,6.289463621208));
#39281=CARTESIAN_POINT('Ctrl Pts',(-17.7465828115781,17.4021072682102,6.28964933029322));
#39282=CARTESIAN_POINT('Ctrl Pts',(-17.7372993592615,17.4029581027146,6.28981731497344));
#39283=CARTESIAN_POINT('Ctrl Pts',(-17.7279574142293,17.4033800700187,6.28990062617237));
#39284=CARTESIAN_POINT('Ctrl Pts',(-17.7185558210734,17.4033686132305,6.2898983641991));
#39285=CARTESIAN_POINT('Ctrl Pts',(-17.7180614574138,17.4033680107986,6.28989824525784));
#39286=CARTESIAN_POINT('Ctrl Pts',(-17.7175669272791,17.4033661986565,6.28989788747721));
#39287=CARTESIAN_POINT('Ctrl Pts',(-17.7170722302065,17.4033631739899,6.28989729030154));
#39288=CARTESIAN_POINT('Ctrl Pts',(-17.7150908610137,17.4033510595431,6.28989489848333));
#39289=CARTESIAN_POINT('Ctrl Pts',(-17.713106823896,17.4033194963692,6.28988866680177));
#39290=CARTESIAN_POINT('Ctrl Pts',(-17.7111200943939,17.4032683024772,6.28987855932548));
#39291=CARTESIAN_POINT('Ctrl Pts',(-17.7086373297241,17.4032043267893,6.28986592827277));
#39292=CARTESIAN_POINT('Ctrl Pts',(-17.7061493206867,17.4031095514149,6.28984721627779));
#39293=CARTESIAN_POINT('Ctrl Pts',(-17.7036711651943,17.4029846303786,6.28982255246806));
#39294=CARTESIAN_POINT('Ctrl Pts',(-17.7031768681837,17.4029597134212,6.2898176329836));
#39295=CARTESIAN_POINT('Ctrl Pts',(-17.7026828252418,17.4029335955226,6.28981247639108));
#39296=CARTESIAN_POINT('Ctrl Pts',(-17.7021890358816,17.4029062789949,6.28980708314698));
#39297=CARTESIAN_POINT('Ctrl Pts',(-17.6977316048652,17.4026596930054,6.28975839839293));
#39298=CARTESIAN_POINT('Ctrl Pts',(-17.6932948233157,17.4023154871287,6.28969044003697));
#39299=CARTESIAN_POINT('Ctrl Pts',(-17.6888783478203,17.4018753094736,6.28960353347377));
#39300=CARTESIAN_POINT('Ctrl Pts',(-17.688389904011,17.4018266276569,6.28959392196956));
#39301=CARTESIAN_POINT('Ctrl Pts',(-17.6879017081709,17.4017767739381,6.28958407909064));
#39302=CARTESIAN_POINT('Ctrl Pts',(-17.6874137601304,17.4017257492013,6.28957400501155));
#39303=CARTESIAN_POINT('Ctrl Pts',(-17.6781002074841,17.4007518308069,6.28938171923894));
#39304=CARTESIAN_POINT('Ctrl Pts',(-17.66887685941,17.3993514864911,6.28910524197941));
#39305=CARTESIAN_POINT('Ctrl Pts',(-17.6597422801017,17.397531513091,6.28874591516785));
#39306=CARTESIAN_POINT('Ctrl Pts',(-17.6501291359109,17.3956161904332,6.28836776305657));
#39307=CARTESIAN_POINT('Ctrl Pts',(-17.6406143081556,17.3932361045023,6.28789785031569));
#39308=CARTESIAN_POINT('Ctrl Pts',(-17.6311990050655,17.3903855899544,6.28733505840692));
#39309=CARTESIAN_POINT('Ctrl Pts',(-17.6307333868561,17.3902446224819,6.28730722646584));
#39310=CARTESIAN_POINT('Ctrl Pts',(-17.6302680124599,17.3901025025716,6.28727916699298));
#39311=CARTESIAN_POINT('Ctrl Pts',(-17.6298028822972,17.3899592282443,6.28725087959758));
#39312=CARTESIAN_POINT('Ctrl Pts',(-17.6255653243114,17.3886539306776,6.28699316791192));
#39313=CARTESIAN_POINT('Ctrl Pts',(-17.6213472115623,17.3872525326915,6.2867164826208));
#39314=CARTESIAN_POINT('Ctrl Pts',(-17.6171512211235,17.3857544345316,6.28642070531156));
#39315=CARTESIAN_POINT('Ctrl Pts',(-17.6166913908926,17.3855902609395,6.28638829166563));
#39316=CARTESIAN_POINT('Ctrl Pts',(-17.6162317405224,17.3854248853256,6.2863556406983));
#39317=CARTESIAN_POINT('Ctrl Pts',(-17.6157723292095,17.3852583310309,6.28632275701788));
#39318=CARTESIAN_POINT('Ctrl Pts',(-17.611579352614,17.3837382155269,6.28602263270991));
#39319=CARTESIAN_POINT('Ctrl Pts',(-17.6074023369311,17.3821183117921,6.28570280669268));
#39320=CARTESIAN_POINT('Ctrl Pts',(-17.6032870770419,17.380416304936,6.28536677062928));
#39321=CARTESIAN_POINT('Ctrl Pts',(-17.6028369747322,17.38023014969,6.28533001703112));
#39322=CARTESIAN_POINT('Ctrl Pts',(-17.6023875004942,17.3800429894745,6.28529306501661));
#39323=CARTESIAN_POINT('Ctrl Pts',(-17.6019386577086,17.379854826811,6.28525591508357));
#39324=CARTESIAN_POINT('Ctrl Pts',(-17.5928334838723,17.3760377803621,6.28450229575596));
#39325=CARTESIAN_POINT('Ctrl Pts',(-17.5839822725707,17.3718062598322,6.28366684465546));
#39326=CARTESIAN_POINT('Ctrl Pts',(-17.5753808547761,17.3671661414509,6.28275072195659));
#39327=CARTESIAN_POINT('Ctrl Pts',(-17.5672010821262,17.3627534836386,6.28187950798057));
#39328=CARTESIAN_POINT('Ctrl Pts',(-17.5592466988203,17.3579709628613,6.28093527003623));
#39329=CARTESIAN_POINT('Ctrl Pts',(-17.551515652032,17.3528245952513,6.27991919591984));
#39330=CARTESIAN_POINT('Ctrl Pts',(-17.54338434228,17.3474117824355,6.27885051614107));
#39331=CARTESIAN_POINT('Ctrl Pts',(-17.5355018854376,17.3415935456519,6.27770179140026));
#39332=CARTESIAN_POINT('Ctrl Pts',(-17.527876561236,17.3353594564721,6.27647096275861));
#39333=CARTESIAN_POINT('Ctrl Pts',(-17.527504484612,17.3350552649658,6.27641090464783));
#39334=CARTESIAN_POINT('Ctrl Pts',(-17.5271329362737,17.3347500052773,6.27635063564029));
#39335=CARTESIAN_POINT('Ctrl Pts',(-17.5267620036043,17.3344437506483,6.27629017019649));
#39336=CARTESIAN_POINT('Ctrl Pts',(-17.5252323697242,17.3331808328872,6.27604082577622));
#39337=CARTESIAN_POINT('Ctrl Pts',(-17.5237128212741,17.3319006630474,6.27578807518837));
#39338=CARTESIAN_POINT('Ctrl Pts',(-17.5222096817844,17.3306085300547,6.27553296265302));
#39339=CARTESIAN_POINT('Ctrl Pts',(-17.5203423804563,17.329003355239,6.27521604464285));
#39340=CARTESIAN_POINT('Ctrl Pts',(-17.5184987822701,17.3273784795521,6.27489523698725));
#39341=CARTESIAN_POINT('Ctrl Pts',(-17.5166789587972,17.3257344763096,6.2745706528789));
#39342=CARTESIAN_POINT('Ctrl Pts',(-17.5163243493235,17.3254141270376,6.27450740465644));
#39343=CARTESIAN_POINT('Ctrl Pts',(-17.5159706422872,17.3250930517187,6.27444401308677));
#39344=CARTESIAN_POINT('Ctrl Pts',(-17.5156178386202,17.3247712542517,6.27438047893964));
#39345=CARTESIAN_POINT('Ctrl Pts',(-17.5123492315953,17.3217899092154,6.2737918564873));
#39346=CARTESIAN_POINT('Ctrl Pts',(-17.5091574796189,17.3187456886125,6.27319082018488));
#39347=CARTESIAN_POINT('Ctrl Pts',(-17.5060413667377,17.3156395916544,6.2725775673119));
#39348=CARTESIAN_POINT('Ctrl Pts',(-17.5057055852483,17.3153048894461,6.27251148531459));
#39349=CARTESIAN_POINT('Ctrl Pts',(-17.5053706742823,17.3149694751014,6.2724452627165));
#39350=CARTESIAN_POINT('Ctrl Pts',(-17.50503663389,17.3146333485789,6.27237889950942));
#39351=CARTESIAN_POINT('Ctrl Pts',(-17.4981686427345,17.3077224658295,6.27101444799423));
#39352=CARTESIAN_POINT('Ctrl Pts',(-17.4916683867703,17.3005107152883,6.26959059458653));
#39353=CARTESIAN_POINT('Ctrl Pts',(-17.4855366603079,17.2929973081219,6.26810718354282));
#39354=CARTESIAN_POINT('Ctrl Pts',(-17.4797011422079,17.2858468548555,6.26669543237481));
#39355=CARTESIAN_POINT('Ctrl Pts',(-17.4741996148819,17.2784234803524,6.26522979694795));
#39356=CARTESIAN_POINT('Ctrl Pts',(-17.4690325144084,17.2707263188011,6.26371010632058));
#39357=CARTESIAN_POINT('Ctrl Pts',(-17.4687702346341,17.2703356142262,6.26363296748483));
#39358=CARTESIAN_POINT('Ctrl Pts',(-17.468508824208,17.2699441979455,6.26355568813333));
#39359=CARTESIAN_POINT('Ctrl Pts',(-17.4682482847578,17.2695520685622,6.26347826799026));
#39360=CARTESIAN_POINT('Ctrl Pts',(-17.4658117031665,17.2658848495045,6.26275422986355));
#39361=CARTESIAN_POINT('Ctrl Pts',(-17.4634512948009,17.2621553054514,6.26201788658893));
#39362=CARTESIAN_POINT('Ctrl Pts',(-17.4611684259367,17.2583623237431,6.2612690184882));
#39363=CARTESIAN_POINT('Ctrl Pts',(-17.458641452522,17.2541637628493,6.26044007478003));
#39364=CARTESIAN_POINT('Ctrl Pts',(-17.4562225545235,17.2499084715741,6.2595999304977));
#39365=CARTESIAN_POINT('Ctrl Pts',(-17.453921204761,17.2456173631331,6.25875271464607));
#39366=CARTESIAN_POINT('Ctrl Pts',(-17.4536996553159,17.2452042609139,6.25867115372695));
#39367=CARTESIAN_POINT('Ctrl Pts',(-17.4534791583449,17.2447907694999,6.25858951596709));
#39368=CARTESIAN_POINT('Ctrl Pts',(-17.453259712687,17.2443768893244,6.25850780145202));
#39369=CARTESIAN_POINT('Ctrl Pts',(-17.4489201906875,17.2361924388161,6.25689190283213));
#39370=CARTESIAN_POINT('Ctrl Pts',(-17.4449915782234,17.22785591363,6.25524597931787));
#39371=CARTESIAN_POINT('Ctrl Pts',(-17.4414648184729,17.2193708249878,6.25357072414803));
#39372=CARTESIAN_POINT('Ctrl Pts',(-17.4377596760485,17.2104565625692,6.25181073496798));
#39373=CARTESIAN_POINT('Ctrl Pts',(-17.434498115918,17.2013783091928,6.25001836820042));
#39374=CARTESIAN_POINT('Ctrl Pts',(-17.4316824779197,17.1921354103922,6.24819349463067));
#39375=CARTESIAN_POINT('Ctrl Pts',(-17.4315478755021,17.1916935508474,6.24810625600323));
#39376=CARTESIAN_POINT('Ctrl Pts',(-17.431414290673,17.1912513087585,6.24801894184813));
#39377=CARTESIAN_POINT('Ctrl Pts',(-17.4312817253082,17.1908086844359,6.24793155222665));
#39378=CARTESIAN_POINT('Ctrl Pts',(-17.4298954472664,17.1861800215884,6.24701769125339));
#39379=CARTESIAN_POINT('Ctrl Pts',(-17.4286207447609,17.1815100802888,6.24609568046068));
#39380=CARTESIAN_POINT('Ctrl Pts',(-17.4274595038986,17.1767981983333,6.24516538910623));
#39381=CARTESIAN_POINT('Ctrl Pts',(-17.4264089791608,17.1725355610832,6.24432379446985));
#39382=CARTESIAN_POINT('Ctrl Pts',(-17.4254503111968,17.1682336230582,6.24347444047714));
#39383=CARTESIAN_POINT('Ctrl Pts',(-17.4245878781802,17.16390605946,6.24262002709426));
#39384=CARTESIAN_POINT('Ctrl Pts',(-36.918942728626,17.5305480494939,-3.00047863991406));
#39385=CARTESIAN_POINT('Ctrl Pts',(-36.9184636408495,17.5305448701384,-2.5));
#39386=CARTESIAN_POINT('Ctrl Pts',(-37.418931489881,17.5338661095488,-2.5));
#39387=CARTESIAN_POINT('Ctrl Pts',(-36.918766523927,17.5567617326884,-2.99813492793641));
#39388=CARTESIAN_POINT('Ctrl Pts',(-36.9206303865991,17.5567282897711,-2.5));
#39389=CARTESIAN_POINT('Ctrl Pts',(-37.4188654127938,17.5438230235078,-2.5));
#39390=CARTESIAN_POINT('Ctrl Pts',(-36.9198840261816,17.5827769733229,-2.99578898700793));
#39391=CARTESIAN_POINT('Ctrl Pts',(-36.9240615386413,17.5825477668969,-2.5));
#39392=CARTESIAN_POINT('Ctrl Pts',(-37.4192844801969,17.5537061882809,-2.5));
#39393=CARTESIAN_POINT('Ctrl Pts',(-36.9246169309371,17.6343825999131,-2.99109602673912));
#39394=CARTESIAN_POINT('Ctrl Pts',(-36.9333093941054,17.6333273268776,-2.5));
#39395=CARTESIAN_POINT('Ctrl Pts',(-37.4210593120151,17.5733143538484,-2.5));
#39396=CARTESIAN_POINT('Ctrl Pts',(-36.9282325359345,17.6599800335755,-2.98874837352374));
#39397=CARTESIAN_POINT('Ctrl Pts',(-36.9391161778231,17.6582989890867,-2.5));
#39398=CARTESIAN_POINT('Ctrl Pts',(-37.4224151662337,17.5830420307807,-2.5));
#39399=CARTESIAN_POINT('Ctrl Pts',(-36.9379460863992,17.710766834452,-2.98405135826386));
#39400=CARTESIAN_POINT('Ctrl Pts',(-36.9530417639778,17.7074272412772,-2.5));
#39401=CARTESIAN_POINT('Ctrl Pts',(-37.4260577504339,17.6023455517275,-2.5));
#39402=CARTESIAN_POINT('Ctrl Pts',(-36.9440439356691,17.7359562130125,-2.98170199150478));
#39403=CARTESIAN_POINT('Ctrl Pts',(-36.961150208635,17.7315882072703,-2.5));
#39404=CARTESIAN_POINT('Ctrl Pts',(-37.4283444361295,17.6119214029654,-2.5));
#39405=CARTESIAN_POINT('Ctrl Pts',(-36.9550940181883,17.7734276473997,-2.97817796458518));
#39406=CARTESIAN_POINT('Ctrl Pts',(-36.9750602300798,17.7672721065816,-2.5));
#39407=CARTESIAN_POINT('Ctrl Pts',(-37.4324882266632,17.6261687598122,-2.5));
#39408=CARTESIAN_POINT('Ctrl Pts',(-36.9590977423692,17.7858733013829,-2.97700260220075));
#39409=CARTESIAN_POINT('Ctrl Pts',(-36.9799820522302,17.7790613692586,-2.5));
#39410=CARTESIAN_POINT('Ctrl Pts',(-37.4339896230655,17.6309012462933,-2.5));
#39411=CARTESIAN_POINT('Ctrl Pts',(-36.9677444087214,17.8106277669609,-2.97465510692309));
#39412=CARTESIAN_POINT('Ctrl Pts',(-36.9903966889781,17.8024136686443,-2.5));
#39413=CARTESIAN_POINT('Ctrl Pts',(-37.437232116886,17.6403150006157,-2.5));
#39414=CARTESIAN_POINT('Ctrl Pts',(-36.9723569013568,17.8228504435788,-2.97349114599914));
#39415=CARTESIAN_POINT('Ctrl Pts',(-36.9958519245572,17.8138964486576,-2.5));
#39416=CARTESIAN_POINT('Ctrl Pts',(-37.4389618074377,17.6449635078328,-2.5));
#39417=CARTESIAN_POINT('Ctrl Pts',(-36.9968316404772,17.8831937506765,-2.96772154502321));
#39418=CARTESIAN_POINT('Ctrl Pts',(-37.0242345246282,17.8701746208594,-2.5));
#39419=CARTESIAN_POINT('Ctrl Pts',(-37.4481398206947,17.6679151360551,-2.5));
#39420=CARTESIAN_POINT('Ctrl Pts',(-37.0208955392833,17.9290397288272,-2.96326313438592));
#39421=CARTESIAN_POINT('Ctrl Pts',(-37.0507916007085,17.9123870158746,-2.5));
#39422=CARTESIAN_POINT('Ctrl Pts',(-37.4571637864037,17.6853590086553,-2.5));
#39423=CARTESIAN_POINT('Ctrl Pts',(-37.0636620936595,17.9942014163556,-2.95683590040463));
#39424=CARTESIAN_POINT('Ctrl Pts',(-37.0962159645972,17.9716354404605,-2.5));
#39425=CARTESIAN_POINT('Ctrl Pts',(-37.4732012555054,17.7101600273524,-2.5));
#39426=CARTESIAN_POINT('Ctrl Pts',(-37.0790511866489,18.0153339916105,-2.95473552840589));
#39427=CARTESIAN_POINT('Ctrl Pts',(-37.1122588011471,17.9906733177174,-2.5));
#39428=CARTESIAN_POINT('Ctrl Pts',(-37.4789721679196,17.7182046074472,-2.5));
#39429=CARTESIAN_POINT('Ctrl Pts',(-37.1121011063091,18.0562700748877,-2.95063882870761));
#39430=CARTESIAN_POINT('Ctrl Pts',(-37.1461872334036,18.0272996809472,-2.5));
#39431=CARTESIAN_POINT('Ctrl Pts',(-37.4913658752322,17.733790264152,-2.5));
#39432=CARTESIAN_POINT('Ctrl Pts',(-37.1295103581676,18.0757653348942,-2.94867340342006));
#39433=CARTESIAN_POINT('Ctrl Pts',(-37.1638134804818,18.0446236356694,-2.5));
#39434=CARTESIAN_POINT('Ctrl Pts',(-37.4978943532022,17.7412139562433,-2.5));
#39435=CARTESIAN_POINT('Ctrl Pts',(-37.1843057553075,18.1314233942583,-2.94302770433399));
#39436=CARTESIAN_POINT('Ctrl Pts',(-37.2185148052678,18.0936922878623,-2.5));
#39437=CARTESIAN_POINT('Ctrl Pts',(-37.5184426204004,17.7624112761694,-2.5));
#39438=CARTESIAN_POINT('Ctrl Pts',(-37.2242361969918,18.1647864737446,-2.93959528754205));
#39439=CARTESIAN_POINT('Ctrl Pts',(-37.2575873678388,18.1227938260313,-2.5));
#39440=CARTESIAN_POINT('Ctrl Pts',(-37.5334165320212,17.7751217694643,-2.5));
#39441=CARTESIAN_POINT('Ctrl Pts',(-37.278501267837,18.2017080527822,-2.93576187067611));
#39442=CARTESIAN_POINT('Ctrl Pts',(-37.3098415222596,18.154743770369,-2.5));
#39443=CARTESIAN_POINT('Ctrl Pts',(-37.5537659442094,17.7891910078983,-2.5));
#39444=CARTESIAN_POINT('Ctrl Pts',(-37.2895908939828,18.2088614252754,-2.9350171685076));
#39445=CARTESIAN_POINT('Ctrl Pts',(-37.3204553852497,18.1609059986669,-2.5));
#39446=CARTESIAN_POINT('Ctrl Pts',(-37.5579245541323,17.7919170308987,-2.5));
#39447=CARTESIAN_POINT('Ctrl Pts',(-37.3121456740118,18.222628713375,-2.93358056573866));
#39448=CARTESIAN_POINT('Ctrl Pts',(-37.3419594345533,18.1727383129417,-2.5));
#39449=CARTESIAN_POINT('Ctrl Pts',(-37.5663825921581,17.7971638038772,-2.5));
#39450=CARTESIAN_POINT('Ctrl Pts',(-37.3235504689819,18.2292070024891,-2.93289238561845));
#39451=CARTESIAN_POINT('Ctrl Pts',(-37.3527929576584,18.1783789941509,-2.5));
#39452=CARTESIAN_POINT('Ctrl Pts',(-37.5706593939047,17.7996709619125,-2.5));
#39453=CARTESIAN_POINT('Ctrl Pts',(-37.3581397345302,18.2480437180578,-2.93091764257171));
#39454=CARTESIAN_POINT('Ctrl Pts',(-37.3855178350711,18.1944875128524,-2.5));
#39455=CARTESIAN_POINT('Ctrl Pts',(-37.5836303643146,17.8068505202015,-2.5));
#39456=CARTESIAN_POINT('Ctrl Pts',(-37.3816981781207,18.2594061256977,-2.92972067272748));
#39457=CARTESIAN_POINT('Ctrl Pts',(-37.4076765730136,18.2041692805068,-2.5));
#39458=CARTESIAN_POINT('Ctrl Pts',(-37.5924647836065,17.811181769741,-2.5));
#39459=CARTESIAN_POINT('Ctrl Pts',(-37.4297964715305,18.2797809159781,-2.92756741754469));
#39460=CARTESIAN_POINT('Ctrl Pts',(-37.4526661261266,18.2214705311287,-2.5));
#39461=CARTESIAN_POINT('Ctrl Pts',(-37.6105016433052,17.8189490809156,-2.5));
#39462=CARTESIAN_POINT('Ctrl Pts',(-37.4543363298823,18.2887932678948,-2.92661112217483));
#39463=CARTESIAN_POINT('Ctrl Pts',(-37.4755052012686,18.2290974806186,-2.5));
#39464=CARTESIAN_POINT('Ctrl Pts',(-37.6197040888717,17.8223851300001,-2.5));
#39465=CARTESIAN_POINT('Ctrl Pts',(-37.4918913116176,18.3005282374446,-2.92536297515959));
#39466=CARTESIAN_POINT('Ctrl Pts',(-37.5103223388011,18.2390056374751,-2.5));
#39467=CARTESIAN_POINT('Ctrl Pts',(-37.633787209243,17.8268594543971,-2.5));
#39468=CARTESIAN_POINT('Ctrl Pts',(-37.5045340558524,18.3041421023044,-2.92497802297482));
#39469=CARTESIAN_POINT('Ctrl Pts',(-37.5220166849113,18.2420518473036,-2.5));
#39470=CARTESIAN_POINT('Ctrl Pts',(-37.6385282366181,17.8282374131812,-2.5));
#39471=CARTESIAN_POINT('Ctrl Pts',(-37.5236880380742,18.3091085696021,-2.92444842107095));
#39472=CARTESIAN_POINT('Ctrl Pts',(-37.5397059345923,18.2462341178242,-2.5));
#39473=CARTESIAN_POINT('Ctrl Pts',(-37.6457109814105,17.8301311528227,-2.5));
#39474=CARTESIAN_POINT('Ctrl Pts',(-37.530104354971,18.310688300037,-2.92427986194296));
#39475=CARTESIAN_POINT('Ctrl Pts',(-37.5456258343898,18.2475634797771,-2.5));
#39476=CARTESIAN_POINT('Ctrl Pts',(-37.6481170992389,17.8307335274115,-2.5));
#39477=CARTESIAN_POINT('Ctrl Pts',(-37.5430010389201,18.3136945178689,-2.9239589307846));
#39478=CARTESIAN_POINT('Ctrl Pts',(-37.5575155990342,18.2500919427414,-2.5));
#39479=CARTESIAN_POINT('Ctrl Pts',(-37.6529533567628,17.8318798449285,-2.5));
#39480=CARTESIAN_POINT('Ctrl Pts',(-37.5494894557846,18.3151225191071,-2.92380639706833));
#39481=CARTESIAN_POINT('Ctrl Pts',(-37.5634930070409,18.2512923999885,-2.5));
#39482=CARTESIAN_POINT('Ctrl Pts',(-37.6553865130038,17.8324243739287,-2.5));
#39483=CARTESIAN_POINT('Ctrl Pts',(-37.6078715508142,18.3272151542962,-2.92251412976417));
#39484=CARTESIAN_POINT('Ctrl Pts',(-37.6171933811497,18.261444733944,-2.5));
#39485=CARTESIAN_POINT('Ctrl Pts',(-37.6772797946946,17.8370356375276,-2.5));
#39486=CARTESIAN_POINT('Ctrl Pts',(-37.6600314084477,18.3327140130362,-2.92192313396902));
#39487=CARTESIAN_POINT('Ctrl Pts',(-37.6650031743221,18.2660494018553,-2.5));
#39488=CARTESIAN_POINT('Ctrl Pts',(-37.6968397447769,17.8391327868468,-2.5));
#39489=CARTESIAN_POINT('Ctrl Pts',(-37.7386551922739,18.3333477986367,-2.92185513454714));
#39490=CARTESIAN_POINT('Ctrl Pts',(-37.7369884997638,18.2665799642824,-2.5));
#39491=CARTESIAN_POINT('Ctrl Pts',(-37.7263236637676,17.8393744833388,-2.5));
#39492=CARTESIAN_POINT('Ctrl Pts',(-37.7649275847458,18.332280602678,-2.92196969819476));
#39493=CARTESIAN_POINT('Ctrl Pts',(-37.7610453062294,18.2656866234871,-2.5));
#39494=CARTESIAN_POINT('Ctrl Pts',(-37.7361758116312,17.8389674969796,-2.5));
#39495=CARTESIAN_POINT('Ctrl Pts',(-37.8044355425913,18.3287092953001,-2.9223525645861));
#39496=CARTESIAN_POINT('Ctrl Pts',(-37.7972513234411,18.2626950729203,-2.5));
#39497=CARTESIAN_POINT('Ctrl Pts',(-37.7509912947654,17.8376055413245,-2.5));
#39498=CARTESIAN_POINT('Ctrl Pts',(-37.8176556209491,18.3271839572083,-2.92251604054704));
#39499=CARTESIAN_POINT('Ctrl Pts',(-37.8093757241164,18.2614166995762,-2.5));
#39500=CARTESIAN_POINT('Ctrl Pts',(-37.7559488239131,17.8370238468006,-2.5));
#39501=CARTESIAN_POINT('Ctrl Pts',(-37.8438653515097,18.3235000632348,-2.92291055095015));
#39502=CARTESIAN_POINT('Ctrl Pts',(-37.8334337540048,18.2583273875558,-2.5));
#39503=CARTESIAN_POINT('Ctrl Pts',(-37.7657774740514,17.8356190137894,-2.5));
#39504=CARTESIAN_POINT('Ctrl Pts',(-37.8568746743686,18.321341537448,-2.92314158144293));
#39505=CARTESIAN_POINT('Ctrl Pts',(-37.8453867146324,18.256516085823,-2.5));
#39506=CARTESIAN_POINT('Ctrl Pts',(-37.7706559690046,17.8347958710238,-2.5));
#39507=CARTESIAN_POINT('Ctrl Pts',(-37.9214525991908,18.3089956020391,-2.92446167772975));
#39508=CARTESIAN_POINT('Ctrl Pts',(-37.9048311581349,18.2461405986857,-2.5));
#39509=CARTESIAN_POINT('Ctrl Pts',(-37.7948726934621,17.8300879827949,-2.5));
#39510=CARTESIAN_POINT('Ctrl Pts',(-37.971628515283,18.2941930137726,-2.92604160841261));
#39511=CARTESIAN_POINT('Ctrl Pts',(-37.951260778169,18.233665691823,-2.5));
#39512=CARTESIAN_POINT('Ctrl Pts',(-37.8136886637651,17.8244435332827,-2.5));
#39513=CARTESIAN_POINT('Ctrl Pts',(-38.0324952429552,18.2695437413729,-2.9286496092432));
#39514=CARTESIAN_POINT('Ctrl Pts',(-38.0080199920834,18.2127861786537,-2.5));
#39515=CARTESIAN_POINT('Ctrl Pts',(-37.8365136817825,17.8150464189915,-2.5));
#39516=CARTESIAN_POINT('Ctrl Pts',(-38.044575088039,18.264303794869,-2.92920311231327));
#39517=CARTESIAN_POINT('Ctrl Pts',(-38.0193295823946,18.208334158798,-2.5));
#39518=CARTESIAN_POINT('Ctrl Pts',(-37.8410436263355,17.8130488679072,-2.5));
#39519=CARTESIAN_POINT('Ctrl Pts',(-38.0685444585904,18.2531925029883,-2.93037437162195));
#39520=CARTESIAN_POINT('Ctrl Pts',(-38.0418344218168,18.1988760473144,-2.5));
#39521=CARTESIAN_POINT('Ctrl Pts',(-37.850032136943,17.8088132624928,-2.5));
#39522=CARTESIAN_POINT('Ctrl Pts',(-38.0804306041699,18.2473200654554,-2.93099223718261));
#39523=CARTESIAN_POINT('Ctrl Pts',(-38.0530277696176,18.1938679552602,-2.5));
#39524=CARTESIAN_POINT('Ctrl Pts',(-37.8544894413598,17.8065748058377,-2.5));
#39525=CARTESIAN_POINT('Ctrl Pts',(-38.1154058739446,18.2289535054552,-2.93292028761117));
#39526=CARTESIAN_POINT('Ctrl Pts',(-38.0860884329982,18.1781636427194,-2.5));
#39527=CARTESIAN_POINT('Ctrl Pts',(-37.8676051730758,17.7995742349009,-2.5));
#39528=CARTESIAN_POINT('Ctrl Pts',(-38.1379498775984,18.2156512801827,-2.93431116406502));
#39529=CARTESIAN_POINT('Ctrl Pts',(-38.107532686332,18.1667488029368,-2.5));
#39530=CARTESIAN_POINT('Ctrl Pts',(-37.8760591693826,17.7945044510302,-2.5));
#39531=CARTESIAN_POINT('Ctrl Pts',(-38.2033280576451,18.17265741314,-2.93878236806526));
#39532=CARTESIAN_POINT('Ctrl Pts',(-38.1702794467489,18.1296291178422,-2.5));
#39533=CARTESIAN_POINT('Ctrl Pts',(-37.9005759909892,17.7781206666248,-2.5));
#39534=CARTESIAN_POINT('Ctrl Pts',(-38.2439301407294,18.1399084455847,-2.94215865140722));
#39535=CARTESIAN_POINT('Ctrl Pts',(-38.2098765411374,18.1011163150348,-2.5));
#39536=CARTESIAN_POINT('Ctrl Pts',(-37.9158017810326,17.7656435334912,-2.5));
#39537=CARTESIAN_POINT('Ctrl Pts',(-38.2908370693989,18.0936969886663,-2.94685549765066));
#39538=CARTESIAN_POINT('Ctrl Pts',(-38.2564928085569,18.0604885105553,-2.5));
#39539=CARTESIAN_POINT('Ctrl Pts',(-37.9333918647676,17.7480431201017,-2.5));
#39540=CARTESIAN_POINT('Ctrl Pts',(-38.2999735282245,18.0842373184233,-2.94781393656573));
#39541=CARTESIAN_POINT('Ctrl Pts',(-38.2656503724343,18.0521248196139,-2.5));
#39542=CARTESIAN_POINT('Ctrl Pts',(-37.9368180370691,17.744440511481,-2.5));
#39543=CARTESIAN_POINT('Ctrl Pts',(-38.3176873507553,18.0649722522993,-2.94975921175979));
#39544=CARTESIAN_POINT('Ctrl Pts',(-38.2835158468797,18.035036707545,-2.5));
#39545=CARTESIAN_POINT('Ctrl Pts',(-37.9434607258409,17.7371042069719,-2.5));
#39546=CARTESIAN_POINT('Ctrl Pts',(-38.3262776360071,18.0551541758763,-2.95074733976652));
#39547=CARTESIAN_POINT('Ctrl Pts',(-38.292236426,18.0262999067001,-2.5));
#39548=CARTESIAN_POINT('Ctrl Pts',(-37.9466820784148,17.7333656728621,-2.5));
#39549=CARTESIAN_POINT('Ctrl Pts',(-38.3512613834271,18.0251519219321,-2.95375629684687));
#39550=CARTESIAN_POINT('Ctrl Pts',(-38.3177954315766,17.9994877930366,-2.5));
#39551=CARTESIAN_POINT('Ctrl Pts',(-37.9560509888996,17.721942323421,-2.5));
#39552=CARTESIAN_POINT('Ctrl Pts',(-38.3668695803311,18.0044210131818,-2.95582157994119));
#39553=CARTESIAN_POINT('Ctrl Pts',(-38.3339844060987,17.9808535987548,-2.5));
#39554=CARTESIAN_POINT('Ctrl Pts',(-37.9619040598854,17.7140502257561,-2.5));
#39555=CARTESIAN_POINT('Ctrl Pts',(-38.3960122766866,17.96151412598,-2.96006384799544));
#39556=CARTESIAN_POINT('Ctrl Pts',(-38.3647032001448,17.9420087393569,-2.5));
#39557=CARTESIAN_POINT('Ctrl Pts',(-37.9728325697887,17.6977186737315,-2.5));
#39558=CARTESIAN_POINT('Ctrl Pts',(-38.4095468146066,17.9393381811376,-2.96224084544494));
#39559=CARTESIAN_POINT('Ctrl Pts',(-38.3792301089262,17.921787539762,-2.5));
#39560=CARTESIAN_POINT('Ctrl Pts',(-37.9779080274105,17.6892792325375,-2.5));
#39561=CARTESIAN_POINT('Ctrl Pts',(-38.4282645108262,17.904969535058,-2.96558787871309));
#39562=CARTESIAN_POINT('Ctrl Pts',(-38.399714653804,17.8902405113807,-2.5));
#39563=CARTESIAN_POINT('Ctrl Pts',(-37.9849271555627,17.6762019272695,-2.5));
#39564=CARTESIAN_POINT('Ctrl Pts',(-38.4342446366122,17.89331766282,-2.96671826104229));
#39565=CARTESIAN_POINT('Ctrl Pts',(-38.4063407380303,17.8794930259532,-2.5));
#39566=CARTESIAN_POINT('Ctrl Pts',(-37.9871697012262,17.6717687488141,-2.5));
#39567=CARTESIAN_POINT('Ctrl Pts',(-38.4456424175336,17.8696845533725,-2.96900170083772));
#39568=CARTESIAN_POINT('Ctrl Pts',(-38.4191252098151,17.8576079915772,-2.5));
#39569=CARTESIAN_POINT('Ctrl Pts',(-37.991443877371,17.6627778699454,-2.5));
#39570=CARTESIAN_POINT('Ctrl Pts',(-38.4510249910641,17.8577775263316,-2.9701475957582));
#39571=CARTESIAN_POINT('Ctrl Pts',(-38.4252432488303,17.8465380939854,-2.5));
#39572=CARTESIAN_POINT('Ctrl Pts',(-37.9934623353037,17.6582483931711,-2.5));
#39573=CARTESIAN_POINT('Ctrl Pts',(-38.4763900971177,17.7977995570222,-2.97589627219185));
#39574=CARTESIAN_POINT('Ctrl Pts',(-38.4545812226388,17.790369539723,-2.5));
#39575=CARTESIAN_POINT('Ctrl Pts',(-38.002974265032,17.6354345524181,-2.5));
#39576=CARTESIAN_POINT('Ctrl Pts',(-38.4917731732021,17.7484124059281,-2.98055544920644));
#39577=CARTESIAN_POINT('Ctrl Pts',(-38.473661265785,17.7435263663243,-2.5));
#39578=CARTESIAN_POINT('Ctrl Pts',(-38.0087429143111,17.6166554164039,-2.5));
#39579=CARTESIAN_POINT('Ctrl Pts',(-38.5049497227733,17.6849440597232,-2.9864412217583));
#39580=CARTESIAN_POINT('Ctrl Pts',(-38.4919775578133,17.6825071777955,-2.5));
#39581=CARTESIAN_POINT('Ctrl Pts',(-38.0136841107577,17.5925304537987,-2.5));
#39582=CARTESIAN_POINT('Ctrl Pts',(-38.5072797054594,17.6721629059777,-2.9876215411643));
#39583=CARTESIAN_POINT('Ctrl Pts',(-38.4953743016544,17.6701248728446,-2.5));
#39584=CARTESIAN_POINT('Ctrl Pts',(-38.0145578594488,17.5876726194739,-2.5));
#39585=CARTESIAN_POINT('Ctrl Pts',(-38.5113201026512,17.646423044551,-2.98998846097813));
#39586=CARTESIAN_POINT('Ctrl Pts',(-38.501596520551,17.645080935214,-2.5));
#39587=CARTESIAN_POINT('Ctrl Pts',(-38.0160730018852,17.5778902994518,-2.5));
#39588=CARTESIAN_POINT('Ctrl Pts',(-38.5130325575213,17.6334445126556,-2.99117686889631));
#39589=CARTESIAN_POINT('Ctrl Pts',(-38.5044245550668,17.6323990130624,-2.5));
#39590=CARTESIAN_POINT('Ctrl Pts',(-38.0167151730816,17.5729582831273,-2.5));
#39591=CARTESIAN_POINT('Ctrl Pts',(-38.5172060896891,17.5943721213219,-2.99473928414168));
#39592=CARTESIAN_POINT('Ctrl Pts',(-38.5120043473919,17.5940082770842,-2.5));
#39593=CARTESIAN_POINT('Ctrl Pts',(-38.0182802555498,17.5581115117232,-2.5));
#39594=CARTESIAN_POINT('Ctrl Pts',(-38.5186917422194,17.5683120165936,-2.99709499970835));
#39595=CARTESIAN_POINT('Ctrl Pts',(-38.5157988525533,17.5682102346573,-2.5));
#39596=CARTESIAN_POINT('Ctrl Pts',(-38.0188373699573,17.5482108332471,-2.5));
#39597=CARTESIAN_POINT('Ctrl Pts',(-38.5191072198307,17.5161686034308,-3.00176886678129));
#39598=CARTESIAN_POINT('Ctrl Pts',(-38.5208771553493,17.5161399120222,-2.5));
#39599=CARTESIAN_POINT('Ctrl Pts',(-38.0189931741039,17.5284038967669,-2.5));
#39600=CARTESIAN_POINT('Ctrl Pts',(-38.5180370412835,17.4900852974077,-3.00408701695548));
#39601=CARTESIAN_POINT('Ctrl Pts',(-38.5221491625175,17.4898665253747,-2.5));
#39602=CARTESIAN_POINT('Ctrl Pts',(-38.0185918623631,17.5184976387542,-2.5));
#39603=CARTESIAN_POINT('Ctrl Pts',(-38.5144871859473,17.4509429730902,-3.00753674366307));
#39604=CARTESIAN_POINT('Ctrl Pts',(-38.5220957984724,17.4501405073408,-2.5));
#39605=CARTESIAN_POINT('Ctrl Pts',(-38.0172606587587,17.5036340064431,-2.5));
#39606=CARTESIAN_POINT('Ctrl Pts',(-38.512979645677,17.4379142878159,-3.00868013835556));
#39607=CARTESIAN_POINT('Ctrl Pts',(-38.5217466988597,17.4368445410147,-2.5));
#39608=CARTESIAN_POINT('Ctrl Pts',(-38.0166953304505,17.4986869777819,-2.5));
#39609=CARTESIAN_POINT('Ctrl Pts',(-38.5093456409823,17.4120774324436,-3.01093824610606));
#39610=CARTESIAN_POINT('Ctrl Pts',(-38.5203938380985,17.4103637207151,-2.5));
#39611=CARTESIAN_POINT('Ctrl Pts',(-38.0153325853393,17.4888774005165,-2.5));
#39612=CARTESIAN_POINT('Ctrl Pts',(-38.5072169868592,17.3992427493601,-3.01205529745571));
#39613=CARTESIAN_POINT('Ctrl Pts',(-38.5193887795888,17.3971525411347,-2.5));
#39614=CARTESIAN_POINT('Ctrl Pts',(-38.014534334724,17.4840047859771,-2.5));
#39615=CARTESIAN_POINT('Ctrl Pts',(-38.4950383810716,17.335482072003,-3.01758225181016));
#39616=CARTESIAN_POINT('Ctrl Pts',(-38.512708363373,17.3310164313404,-2.5));
#39617=CARTESIAN_POINT('Ctrl Pts',(-38.0099673675257,17.4598001953765,-2.5));
#39618=CARTESIAN_POINT('Ctrl Pts',(-38.4804258988967,17.2857825382543,-3.02181836676292));
#39619=CARTESIAN_POINT('Ctrl Pts',(-38.5021474563194,17.2787657562271,-2.5));
#39620=CARTESIAN_POINT('Ctrl Pts',(-38.0044876905449,17.4409392110453,-2.5));
#39621=CARTESIAN_POINT('Ctrl Pts',(-38.4559979025521,17.2253187773268,-3.02689693274587));
#39622=CARTESIAN_POINT('Ctrl Pts',(-38.482188384964,17.2143685236006,-2.5));
#39623=CARTESIAN_POINT('Ctrl Pts',(-37.9953271771502,17.4179991279534,-2.5));
#39624=CARTESIAN_POINT('Ctrl Pts',(-38.4508014471794,17.2133098047403,-3.02790174447839));
#39625=CARTESIAN_POINT('Ctrl Pts',(-38.4778364738777,17.2014855815011,-2.5));
#39626=CARTESIAN_POINT('Ctrl Pts',(-37.9933785134793,17.4134431981463,-2.5));
#39627=CARTESIAN_POINT('Ctrl Pts',(-38.4425304868847,17.1954247892708,-3.02939268814916));
#39628=CARTESIAN_POINT('Ctrl Pts',(-38.4707770006933,17.1822327898589,-2.5));
#39629=CARTESIAN_POINT('Ctrl Pts',(-37.9902768971576,17.4066584740223,-2.5));
#39630=CARTESIAN_POINT('Ctrl Pts',(-38.4396936273783,17.1894842833032,-3.02988697260699));
#39631=CARTESIAN_POINT('Ctrl Pts',(-38.4683326604495,17.1758218953105,-2.5));
#39632=CARTESIAN_POINT('Ctrl Pts',(-37.9892130751568,17.4044050008767,-2.5));
#39633=CARTESIAN_POINT('Ctrl Pts',(-38.433892526343,17.1777122168892,-3.03086468827693));
#39634=CARTESIAN_POINT('Ctrl Pts',(-38.4632915541776,17.1630927437411,-2.5));
#39635=CARTESIAN_POINT('Ctrl Pts',(-37.9870376657812,17.3999395207739,-2.5));
#39636=CARTESIAN_POINT('Ctrl Pts',(-38.4309245022383,17.1718722889636,-3.03134881683581));
#39637=CARTESIAN_POINT('Ctrl Pts',(-38.4606914472883,17.1567656550912,-2.5));
#39638=CARTESIAN_POINT('Ctrl Pts',(-37.9859246535537,17.3977243429034,-2.5));
#39639=CARTESIAN_POINT('Ctrl Pts',(-38.4157502976598,17.1429009507965,-3.03374623521863));
#39640=CARTESIAN_POINT('Ctrl Pts',(-38.4472751802113,17.1252685427155,-2.5));
#39641=CARTESIAN_POINT('Ctrl Pts',(-37.9802343339963,17.3867353766995,-2.5));
#39642=CARTESIAN_POINT('Ctrl Pts',(-38.4025443177972,17.1204528053856,-3.03559000380591));
#39643=CARTESIAN_POINT('Ctrl Pts',(-38.4352923297066,17.1007128648909,-2.5));
#39644=CARTESIAN_POINT('Ctrl Pts',(-37.9752820848364,17.3782217794531,-2.5));
#39645=CARTESIAN_POINT('Ctrl Pts',(-38.3597927098826,17.0552514733911,-3.04091068696068));
#39646=CARTESIAN_POINT('Ctrl Pts',(-38.3955062069388,17.0287324610293,-2.5));
#39647=CARTESIAN_POINT('Ctrl Pts',(-37.9592502348198,17.3534964507582,-2.5));
#39648=CARTESIAN_POINT('Ctrl Pts',(-38.3271443327293,17.0146202226201,-3.04417881485026));
#39649=CARTESIAN_POINT('Ctrl Pts',(-38.3640171485458,16.9833146484955,-2.5));
#39650=CARTESIAN_POINT('Ctrl Pts',(-37.9470071050743,17.3380921508149,-2.5));
#39651=CARTESIAN_POINT('Ctrl Pts',(-38.2809131555838,16.9675438780044,-3.0479256286666));
#39652=CARTESIAN_POINT('Ctrl Pts',(-38.3181512189723,16.9301557601742,-2.5));
#39653=CARTESIAN_POINT('Ctrl Pts',(-37.9296703965765,17.3202474359949,-2.5));
#39654=CARTESIAN_POINT('Ctrl Pts',(-38.2714380751677,16.9583630961748,-3.04865416425237));
#39655=CARTESIAN_POINT('Ctrl Pts',(-38.3086648857525,16.9197304651529,-2.5));
#39656=CARTESIAN_POINT('Ctrl Pts',(-37.9261172426642,17.3167675393722,-2.5));
#39657=CARTESIAN_POINT('Ctrl Pts',(-38.2521347050763,16.9405580024456,-3.05006336142326));
#39658=CARTESIAN_POINT('Ctrl Pts',(-38.2892172779821,16.8994516379931,-2.5));
#39659=CARTESIAN_POINT('Ctrl Pts',(-37.9188784832198,17.3100189529994,-2.5));
#39660=CARTESIAN_POINT('Ctrl Pts',(-38.2422914181653,16.9319183323786,-3.05074524347667));
#39661=CARTESIAN_POINT('Ctrl Pts',(-38.2792412041749,16.8895824979303,-2.5));
#39662=CARTESIAN_POINT('Ctrl Pts',(-37.9151872472733,17.3067444493034,-2.5));
#39663=CARTESIAN_POINT('Ctrl Pts',(-38.2121946005029,16.9067773575311,-3.05272459995863));
#39664=CARTESIAN_POINT('Ctrl Pts',(-38.2485441235301,16.860762254136,-2.5));
#39665=CARTESIAN_POINT('Ctrl Pts',(-37.9039009442048,17.2972161773508,-2.5));
#39666=CARTESIAN_POINT('Ctrl Pts',(-38.1913754559341,16.8910522598471,-3.05395594589729));
#39667=CARTESIAN_POINT('Ctrl Pts',(-38.227102342556,16.842648790628,-2.5));
#39668=CARTESIAN_POINT('Ctrl Pts',(-37.8960937635255,17.2912569793141,-2.5));
#39669=CARTESIAN_POINT('Ctrl Pts',(-38.1482366444428,16.861662216655,-3.05624785925289));
#39670=CARTESIAN_POINT('Ctrl Pts',(-38.1822556751584,16.8086281750341,-2.5));
#39671=CARTESIAN_POINT('Ctrl Pts',(-37.8799167074083,17.280120019,-2.5));
#39672=CARTESIAN_POINT('Ctrl Pts',(-38.1259170445788,16.8479971821675,-3.05730841943199));
#39673=CARTESIAN_POINT('Ctrl Pts',(-38.1588541824173,16.7927328735794,-2.5));
#39674=CARTESIAN_POINT('Ctrl Pts',(-37.8715468617295,17.274942215395,-2.5));
#39675=CARTESIAN_POINT('Ctrl Pts',(-38.0912859803399,16.829081464749,-3.05877140147105));
#39676=CARTESIAN_POINT('Ctrl Pts',(-38.1222868782628,16.7706491428746,-2.5));
#39677=CARTESIAN_POINT('Ctrl Pts',(-37.8585602075906,17.2677752860875,-2.5));
#39678=CARTESIAN_POINT('Ctrl Pts',(-38.0795482163152,16.8230394748505,-3.05923777409933));
#39679=CARTESIAN_POINT('Ctrl Pts',(-38.1098421306826,16.7635765111134,-2.5));
#39680=CARTESIAN_POINT('Ctrl Pts',(-37.854158548831,17.2654861133914,-2.5));
#39681=CARTESIAN_POINT('Ctrl Pts',(-38.0556863997546,16.8114994618048,-3.06012706376275));
#39682=CARTESIAN_POINT('Ctrl Pts',(-38.0844586622232,16.7500420272248,-2.5));
#39683=CARTESIAN_POINT('Ctrl Pts',(-37.8452103654877,17.2611139901796,-2.5));
#39684=CARTESIAN_POINT('Ctrl Pts',(-38.0436500462945,16.8060440839517,-3.06054669237718));
#39685=CARTESIAN_POINT('Ctrl Pts',(-38.0716141384825,16.7436315079723,-2.5));
#39686=CARTESIAN_POINT('Ctrl Pts',(-37.8406967327678,17.2590471876283,-2.5));
#39687=CARTESIAN_POINT('Ctrl Pts',(-37.983033732995,16.7803474050268,-3.06252042955387));
#39688=CARTESIAN_POINT('Ctrl Pts',(-38.006651933923,16.7133430503521,-2.5));
#39689=CARTESIAN_POINT('Ctrl Pts',(-37.817965621475,17.2493120442009,-2.5));
#39690=CARTESIAN_POINT('Ctrl Pts',(-37.9330756082843,16.7647592929747,-3.06370859239269));
#39691=CARTESIAN_POINT('Ctrl Pts',(-37.9526360706556,16.6948699048902,-2.5));
#39692=CARTESIAN_POINT('Ctrl Pts',(-37.7992313215639,17.2434072153618,-2.5));
#39693=CARTESIAN_POINT('Ctrl Pts',(-37.8688152137882,16.7514251465279,-3.06472324864037));
#39694=CARTESIAN_POINT('Ctrl Pts',(-37.8827461609207,16.6790214482703,-2.5));
#39695=CARTESIAN_POINT('Ctrl Pts',(-37.7751336713641,17.2383563320521,-2.5));
#39696=CARTESIAN_POINT('Ctrl Pts',(-37.8558716761049,16.7490686581359,-3.06490240337987));
#39697=CARTESIAN_POINT('Ctrl Pts',(-37.8686399794402,16.6762161508003,-2.5));
#39698=CARTESIAN_POINT('Ctrl Pts',(-37.7702798457447,17.2374637147322,-2.5));
#39699=CARTESIAN_POINT('Ctrl Pts',(-37.836316999401,16.7460068446618,-3.06513506367886));
#39700=CARTESIAN_POINT('Ctrl Pts',(-37.8473067499512,16.6725690712863,-2.5));
#39701=CARTESIAN_POINT('Ctrl Pts',(-37.762946841142,17.2363039481978,-2.5));
#39702=CARTESIAN_POINT('Ctrl Pts',(-37.829775537342,16.7450650975492,-3.06520660039349));
#39703=CARTESIAN_POINT('Ctrl Pts',(-37.8401659882031,16.6714468083953,-2.5));
#39704=CARTESIAN_POINT('Ctrl Pts',(-37.7604937934312,17.23594722548,-2.5));
#39705=CARTESIAN_POINT('Ctrl Pts',(-37.8166456311835,16.7433410180028,-3.0653375358751));
#39706=CARTESIAN_POINT('Ctrl Pts',(-37.82582654984,16.669391703467,-2.5));
#39707=CARTESIAN_POINT('Ctrl Pts',(-37.7555700780584,17.2352941782029,-2.5));
#39708=CARTESIAN_POINT('Ctrl Pts',(-37.8100479347227,16.7425577604292,-3.06539700330435));
#39709=CARTESIAN_POINT('Ctrl Pts',(-37.818617934926,16.668457783908,-2.5));
#39710=CARTESIAN_POINT('Ctrl Pts',(-37.7530959419294,17.2349974951212,-2.5));
#39711=CARTESIAN_POINT('Ctrl Pts',(-37.777067284866,16.7390579643222,-3.06566266886128));
#39712=CARTESIAN_POINT('Ctrl Pts',(-37.7825632243643,16.6642830215665,-2.5));
#39713=CARTESIAN_POINT('Ctrl Pts',(-37.7407281994226,17.2336718308661,-2.5));
#39714=CARTESIAN_POINT('Ctrl Pts',(-37.7507569280122,16.7375882697876,-3.06577409663493));
#39715=CARTESIAN_POINT('Ctrl Pts',(-37.7537706577765,16.6625286572503,-2.5));
#39716=CARTESIAN_POINT('Ctrl Pts',(-37.7308618146269,17.2331151625715,-2.5));
#39717=CARTESIAN_POINT('Ctrl Pts',(-37.6720409935013,16.7370385868534,-3.06581578422071));
#39718=CARTESIAN_POINT('Ctrl Pts',(-37.6675998077381,16.6618723975768,-2.5));
#39719=CARTESIAN_POINT('Ctrl Pts',(-37.7013433392571,17.2329069461004,-2.5));
#39720=CARTESIAN_POINT('Ctrl Pts',(-37.6198485285534,16.7417812990776,-3.06545669284864));
#39721=CARTESIAN_POINT('Ctrl Pts',(-37.6105054868964,16.6675345545024,-2.5));
#39722=CARTESIAN_POINT('Ctrl Pts',(-37.6817711620469,17.2347033137879,-2.5));
#39723=CARTESIAN_POINT('Ctrl Pts',(-37.5549716201007,16.7542328279335,-3.06450964654665));
#39724=CARTESIAN_POINT('Ctrl Pts',(-37.539791579201,16.6823618030451,-2.5));
#39725=CARTESIAN_POINT('Ctrl Pts',(-37.6574423248857,17.2394198627989,-2.5));
#39726=CARTESIAN_POINT('Ctrl Pts',(-37.5419780772432,16.7570618699045,-3.06429433377577));
#39727=CARTESIAN_POINT('Ctrl Pts',(-37.5256575742345,16.6857256023118,-2.5));
#39728=CARTESIAN_POINT('Ctrl Pts',(-37.6525697466396,17.2404914902659,-2.5));
#39729=CARTESIAN_POINT('Ctrl Pts',(-37.5162549007385,16.7633361071356,-3.06381631649363));
#39730=CARTESIAN_POINT('Ctrl Pts',(-37.4977213282955,16.6931780113973,-2.5));
#39731=CARTESIAN_POINT('Ctrl Pts',(-37.642923553396,17.2428681687046,-2.5));
#39732=CARTESIAN_POINT('Ctrl Pts',(-37.5035214136028,16.7667796187423,-3.0635537446777));
#39733=CARTESIAN_POINT('Ctrl Pts',(-37.4839161235599,16.6972638969602,-2.5));
#39734=CARTESIAN_POINT('Ctrl Pts',(-37.6381484975799,17.2441725977466,-2.5));
#39735=CARTESIAN_POINT('Ctrl Pts',(-37.4656977945507,16.7780114577165,-3.06269625818825));
#39736=CARTESIAN_POINT('Ctrl Pts',(-37.4430016133797,16.7105699687229,-2.5));
#39737=CARTESIAN_POINT('Ctrl Pts',(-37.6239646379375,17.2484273528784,-2.5));
#39738=CARTESIAN_POINT('Ctrl Pts',(-37.4409836224016,16.7866989403601,-3.06203177270948));
#39739=CARTESIAN_POINT('Ctrl Pts',(-37.4163729269822,16.720839368388,-2.5));
#39740=CARTESIAN_POINT('Ctrl Pts',(-37.6146968252125,17.2517183816627,-2.5));
#39741=CARTESIAN_POINT('Ctrl Pts',(-37.3925416751236,16.80643246839,-3.06051737328866));
#39742=CARTESIAN_POINT('Ctrl Pts',(-37.3644453567216,16.7440900855917,-2.5));
#39743=CARTESIAN_POINT('Ctrl Pts',(-37.5965310946519,17.2591942841924,-2.5));
#39744=CARTESIAN_POINT('Ctrl Pts',(-37.3688139142769,16.8174785426132,-3.05966746752498));
#39745=CARTESIAN_POINT('Ctrl Pts',(-37.3391549609578,16.7570619950295,-2.5));
#39746=CARTESIAN_POINT('Ctrl Pts',(-37.5876331822018,17.2633791709517,-2.5));
#39747=CARTESIAN_POINT('Ctrl Pts',(-37.3339711607475,16.8358377670208,-3.05824914363553));
#39748=CARTESIAN_POINT('Ctrl Pts',(-37.3022443333108,16.7785464121055,-2.5));
#39749=CARTESIAN_POINT('Ctrl Pts',(-37.5745671530757,17.270335145276,-2.5));
#39750=CARTESIAN_POINT('Ctrl Pts',(-37.3224819496572,16.8422563904187,-3.05775241081752));
#39751=CARTESIAN_POINT('Ctrl Pts',(-37.2901231475283,16.7860382908692,-2.5));
#39752=CARTESIAN_POINT('Ctrl Pts',(-37.570258695808,17.2727671020922,-2.5));
#39753=CARTESIAN_POINT('Ctrl Pts',(-37.2997579173503,16.8557016280555,-3.05670968389331));
#39754=CARTESIAN_POINT('Ctrl Pts',(-37.2662411766355,16.8016967416051,-2.5));
#39755=CARTESIAN_POINT('Ctrl Pts',(-37.5617371876123,17.2778615635871,-2.5));
#39756=CARTESIAN_POINT('Ctrl Pts',(-37.2885084984505,16.8627400253605,-3.0561627663965));
#39757=CARTESIAN_POINT('Ctrl Pts',(-37.2544661462563,16.8098753233558,-2.5));
#39758=CARTESIAN_POINT('Ctrl Pts',(-37.5575186558127,17.2805285214769,-2.5));
#39759=CARTESIAN_POINT('Ctrl Pts',(-37.2335131076936,16.8990718659001,-3.05333313807168));
#39760=CARTESIAN_POINT('Ctrl Pts',(-37.1972561950466,16.8519104255022,-2.5));
#39761=CARTESIAN_POINT('Ctrl Pts',(-37.5368953730412,17.2942956929266,-2.5));
#39762=CARTESIAN_POINT('Ctrl Pts',(-37.1930113241315,16.9320140399769,-3.05074799765065));
#39763=CARTESIAN_POINT('Ctrl Pts',(-37.1558511506002,16.8897253205875,-2.5));
#39764=CARTESIAN_POINT('Ctrl Pts',(-37.5217072095524,17.3067799280439,-2.5));
#39765=CARTESIAN_POINT('Ctrl Pts',(-37.1373488654157,16.987068334806,-3.04637357495642));
#39766=CARTESIAN_POINT('Ctrl Pts',(-37.1001829683923,16.9522623708449,-2.5));
#39767=CARTESIAN_POINT('Ctrl Pts',(-37.5008337929987,17.3276482177729,-2.5));
#39768=CARTESIAN_POINT('Ctrl Pts',(-37.119649230241,17.0063667438965,-3.04483205480724));
#39769=CARTESIAN_POINT('Ctrl Pts',(-37.08275128213,16.9740145507512,-2.5));
#39770=CARTESIAN_POINT('Ctrl Pts',(-37.4941964218283,17.334963880511,-2.5));
#39771=CARTESIAN_POINT('Ctrl Pts',(-37.09862407612,17.0317074280592,-3.04279459962286));
#39772=CARTESIAN_POINT('Ctrl Pts',(-37.0623359323734,17.0024240843538,-2.5));
#39773=CARTESIAN_POINT('Ctrl Pts',(-37.4863119967309,17.344571096994,-2.5));
#39774=CARTESIAN_POINT('Ctrl Pts',(-37.0944707116322,17.0368412601703,-3.04238118958153));
#39775=CARTESIAN_POINT('Ctrl Pts',(-37.0583251973171,17.0081622414672,-2.5));
#39776=CARTESIAN_POINT('Ctrl Pts',(-37.4847544852643,17.3465174947961,-2.5));
#39777=CARTESIAN_POINT('Ctrl Pts',(-37.086318602129,17.0471765103316,-3.04154758456322));
#39778=CARTESIAN_POINT('Ctrl Pts',(-37.0504867079477,17.0196942280984,-2.5));
#39779=CARTESIAN_POINT('Ctrl Pts',(-37.4816974406886,17.350436015139,-2.5));
#39780=CARTESIAN_POINT('Ctrl Pts',(-37.0823147848581,17.0523838124048,-3.04112691976143));
#39781=CARTESIAN_POINT('Ctrl Pts',(-37.0466539524108,17.0254945229426,-2.5));
#39782=CARTESIAN_POINT('Ctrl Pts',(-37.4801960124776,17.3524103736432,-2.5));
#39783=CARTESIAN_POINT('Ctrl Pts',(-37.0705176170079,17.0681234054201,-3.03985333807572));
#39784=CARTESIAN_POINT('Ctrl Pts',(-37.0354170178543,17.0429878142689,-2.5));
#39785=CARTESIAN_POINT('Ctrl Pts',(-37.475772070005,17.3583782202939,-2.5));
#39786=CARTESIAN_POINT('Ctrl Pts',(-37.0629384235517,17.0787733000584,-3.03898884786155));
#39787=CARTESIAN_POINT('Ctrl Pts',(-37.0282631566779,17.0547884840968,-2.5));
#39788=CARTESIAN_POINT('Ctrl Pts',(-37.4729298774794,17.3624164681974,-2.5));
#39789=CARTESIAN_POINT('Ctrl Pts',(-37.026446523552,17.132793523799,-3.03458889787333));
#39790=CARTESIAN_POINT('Ctrl Pts',(-36.9942613247177,17.1142615428478,-2.5));
#39791=CARTESIAN_POINT('Ctrl Pts',(-37.4592454049732,17.3829010974121,-2.5));
#39792=CARTESIAN_POINT('Ctrl Pts',(-37.0017062809529,17.1784542255603,-3.03082304423241));
#39793=CARTESIAN_POINT('Ctrl Pts',(-36.9722499558993,17.1639506562642,-2.5));
#39794=CARTESIAN_POINT('Ctrl Pts',(-37.4499678115662,17.4002194094609,-2.5));
#39795=CARTESIAN_POINT('Ctrl Pts',(-36.9763738972329,17.2385950219028,-3.02578307239997));
#39796=CARTESIAN_POINT('Ctrl Pts',(-36.9511407639783,17.2285709769479,-2.5));
#39797=CARTESIAN_POINT('Ctrl Pts',(-37.4404681807179,17.4230360661467,-2.5));
#39798=CARTESIAN_POINT('Ctrl Pts',(-36.9715895606736,17.2507777927924,-3.02475831530062));
#39799=CARTESIAN_POINT('Ctrl Pts',(-36.9472559919366,17.2415671008265,-2.5));
#39800=CARTESIAN_POINT('Ctrl Pts',(-37.4386740479595,17.4276583514805,-2.5));
#39801=CARTESIAN_POINT('Ctrl Pts',(-36.9625961480096,17.2754584703774,-3.02267407819011));
#39802=CARTESIAN_POINT('Ctrl Pts',(-36.9401413648218,17.2677878485332,-2.5));
#39803=CARTESIAN_POINT('Ctrl Pts',(-37.4353015260892,17.4370231465561,-2.5));
#39804=CARTESIAN_POINT('Ctrl Pts',(-36.9584132845463,17.2878868497566,-3.02162045942486));
#39805=CARTESIAN_POINT('Ctrl Pts',(-36.9369311676226,17.2809375542772,-2.5));
#39806=CARTESIAN_POINT('Ctrl Pts',(-37.4337329516611,17.441739269899,-2.5));
#39807=CARTESIAN_POINT('Ctrl Pts',(-36.9468363797903,17.3252899977778,-3.01843695447992));
#39808=CARTESIAN_POINT('Ctrl Pts',(-36.9283615872827,17.3203042842923,-2.5));
#39809=CARTESIAN_POINT('Ctrl Pts',(-37.4293916024477,17.4559334232034,-2.5));
#39810=CARTESIAN_POINT('Ctrl Pts',(-36.9403896403824,17.3504426477826,-3.01627937557837));
#39811=CARTESIAN_POINT('Ctrl Pts',(-36.9240158817722,17.3465871928938,-2.5));
#39812=CARTESIAN_POINT('Ctrl Pts',(-37.4269740834161,17.4654799598295,-2.5));
#39813=CARTESIAN_POINT('Ctrl Pts',(-36.9299795767171,17.401171550854,-3.01189204818851));
#39814=CARTESIAN_POINT('Ctrl Pts',(-36.9179681053284,17.3991512563075,-2.5));
#39815=CARTESIAN_POINT('Ctrl Pts',(-37.4230703062887,17.4847366734944,-2.5));
#39816=CARTESIAN_POINT('Ctrl Pts',(-36.9260163611498,17.4267478207179,-3.0096623048872));
#39817=CARTESIAN_POINT('Ctrl Pts',(-36.9162547401427,17.4254293823291,-2.5));
#39818=CARTESIAN_POINT('Ctrl Pts',(-37.421584098594,17.4944468593896,-2.5));
#39819=CARTESIAN_POINT('Ctrl Pts',(-36.9205861826877,17.4783255467987,-3.0051277827859));
#39820=CARTESIAN_POINT('Ctrl Pts',(-36.91541973322,17.4779707405914,-2.5));
#39821=CARTESIAN_POINT('Ctrl Pts',(-37.4195477886376,17.5140317228638,-2.5));
#39822=CARTESIAN_POINT('Ctrl Pts',(-36.919118933325,17.5043343662994,-3.00282235189172));
#39823=CARTESIAN_POINT('Ctrl Pts',(-36.9162867050069,17.5042383112405,-2.5));
#39824=CARTESIAN_POINT('Ctrl Pts',(-37.4189975669682,17.5239091955899,-2.5));
#39825=CARTESIAN_POINT('Ctrl Pts',(-36.918942728626,17.5305480494939,-3.00047863991406));
#39826=CARTESIAN_POINT('Ctrl Pts',(-36.9184636408495,17.5305448701384,-2.5));
#39827=CARTESIAN_POINT('Ctrl Pts',(-37.418931489881,17.5338661095488,-2.5));
#39828=CARTESIAN_POINT('Ctrl Pts',(-38.0189154695161,17.5383073665605,-2.50000000000004));
#39829=CARTESIAN_POINT('Ctrl Pts',(-38.0189627830564,17.5323016024105,-2.50000000000007));
#39830=CARTESIAN_POINT('Ctrl Pts',(-38.0188335214001,17.526294798684,-2.5));
#39831=CARTESIAN_POINT('Ctrl Pts',(-38.0185267455263,17.5202869732672,-2.5));
#39832=CARTESIAN_POINT('Ctrl Pts',(-38.0183276500332,17.5163879346995,-2.5));
#39833=CARTESIAN_POINT('Ctrl Pts',(-38.0180536771219,17.5124884613595,-2.5));
#39834=CARTESIAN_POINT('Ctrl Pts',(-38.0177044004012,17.5085885499102,-2.5));
#39835=CARTESIAN_POINT('Ctrl Pts',(-38.0172606705395,17.5036340050864,-2.5));
#39836=CARTESIAN_POINT('Ctrl Pts',(-38.0166953474297,17.4986869761097,-2.5));
#39837=CARTESIAN_POINT('Ctrl Pts',(-38.0160139739599,17.4937821869174,-2.5));
#39838=CARTESIAN_POINT('Ctrl Pts',(-38.0158691453091,17.4927396543972,-2.5));
#39839=CARTESIAN_POINT('Ctrl Pts',(-38.0157190359243,17.4916985754705,-2.5));
#39840=CARTESIAN_POINT('Ctrl Pts',(-38.0155636624038,17.4906589455518,-2.5));
#39841=CARTESIAN_POINT('Ctrl Pts',(-38.014988053617,17.4868074519734,-2.5));
#39842=CARTESIAN_POINT('Ctrl Pts',(-38.0143402000425,17.482975834817,-2.5));
#39843=CARTESIAN_POINT('Ctrl Pts',(-38.0136209507028,17.4791638660799,-2.5));
#39844=CARTESIAN_POINT('Ctrl Pts',(-38.0106871725347,17.4636150570073,-2.5));
#39845=CARTESIAN_POINT('Ctrl Pts',(-38.0065759453709,17.4483902924033,-2.49999999999996));
#39846=CARTESIAN_POINT('Ctrl Pts',(-38.0012757977561,17.4334930688153,-2.50000000000006));
#39847=CARTESIAN_POINT('Ctrl Pts',(-37.9999753398566,17.4298378475833,-2.50000000000009));
#39848=CARTESIAN_POINT('Ctrl Pts',(-37.9986033182443,17.4262026238621,-2.50000000000007));
#39849=CARTESIAN_POINT('Ctrl Pts',(-37.9971594850432,17.4225870626251,-2.50000000000005));
#39850=CARTESIAN_POINT('Ctrl Pts',(-37.9953274844092,17.4179994755872,-2.50000000000002));
#39851=CARTESIAN_POINT('Ctrl Pts',(-37.9933788600298,17.4134438231221,-2.5));
#39852=CARTESIAN_POINT('Ctrl Pts',(-37.9913107977719,17.4089200356984,-2.5));
#39853=CARTESIAN_POINT('Ctrl Pts',(-37.9908731012467,17.407962595453,-2.5));
#39854=CARTESIAN_POINT('Ctrl Pts',(-37.9904300218038,17.4070065658388,-2.5));
#39855=CARTESIAN_POINT('Ctrl Pts',(-37.9899820161801,17.4060528984355,-2.5));
#39856=CARTESIAN_POINT('Ctrl Pts',(-37.9893718123521,17.4047539604999,-2.5));
#39857=CARTESIAN_POINT('Ctrl Pts',(-37.9887525557905,17.4034596118976,-2.5));
#39858=CARTESIAN_POINT('Ctrl Pts',(-37.9881254017715,17.4021722455759,-2.5));
#39859=CARTESIAN_POINT('Ctrl Pts',(-37.9870375902219,17.3999392822031,-2.5));
#39860=CARTESIAN_POINT('Ctrl Pts',(-37.9859245939872,17.397724152872,-2.5));
#39861=CARTESIAN_POINT('Ctrl Pts',(-37.9847866171473,17.3955265354199,-2.5));
#39862=CARTESIAN_POINT('Ctrl Pts',(-37.9820294084877,17.3902019192611,-2.5));
#39863=CARTESIAN_POINT('Ctrl Pts',(-37.9791258866422,17.3849798744598,-2.5));
#39864=CARTESIAN_POINT('Ctrl Pts',(-37.9760768589988,17.3798572660055,-2.5));
#39865=CARTESIAN_POINT('Ctrl Pts',(-37.9740918835002,17.3765223496125,-2.5));
#39866=CARTESIAN_POINT('Ctrl Pts',(-37.9720454773427,17.3732300388444,-2.5));
#39867=CARTESIAN_POINT('Ctrl Pts',(-37.9699381542059,17.3699799906587,-2.5));
#39868=CARTESIAN_POINT('Ctrl Pts',(-37.9613591254407,17.3567488651679,-2.5));
#39869=CARTESIAN_POINT('Ctrl Pts',(-37.9517779186379,17.3442130263075,-2.5));
#39870=CARTESIAN_POINT('Ctrl Pts',(-37.9411583825942,17.3323984400336,-2.5));
#39871=CARTESIAN_POINT('Ctrl Pts',(-37.9385479640711,17.3294942627961,-2.5));
#39872=CARTESIAN_POINT('Ctrl Pts',(-37.935875250628,17.3266341069194,-2.49999999999999));
#39873=CARTESIAN_POINT('Ctrl Pts',(-37.9331377938301,17.3238163249865,-2.50000000000001));
#39874=CARTESIAN_POINT('Ctrl Pts',(-37.9324072910173,17.3230643870456,-2.50000000000001));
#39875=CARTESIAN_POINT('Ctrl Pts',(-37.931672878228,17.3223162896498,-2.50000000000001));
#39876=CARTESIAN_POINT('Ctrl Pts',(-37.9309346989953,17.321572153053,-2.50000000000002));
#39877=CARTESIAN_POINT('Ctrl Pts',(-37.9281679076421,17.3187830327274,-2.50000000000006));
#39878=CARTESIAN_POINT('Ctrl Pts',(-37.9253540527131,17.3160558693812,-2.50000000000001));
#39879=CARTESIAN_POINT('Ctrl Pts',(-37.9224978903194,17.3133932168198,-2.5));
#39880=CARTESIAN_POINT('Ctrl Pts',(-37.9217364535199,17.3126833686512,-2.5));
#39881=CARTESIAN_POINT('Ctrl Pts',(-37.9209717564412,17.311977852874,-2.5));
#39882=CARTESIAN_POINT('Ctrl Pts',(-37.9202037072535,17.3112765614779,-2.5));
#39883=CARTESIAN_POINT('Ctrl Pts',(-37.9173220266189,17.3086453526081,-2.5));
#39884=CARTESIAN_POINT('Ctrl Pts',(-37.9143956775635,17.3060761773964,-2.5));
#39885=CARTESIAN_POINT('Ctrl Pts',(-37.91142514877,17.3035683556681,-2.5));
#39886=CARTESIAN_POINT('Ctrl Pts',(-37.9068726347334,17.2997249680383,-2.5));
#39887=CARTESIAN_POINT('Ctrl Pts',(-37.9022165303951,17.2960254389671,-2.5));
#39888=CARTESIAN_POINT('Ctrl Pts',(-37.8974571980587,17.2924692568552,-2.5));
#39889=CARTESIAN_POINT('Ctrl Pts',(-37.8943505147015,17.2901479371822,-2.5));
#39890=CARTESIAN_POINT('Ctrl Pts',(-37.891199835165,17.2878877196527,-2.5));
#39891=CARTESIAN_POINT('Ctrl Pts',(-37.8880052659395,17.285688454894,-2.5));
#39892=CARTESIAN_POINT('Ctrl Pts',(-37.8831125345718,17.2823201097711,-2.5));
#39893=CARTESIAN_POINT('Ctrl Pts',(-37.8781168611668,17.2790947284676,-2.5));
#39894=CARTESIAN_POINT('Ctrl Pts',(-37.8730167977921,17.2760143027342,-2.5));
#39895=CARTESIAN_POINT('Ctrl Pts',(-37.8696855682523,17.2740022482862,-2.5));
#39896=CARTESIAN_POINT('Ctrl Pts',(-37.8663097399484,17.2720520067105,-2.5));
#39897=CARTESIAN_POINT('Ctrl Pts',(-37.8628890941836,17.2701642591167,-2.5));
#39898=CARTESIAN_POINT('Ctrl Pts',(-37.861981599614,17.2696634411987,-2.5));
#39899=CARTESIAN_POINT('Ctrl Pts',(-37.8610709158903,17.2691670147014,-2.5));
#39900=CARTESIAN_POINT('Ctrl Pts',(-37.8601570499388,17.2686750119215,-2.5));
#39901=CARTESIAN_POINT('Ctrl Pts',(-37.8567118526816,17.2668202031006,-2.5));
#39902=CARTESIAN_POINT('Ctrl Pts',(-37.8532208743116,17.2650279611968,-2.5));
#39903=CARTESIAN_POINT('Ctrl Pts',(-37.8496844586753,17.2633000486829,-2.5));
#39904=CARTESIAN_POINT('Ctrl Pts',(-37.848746946163,17.2628419748114,-2.5));
#39905=CARTESIAN_POINT('Ctrl Pts',(-37.8478076846838,17.2623891308455,-2.5));
#39906=CARTESIAN_POINT('Ctrl Pts',(-37.8468667418028,17.2619415236482,-2.5));
#39907=CARTESIAN_POINT('Ctrl Pts',(-37.8433171174546,17.2602529648227,-2.5));
#39908=CARTESIAN_POINT('Ctrl Pts',(-37.8397439187893,17.2586391053616,-2.5));
#39909=CARTESIAN_POINT('Ctrl Pts',(-37.8361505179169,17.2571001416462,-2.5));
#39910=CARTESIAN_POINT('Ctrl Pts',(-37.8215612152096,17.2508519082044,-2.5));
#39911=CARTESIAN_POINT('Ctrl Pts',(-37.8066209717456,17.24581669925,-2.49999999999996));
#39912=CARTESIAN_POINT('Ctrl Pts',(-37.7913279313869,17.2419826890728,-2.50000000000007));
#39913=CARTESIAN_POINT('Ctrl Pts',(-37.7875576854708,17.2410374773377,-2.50000000000009));
#39914=CARTESIAN_POINT('Ctrl Pts',(-37.7837661046096,17.2401654107225,-2.50000000000008));
#39915=CARTESIAN_POINT('Ctrl Pts',(-37.7799532476229,17.2393662882056,-2.50000000000005));
#39916=CARTESIAN_POINT('Ctrl Pts',(-37.7751337035001,17.2383561778754,-2.50000000000002));
#39917=CARTESIAN_POINT('Ctrl Pts',(-37.7702798591916,17.2374636662302,-2.5));
#39918=CARTESIAN_POINT('Ctrl Pts',(-37.7653911781742,17.2366905233561,-2.5));
#39919=CARTESIAN_POINT('Ctrl Pts',(-37.7643715662832,17.2365292721586,-2.5));
#39920=CARTESIAN_POINT('Ctrl Pts',(-37.7633504386129,17.2363732145414,-2.5));
#39921=CARTESIAN_POINT('Ctrl Pts',(-37.7623277881001,17.2362223736589,-2.5));
#39922=CARTESIAN_POINT('Ctrl Pts',(-37.7608988179668,17.2360116006595,-2.5));
#39923=CARTESIAN_POINT('Ctrl Pts',(-37.7594668741216,17.2358110159626,-2.5));
#39924=CARTESIAN_POINT('Ctrl Pts',(-37.7580319373903,17.2356206894349,-2.5));
#39925=CARTESIAN_POINT('Ctrl Pts',(-37.7555700795487,17.2352941545819,-2.5));
#39926=CARTESIAN_POINT('Ctrl Pts',(-37.7530959436449,17.2349974558877,-2.5));
#39927=CARTESIAN_POINT('Ctrl Pts',(-37.7506223976568,17.2347323228172,-2.5));
#39928=CARTESIAN_POINT('Ctrl Pts',(-37.7495913604537,17.2346218085753,-2.5));
#39929=CARTESIAN_POINT('Ctrl Pts',(-37.7485606256491,17.2345167684412,-2.5));
#39930=CARTESIAN_POINT('Ctrl Pts',(-37.7475301924415,17.2344171850529,-2.5));
#39931=CARTESIAN_POINT('Ctrl Pts',(-37.7425867575079,17.2339394403559,-2.5));
#39932=CARTESIAN_POINT('Ctrl Pts',(-37.7376502518963,17.2335871585163,-2.5));
#39933=CARTESIAN_POINT('Ctrl Pts',(-37.732720534154,17.2333582875895,-2.5));
#39934=CARTESIAN_POINT('Ctrl Pts',(-37.7288168891892,17.233177053919,-2.5));
#39935=CARTESIAN_POINT('Ctrl Pts',(-37.7249175017295,17.2330732131101,-2.5));
#39936=CARTESIAN_POINT('Ctrl Pts',(-37.7210223229877,17.2330457357049,-2.5));
#39937=CARTESIAN_POINT('Ctrl Pts',(-37.7052413970366,17.232934413754,-2.5));
#39938=CARTESIAN_POINT('Ctrl Pts',(-37.6895290645007,17.2340676126699,-2.5));
#39939=CARTESIAN_POINT('Ctrl Pts',(-37.6738870110463,17.2364666559217,-2.5));
#39940=CARTESIAN_POINT('Ctrl Pts',(-37.6700231603601,17.2370592600157,-2.5));
#39941=CARTESIAN_POINT('Ctrl Pts',(-37.6661623118345,17.2377293485442,-2.5));
#39942=CARTESIAN_POINT('Ctrl Pts',(-37.6623080806904,17.2384764930194,-2.5));
#39943=CARTESIAN_POINT('Ctrl Pts',(-37.6612987119646,17.2386721596099,-2.50000000000001));
#39944=CARTESIAN_POINT('Ctrl Pts',(-37.660289210411,17.2388733128986,-2.50000000000001));
#39945=CARTESIAN_POINT('Ctrl Pts',(-37.6592801428124,17.2390798290796,-2.50000000000001));
#39946=CARTESIAN_POINT('Ctrl Pts',(-37.6554261020534,17.2398685986132,-2.50000000000004));
#39947=CARTESIAN_POINT('Ctrl Pts',(-37.6515701993178,17.2407376700213,-2.5));
#39948=CARTESIAN_POINT('Ctrl Pts',(-37.6477466423331,17.2416797982958,-2.5));
#39949=CARTESIAN_POINT('Ctrl Pts',(-37.6467465078848,17.2419262324266,-2.5));
#39950=CARTESIAN_POINT('Ctrl Pts',(-37.6457485236272,17.2421776330844,-2.5));
#39951=CARTESIAN_POINT('Ctrl Pts',(-37.6447527879308,17.2424339430849,-2.5));
#39952=CARTESIAN_POINT('Ctrl Pts',(-37.6409454659456,17.2434139769465,-2.5));
#39953=CARTESIAN_POINT('Ctrl Pts',(-37.6371682078251,17.2444666547528,-2.5));
#39954=CARTESIAN_POINT('Ctrl Pts',(-37.6334205438091,17.2455908476015,-2.5));
#39955=CARTESIAN_POINT('Ctrl Pts',(-37.62771375832,17.2473027212937,-2.5));
#39956=CARTESIAN_POINT('Ctrl Pts',(-37.6220754800291,17.2491801446527,-2.5));
#39957=CARTESIAN_POINT('Ctrl Pts',(-37.6165050088923,17.2512214488661,-2.5));
#39958=CARTESIAN_POINT('Ctrl Pts',(-37.6128454688109,17.2525624906566,-2.5));
#39959=CARTESIAN_POINT('Ctrl Pts',(-37.6092151764346,17.2539742724173,-2.5));
#39960=CARTESIAN_POINT('Ctrl Pts',(-37.6056139518807,17.2554563133632,-2.5));
#39961=CARTESIAN_POINT('Ctrl Pts',(-37.5965310358405,17.2591942789575,-2.5));
#39962=CARTESIAN_POINT('Ctrl Pts',(-37.5876330400573,17.2633792084384,-2.5));
#39963=CARTESIAN_POINT('Ctrl Pts',(-37.5789224592486,17.2680164179132,-2.50000000000001));
#39964=CARTESIAN_POINT('Ctrl Pts',(-37.5745670413693,17.2703350905137,-2.50000000000001));
#39965=CARTESIAN_POINT('Ctrl Pts',(-37.5702585583013,17.2727670296124,-2.50000000000002));
#39966=CARTESIAN_POINT('Ctrl Pts',(-37.5659978498847,17.2753141792429,-2.50000000000003));
#39967=CARTESIAN_POINT('Ctrl Pts',(-37.565118441144,17.2758399100439,-2.50000000000004));
#39968=CARTESIAN_POINT('Ctrl Pts',(-37.5642408341502,17.2763707385894,-2.50000000000004));
#39969=CARTESIAN_POINT('Ctrl Pts',(-37.5633654832279,17.2769063722233,-2.50000000000004));
#39970=CARTESIAN_POINT('Ctrl Pts',(-37.5599999378737,17.2789657740497,-2.50000000000006));
#39971=CARTESIAN_POINT('Ctrl Pts',(-37.5566672283182,17.2810965684525,-2.50000000000007));
#39972=CARTESIAN_POINT('Ctrl Pts',(-37.5533938832534,17.2832817819911,-2.50000000000004));
#39973=CARTESIAN_POINT('Ctrl Pts',(-37.5525431027284,17.283849744453,-2.50000000000004));
#39974=CARTESIAN_POINT('Ctrl Pts',(-37.5516958228496,17.2844216135967,-2.50000000000003));
#39975=CARTESIAN_POINT('Ctrl Pts',(-37.5508520501366,17.2849973762455,-2.50000000000002));
#39976=CARTESIAN_POINT('Ctrl Pts',(-37.5467618946436,17.2877883633497,-2.49999999999998));
#39977=CARTESIAN_POINT('Ctrl Pts',(-37.5427534964736,17.2906709132821,-2.5));
#39978=CARTESIAN_POINT('Ctrl Pts',(-37.5388261662278,17.2936446071485,-2.5));
#39979=CARTESIAN_POINT('Ctrl Pts',(-37.5309715057361,17.2995919948813,-2.5));
#39980=CARTESIAN_POINT('Ctrl Pts',(-37.5234412766274,17.3059038765257,-2.49999999999992));
#39981=CARTESIAN_POINT('Ctrl Pts',(-37.516230966746,17.312574402672,-2.50000000000008));
#39982=CARTESIAN_POINT('Ctrl Pts',(-37.513367337156,17.3152236530326,-2.50000000000014));
#39983=CARTESIAN_POINT('Ctrl Pts',(-37.5105542607098,17.3179296200831,-2.50000000000013));
#39984=CARTESIAN_POINT('Ctrl Pts',(-37.507791384449,17.3206919070763,-2.50000000000009));
#39985=CARTESIAN_POINT('Ctrl Pts',(-37.5035976368246,17.3248847602562,-2.50000000000003));
#39986=CARTESIAN_POINT('Ctrl Pts',(-37.4995203862508,17.329208307633,-2.5));
#39987=CARTESIAN_POINT('Ctrl Pts',(-37.4955614569713,17.3336646801914,-2.5));
#39988=CARTESIAN_POINT('Ctrl Pts',(-37.492952123164,17.3366018793061,-2.5));
#39989=CARTESIAN_POINT('Ctrl Pts',(-37.4903949401247,17.3395960061336,-2.5));
#39990=CARTESIAN_POINT('Ctrl Pts',(-37.4878888724731,17.3426496460838,-2.5));
#39991=CARTESIAN_POINT('Ctrl Pts',(-37.487241336329,17.3434386679754,-2.5));
#39992=CARTESIAN_POINT('Ctrl Pts',(-37.4865970049051,17.3442319721867,-2.5));
#39993=CARTESIAN_POINT('Ctrl Pts',(-37.4859565191968,17.345028757489,-2.5));
#39994=CARTESIAN_POINT('Ctrl Pts',(-37.4850374162825,17.3461721517661,-2.5));
#39995=CARTESIAN_POINT('Ctrl Pts',(-37.4841265961072,17.3473222729907,-2.5));
#39996=CARTESIAN_POINT('Ctrl Pts',(-37.4832259396789,17.3484767367919,-2.5));
#39997=CARTESIAN_POINT('Ctrl Pts',(-37.4816972641988,17.3504361970814,-2.5));
#39998=CARTESIAN_POINT('Ctrl Pts',(-37.4801959692323,17.3524104032434,-2.5));
#39999=CARTESIAN_POINT('Ctrl Pts',(-37.4787213561336,17.3543996492973,-2.5));
#40000=CARTESIAN_POINT('Ctrl Pts',(-37.478116210868,17.3552159873814,-2.5));
#40001=CARTESIAN_POINT('Ctrl Pts',(-37.4775155587945,17.3560348581811,-2.5));
#40002=CARTESIAN_POINT('Ctrl Pts',(-37.476919360215,17.3568562868653,-2.5));
#40003=CARTESIAN_POINT('Ctrl Pts',(-37.4746101165123,17.3600379097028,-2.5));
#40004=CARTESIAN_POINT('Ctrl Pts',(-37.4723682904248,17.3632571145556,-2.5));
#40005=CARTESIAN_POINT('Ctrl Pts',(-37.4701929802585,17.3665133922235,-2.5));
#40006=CARTESIAN_POINT('Ctrl Pts',(-37.4614223503606,17.3796423734205,-2.5));
#40007=CARTESIAN_POINT('Ctrl Pts',(-37.4537235445676,17.3933687395656,-2.5));
#40008=CARTESIAN_POINT('Ctrl Pts',(-37.4471007774525,17.4076943969358,-2.5));
#40009=CARTESIAN_POINT('Ctrl Pts',(-37.4454569144177,17.4112502246117,-2.5));
#40010=CARTESIAN_POINT('Ctrl Pts',(-37.4438793364595,17.414842976684,-2.5));
#40011=CARTESIAN_POINT('Ctrl Pts',(-37.4423681010022,17.4184727323592,-2.5));
#40012=CARTESIAN_POINT('Ctrl Pts',(-37.4419797097032,17.4194055886623,-2.5));
#40013=CARTESIAN_POINT('Ctrl Pts',(-37.4415957390488,17.4203409106205,-2.5));
#40014=CARTESIAN_POINT('Ctrl Pts',(-37.4412162067833,17.4212787088996,-2.5));
#40015=CARTESIAN_POINT('Ctrl Pts',(-37.4397392352041,17.4249282046903,-2.5));
#40016=CARTESIAN_POINT('Ctrl Pts',(-37.4383296884591,17.4286145658692,-2.5));
#40017=CARTESIAN_POINT('Ctrl Pts',(-37.4369877690662,17.4323407425511,-2.5));
#40018=CARTESIAN_POINT('Ctrl Pts',(-37.4366431285229,17.4332977236953,-2.5));
#40019=CARTESIAN_POINT('Ctrl Pts',(-37.4363033603984,17.4342562299466,-2.5));
#40020=CARTESIAN_POINT('Ctrl Pts',(-37.4359684866688,17.4352161447217,-2.5));
#40021=CARTESIAN_POINT('Ctrl Pts',(-37.4346652921558,17.438951748794,-2.5));
#40022=CARTESIAN_POINT('Ctrl Pts',(-37.433437206174,17.4427059852574,-2.5));
#40023=CARTESIAN_POINT('Ctrl Pts',(-37.4322857798653,17.4464706373921,-2.5));
#40024=CARTESIAN_POINT('Ctrl Pts',(-37.4305413739693,17.4521740691535,-2.5));
#40025=CARTESIAN_POINT('Ctrl Pts',(-37.4289695650201,17.4579096521343,-2.5));
#40026=CARTESIAN_POINT('Ctrl Pts',(-37.4275674674098,17.463680867276,-2.5));
#40027=CARTESIAN_POINT('Ctrl Pts',(-37.4266455315817,17.4674756744075,-2.5));
#40028=CARTESIAN_POINT('Ctrl Pts',(-37.4257972794458,17.4712848537314,-2.5));
#40029=CARTESIAN_POINT('Ctrl Pts',(-37.4250221759071,17.4751083128213,-2.5));
#40030=CARTESIAN_POINT('Ctrl Pts',(-37.4230720543668,17.4847279436923,-2.5));
#40031=CARTESIAN_POINT('Ctrl Pts',(-37.4215850091917,17.4944379732078,-2.5));
#40032=CARTESIAN_POINT('Ctrl Pts',(-37.4205659366519,17.5042392904026,-2.5));
#40033=CARTESIAN_POINT('Ctrl Pts',(-37.4199448505089,17.5102128222722,-2.5));
#40034=CARTESIAN_POINT('Ctrl Pts',(-37.4194975446597,17.516221303522,-2.5));
#40035=CARTESIAN_POINT('Ctrl Pts',(-37.4192282868926,17.5222635707283,-2.5));
#40036=CARTESIAN_POINT('Ctrl Pts',(-37.4190560419298,17.5261288263199,-2.5));
#40037=CARTESIAN_POINT('Ctrl Pts',(-37.4189571461659,17.5300000552258,-2.5));
#40038=CARTESIAN_POINT('Ctrl Pts',(-37.4189314692081,17.5338661094116,-2.5));
#40039=CARTESIAN_POINT('Ctrl Pts',(-16.9340264307573,17.163528852123,6.73969634090002));
#40040=CARTESIAN_POINT('Ctrl Pts',(-16.9457712867961,17.2557485214382,6.26075296190838));
#40041=CARTESIAN_POINT('Ctrl Pts',(-17.4245878781802,17.16390605946,6.24262002709426));
#40042=CARTESIAN_POINT('Ctrl Pts',(-16.9238487697737,17.1121753468508,6.73379116642023));
#40043=CARTESIAN_POINT('Ctrl Pts',(-16.9318068964855,17.2064962780678,6.25102883540689));
#40044=CARTESIAN_POINT('Ctrl Pts',(-17.420771254245,17.144754794966,6.23883889336594));
#40045=CARTESIAN_POINT('Ctrl Pts',(-16.9188836705717,17.0606673879271,6.72780634103384));
#40046=CARTESIAN_POINT('Ctrl Pts',(-16.9228736444101,17.1565405083055,6.24116580803177));
#40047=CARTESIAN_POINT('Ctrl Pts',(-17.4189093402838,17.1255458393,6.23504636936957));
#40048=CARTESIAN_POINT('Ctrl Pts',(-16.9189456649685,16.983243156343,6.7187202593339));
#40049=CARTESIAN_POINT('Ctrl Pts',(-16.9168638503772,17.0804387429173,6.22614064079103));
#40050=CARTESIAN_POINT('Ctrl Pts',(-17.4189325924229,17.0966716564302,6.22934558931084));
#40051=CARTESIAN_POINT('Ctrl Pts',(-16.9202265012116,16.9574044014087,6.7156730067294));
#40052=CARTESIAN_POINT('Ctrl Pts',(-16.9161095341114,17.0547943482532,6.22107753461143));
#40053=CARTESIAN_POINT('Ctrl Pts',(-17.4194128979399,17.0870354499882,6.22744306296841));
#40054=CARTESIAN_POINT('Ctrl Pts',(-16.9240802930149,16.9185992377109,6.71107449121992));
#40055=CARTESIAN_POINT('Ctrl Pts',(-16.9169275550253,17.0160227636108,6.21342265905803));
#40056=CARTESIAN_POINT('Ctrl Pts',(-17.4208580798572,17.0725635360787,6.22458579775681));
#40057=CARTESIAN_POINT('Ctrl Pts',(-16.9256893119182,16.905644695499,6.70953565876855));
#40058=CARTESIAN_POINT('Ctrl Pts',(-16.9175289419495,17.0030164596971,6.21085475684852));
#40059=CARTESIAN_POINT('Ctrl Pts',(-17.4214614628586,17.0677322859808,6.22363193892933));
#40060=CARTESIAN_POINT('Ctrl Pts',(-16.9295597285367,16.8797683534593,6.70645460032402));
#40061=CARTESIAN_POINT('Ctrl Pts',(-16.919402781573,16.9769365576265,6.20570566617719));
#40062=CARTESIAN_POINT('Ctrl Pts',(-17.4229128606045,17.0580819710591,6.22172662707637));
#40063=CARTESIAN_POINT('Ctrl Pts',(-16.9318080465975,16.8669299669448,6.70492231261218));
#40064=CARTESIAN_POINT('Ctrl Pts',(-16.9206699203638,16.9639474234362,6.20314115387546));
#40065=CARTESIAN_POINT('Ctrl Pts',(-17.4237559870977,17.0532940171532,6.2207813164412));
#40066=CARTESIAN_POINT('Ctrl Pts',(-16.9445834894833,16.8032276683107,6.69730199287355));
#40067=CARTESIAN_POINT('Ctrl Pts',(-16.928658984358,16.8990583262999,6.1903297620293));
#40068=CARTESIAN_POINT('Ctrl Pts',(-17.4285467632928,17.0295367820529,6.2160908019868));
#40069=CARTESIAN_POINT('Ctrl Pts',(-16.9596689585237,16.7538180319705,6.69133567597977));
#40070=CARTESIAN_POINT('Ctrl Pts',(-16.9402496119177,16.8481169540716,6.18027214203455));
#40071=CARTESIAN_POINT('Ctrl Pts',(-17.4342038179283,17.0111096783419,6.21245264308723));
#40072=CARTESIAN_POINT('Ctrl Pts',(-16.9845527746887,16.6939788697473,6.6840528001532));
#40073=CARTESIAN_POINT('Ctrl Pts',(-16.9613133035777,16.7857105312913,6.16795091749546));
#40074=CARTESIAN_POINT('Ctrl Pts',(-17.4435352591956,16.9887926775086,6.20804648157282));
#40075=CARTESIAN_POINT('Ctrl Pts',(-16.9898335783274,16.6821080424272,6.68260507125331));
#40076=CARTESIAN_POINT('Ctrl Pts',(-16.9658750845434,16.7732516839765,6.16549110248884));
#40077=CARTESIAN_POINT('Ctrl Pts',(-17.4455155553034,16.984365439009,6.2071723888559));
#40078=CARTESIAN_POINT('Ctrl Pts',(-17.0010129029441,16.6585634598165,6.6797280266418));
#40079=CARTESIAN_POINT('Ctrl Pts',(-16.9756875213553,16.7484542773758,6.16059522156661));
#40080=CARTESIAN_POINT('Ctrl Pts',(-17.4497078084659,16.9755844415616,6.20543871087201));
#40081=CARTESIAN_POINT('Ctrl Pts',(-17.0069205341199,16.6468728289804,6.67829663781084));
#40082=CARTESIAN_POINT('Ctrl Pts',(-16.9809474116785,16.7360985023473,6.15815575665741));
#40083=CARTESIAN_POINT('Ctrl Pts',(-17.4519231707424,16.9712243839561,6.20457788202832));
#40084=CARTESIAN_POINT('Ctrl Pts',(-17.0255319975721,16.6122139276746,6.67404499554267));
#40085=CARTESIAN_POINT('Ctrl Pts',(-16.9977536936298,16.6993085573344,6.15089212651984));
#40086=CARTESIAN_POINT('Ctrl Pts',(-17.4589024581334,16.9582981905475,6.20202579645239));
#40087=CARTESIAN_POINT('Ctrl Pts',(-17.0389887268156,16.5898976324254,6.67129663775293));
#40088=CARTESIAN_POINT('Ctrl Pts',(-17.0101778412151,16.6754791025347,6.14618735335466));
#40089=CARTESIAN_POINT('Ctrl Pts',(-17.4639487418597,16.9499751842962,6.20038254205175));
#40090=CARTESIAN_POINT('Ctrl Pts',(-17.0824066515609,16.5252426617237,6.66330736417787));
#40091=CARTESIAN_POINT('Ctrl Pts',(-17.051127346388,16.6058793480108,6.13244591192685));
#40092=CARTESIAN_POINT('Ctrl Pts',(-17.4802304556663,16.925861531581,6.19562165821438));
#40093=CARTESIAN_POINT('Ctrl Pts',(-17.1153868669716,16.4851763244393,6.65831969837799));
#40094=CARTESIAN_POINT('Ctrl Pts',(-17.0831880908469,16.5622697417389,6.12383584060727));
#40095=CARTESIAN_POINT('Ctrl Pts',(-17.4925980312227,16.9109182299925,6.19267132448229));
#40096=CARTESIAN_POINT('Ctrl Pts',(-17.1571321085461,16.443595731894,6.65311644401699));
#40097=CARTESIAN_POINT('Ctrl Pts',(-17.1247289364465,16.5166242121387,6.11482380635895));
#40098=CARTESIAN_POINT('Ctrl Pts',(-17.5082525086683,16.8954100189695,6.18960945774325));
#40099=CARTESIAN_POINT('Ctrl Pts',(-17.1618355598308,16.4390246579602,6.6525440228328));
#40100=CARTESIAN_POINT('Ctrl Pts',(-17.1294344256378,16.5115867952363,6.11382924294728));
#40101=CARTESIAN_POINT('Ctrl Pts',(-17.5100163000558,16.8937051501344,6.18927285662447));
#40102=CARTESIAN_POINT('Ctrl Pts',(-17.171374097915,16.4299815745484,6.65141081135807));
#40103=CARTESIAN_POINT('Ctrl Pts',(-17.1390037634447,16.5016077877741,6.11185903561698));
#40104=CARTESIAN_POINT('Ctrl Pts',(-17.5135932548913,16.8903323645726,6.18860695003381));
#40105=CARTESIAN_POINT('Ctrl Pts',(-17.1762161790489,16.425503359408,6.65084924015553));
#40106=CARTESIAN_POINT('Ctrl Pts',(-17.1438746821593,16.4966594486413,6.11088205929252));
#40107=CARTESIAN_POINT('Ctrl Pts',(-17.5154090352215,16.8886621272269,6.18827718639005));
#40108=CARTESIAN_POINT('Ctrl Pts',(-17.190879548413,16.4122753689571,6.64918933918175));
#40109=CARTESIAN_POINT('Ctrl Pts',(-17.1586695817608,16.4820186331741,6.10799144696816));
#40110=CARTESIAN_POINT('Ctrl Pts',(-17.5209077944372,16.8837284797184,6.18730311070934));
#40111=CARTESIAN_POINT('Ctrl Pts',(-17.2008371206551,16.4037311294511,6.64811568767107));
#40112=CARTESIAN_POINT('Ctrl Pts',(-17.1687645001098,16.4725403371964,6.10612009770977));
#40113=CARTESIAN_POINT('Ctrl Pts',(-17.5246418887157,16.8805417313108,6.18667393440136));
#40114=CARTESIAN_POINT('Ctrl Pts',(-17.2312453506019,16.3789058423747,6.64499241842953));
#40115=CARTESIAN_POINT('Ctrl Pts',(-17.1997603324787,16.4449156410009,6.100666010302));
#40116=CARTESIAN_POINT('Ctrl Pts',(-17.5360449694744,16.8712825880367,6.18484585360074));
#40117=CARTESIAN_POINT('Ctrl Pts',(-17.2522302391352,16.3634303224513,6.64304026443391));
#40118=CARTESIAN_POINT('Ctrl Pts',(-17.2213294853766,16.4276216694408,6.09725157157484));
#40119=CARTESIAN_POINT('Ctrl Pts',(-17.5439143065422,16.8655106243265,6.18370626479344));
#40120=CARTESIAN_POINT('Ctrl Pts',(-17.2956019395641,16.3345930464113,6.63939537781673));
#40121=CARTESIAN_POINT('Ctrl Pts',(-17.2662656597083,16.3952572162235,6.09086168929334));
#40122=CARTESIAN_POINT('Ctrl Pts',(-17.5601786937626,16.8547550179788,6.18158272950716));
#40123=CARTESIAN_POINT('Ctrl Pts',(-17.3179887637184,16.3212313140015,6.63770263755943));
#40124=CARTESIAN_POINT('Ctrl Pts',(-17.2896291828443,16.3801970928505,6.08788829082891));
#40125=CARTESIAN_POINT('Ctrl Pts',(-17.5685737507052,16.8497713855231,6.18059878503843));
#40126=CARTESIAN_POINT('Ctrl Pts',(-17.3526333624528,16.3027934739649,6.63536298725943));
#40127=CARTESIAN_POINT('Ctrl Pts',(-17.3260026650614,16.3593493456032,6.08377221168955));
#40128=CARTESIAN_POINT('Ctrl Pts',(-17.5815654787338,16.8428944620486,6.17924103827948));
#40129=CARTESIAN_POINT('Ctrl Pts',(-17.364359267792,16.296915463442,6.63461640073939));
#40130=CARTESIAN_POINT('Ctrl Pts',(-17.3383566078206,16.3526877545169,6.08245697912365));
#40131=CARTESIAN_POINT('Ctrl Pts',(-17.5859626904173,16.8407020762296,6.17880818414767));
#40132=CARTESIAN_POINT('Ctrl Pts',(-17.3822192836592,16.2885072643732,6.6335476194421));
#40133=CARTESIAN_POINT('Ctrl Pts',(-17.3572223204219,16.3431449083558,6.08057288538689));
#40134=CARTESIAN_POINT('Ctrl Pts',(-17.5926601988439,16.8375659857744,6.17818900950262));
#40135=CARTESIAN_POINT('Ctrl Pts',(-17.3882178337638,16.285772701414,6.63319987789834));
#40136=CARTESIAN_POINT('Ctrl Pts',(-17.3635686188785,16.3400380551801,6.07995948320997));
#40137=CARTESIAN_POINT('Ctrl Pts',(-17.5949096533811,16.8365460418669,6.17798763667366));
#40138=CARTESIAN_POINT('Ctrl Pts',(-17.4003064009864,16.2804414700918,6.6325216769544));
#40139=CARTESIAN_POINT('Ctrl Pts',(-17.3763747964082,16.3339762671101,6.07876267287232));
#40140=CARTESIAN_POINT('Ctrl Pts',(-17.5994428679428,16.8345575960637,6.17759504747957));
#40141=CARTESIAN_POINT('Ctrl Pts',(-17.4064014619839,16.2778429556048,6.63219098038768));
#40142=CARTESIAN_POINT('Ctrl Pts',(-17.3828399484087,16.3310193192068,6.07817886727278));
#40143=CARTESIAN_POINT('Ctrl Pts',(-17.6017285156952,16.8335883975106,6.17740369356977));
#40144=CARTESIAN_POINT('Ctrl Pts',(-17.4613673391331,16.2552073371804,6.6293092707837));
#40145=CARTESIAN_POINT('Ctrl Pts',(-17.4412943532773,16.305207075037,6.07308262169252));
#40146=CARTESIAN_POINT('Ctrl Pts',(-17.6223407123812,16.8251457010694,6.17573680811258));
#40147=CARTESIAN_POINT('Ctrl Pts',(-17.5114824250486,16.2401548090555,6.62738600694331));
#40148=CARTESIAN_POINT('Ctrl Pts',(-17.4949832638486,16.2879639917577,6.06967823010323));
#40149=CARTESIAN_POINT('Ctrl Pts',(-17.6411338750825,16.8195313396363,6.17462833554231));
#40150=CARTESIAN_POINT('Ctrl Pts',(-17.5884810370651,16.2249404862174,6.62544067878907));
#40151=CARTESIAN_POINT('Ctrl Pts',(-17.5778953266643,16.270488978075,6.06622804728844));
#40152=CARTESIAN_POINT('Ctrl Pts',(-17.6700083560242,16.8138566171136,6.17350794556827));
#40153=CARTESIAN_POINT('Ctrl Pts',(-17.61445379365,16.2211054438284,6.6249498806517));
#40154=CARTESIAN_POINT('Ctrl Pts',(-17.6059331605785,16.2660757431219,6.06535671936452));
#40155=CARTESIAN_POINT('Ctrl Pts',(-17.6797481384879,16.8124261864561,6.17322552820585));
#40156=CARTESIAN_POINT('Ctrl Pts',(-17.6538857988551,16.217259998137,6.62445766257136));
#40157=CARTESIAN_POINT('Ctrl Pts',(-17.6485546296303,16.2616476106312,6.06448245014227));
#40158=CARTESIAN_POINT('Ctrl Pts',(-17.6945351416054,16.8109918968226,6.17294234894575));
#40159=CARTESIAN_POINT('Ctrl Pts',(-17.6671432193907,16.2162960247729,6.6243342451152));
#40160=CARTESIAN_POINT('Ctrl Pts',(-17.6628934486627,16.2605370299517,6.06426318242413));
#40161=CARTESIAN_POINT('Ctrl Pts',(-17.6995066741152,16.810632347174,6.1728713611891));
#40162=CARTESIAN_POINT('Ctrl Pts',(-17.6935540371893,16.2150298143844,6.62417212417057));
#40163=CARTESIAN_POINT('Ctrl Pts',(-17.691468213857,16.2590779435578,6.06397510741069));
#40164=CARTESIAN_POINT('Ctrl Pts',(-17.7094107303948,16.8101600586753,6.17277811481509));
#40165=CARTESIAN_POINT('Ctrl Pts',(-17.7067266210675,16.2147239146772,6.62413295366647));
#40166=CARTESIAN_POINT('Ctrl Pts',(-17.7057234775305,16.2587254085436,6.06390550458979));
#40167=CARTESIAN_POINT('Ctrl Pts',(-17.7143504495434,16.8100459686567,6.1727555894295));
#40168=CARTESIAN_POINT('Ctrl Pts',(-17.7724284272708,16.2148007635293,6.6241427921321));
#40169=CARTESIAN_POINT('Ctrl Pts',(-17.7768280969853,16.2588139364961,6.06392298312376));
#40170=CARTESIAN_POINT('Ctrl Pts',(-17.7389886268855,16.8100746189498,6.17276124600583));
#40171=CARTESIAN_POINT('Ctrl Pts',(-17.8244788813812,16.2199564028495,6.62480342778294));
#40172=CARTESIAN_POINT('Ctrl Pts',(-17.8331128420917,16.2647554475499,6.06509604654469));
#40173=CARTESIAN_POINT('Ctrl Pts',(-17.7585075492867,16.8119976109921,6.17314091232356));
#40174=CARTESIAN_POINT('Ctrl Pts',(-17.8889031485325,16.2327695523612,6.62644171019872));
#40175=CARTESIAN_POINT('Ctrl Pts',(-17.90254892953,16.2794864647711,6.06800446787037));
#40176=CARTESIAN_POINT('Ctrl Pts',(-17.7826666468153,16.816776749508,6.17408448249046));
#40177=CARTESIAN_POINT('Ctrl Pts',(-17.9017557691567,16.2356534961519,6.62681033151498));
#40178=CARTESIAN_POINT('Ctrl Pts',(-17.9163762099596,16.2827975605751,6.06865819473137));
#40179=CARTESIAN_POINT('Ctrl Pts',(-17.7874863810826,16.81785241274,6.1742968562754));
#40180=CARTESIAN_POINT('Ctrl Pts',(-17.9273953632276,16.2420759339317,6.62763082558797));
#40181=CARTESIAN_POINT('Ctrl Pts',(-17.9439205439042,16.2901643089726,6.07011265017177));
#40182=CARTESIAN_POINT('Ctrl Pts',(-17.797101226854,16.82024789507,6.17476980880739));
#40183=CARTESIAN_POINT('Ctrl Pts',(-17.9401902056257,16.2456190784938,6.62808328938417));
#40184=CARTESIAN_POINT('Ctrl Pts',(-17.9576446533942,16.294224513599,6.07091427748269));
#40185=CARTESIAN_POINT('Ctrl Pts',(-17.8018992926118,16.8215694340713,6.17503072712393));
#40186=CARTESIAN_POINT('Ctrl Pts',(-17.9780466892305,16.2571128882123,6.62955018787334));
#40187=CARTESIAN_POINT('Ctrl Pts',(-17.9981679747951,16.3073767581212,6.07351099350535));
#40188=CARTESIAN_POINT('Ctrl Pts',(-17.8160954773958,16.8258564334959,6.17587713171108));
#40189=CARTESIAN_POINT('Ctrl Pts',(-18.0027258637711,16.2659587403489,6.63067809312904));
#40190=CARTESIAN_POINT('Ctrl Pts',(-18.0244924260245,16.317478878484,6.07550550765576));
#40191=CARTESIAN_POINT('Ctrl Pts',(-17.825350164657,16.8291557994221,6.17652854268134));
#40192=CARTESIAN_POINT('Ctrl Pts',(-18.0751331263037,16.2959506337827,6.63449608491444));
#40193=CARTESIAN_POINT('Ctrl Pts',(-18.1013159720922,16.3516027063543,6.08224275242306));
#40194=CARTESIAN_POINT('Ctrl Pts',(-17.852502890817,16.8403422289135,6.17873713762098));
#40195=CARTESIAN_POINT('Ctrl Pts',(-18.1212467327399,16.3205175212379,6.63761658916437));
#40196=CARTESIAN_POINT('Ctrl Pts',(-18.1497601127687,16.3794086658638,6.0877326275894));
#40197=CARTESIAN_POINT('Ctrl Pts',(-17.8697955008785,16.8495051762018,6.18054622594794));
#40198=CARTESIAN_POINT('Ctrl Pts',(-18.1706160636699,16.3534706885993,6.6417813765152));
#40199=CARTESIAN_POINT('Ctrl Pts',(-18.2009972681976,16.4164599843371,6.09504786204832));
#40200=CARTESIAN_POINT('Ctrl Pts',(-17.8883089893406,16.8617959232122,6.18297285203741));
#40201=CARTESIAN_POINT('Ctrl Pts',(-18.1760670536863,16.3572075290665,6.64225340483513));
#40202=CARTESIAN_POINT('Ctrl Pts',(-18.2066322253776,16.4206486705888,6.09587485615456));
#40203=CARTESIAN_POINT('Ctrl Pts',(-17.8903531105129,16.863189672331,6.18324802717289));
#40204=CARTESIAN_POINT('Ctrl Pts',(-18.1868377701863,16.3647884998207,6.64321046159106));
#40205=CARTESIAN_POINT('Ctrl Pts',(-18.2177440408947,16.4291367290659,6.09755069767437));
#40206=CARTESIAN_POINT('Ctrl Pts',(-17.8943921317318,16.8660171798007,6.18380627667459));
#40207=CARTESIAN_POINT('Ctrl Pts',(-18.1921652410117,16.3686376965469,6.64369613249193));
#40208=CARTESIAN_POINT('Ctrl Pts',(-18.2232288896621,16.4334416698043,6.09840064450838));
#40209=CARTESIAN_POINT('Ctrl Pts',(-17.8963899309271,16.8674528346187,6.18408972547016));
#40210=CARTESIAN_POINT('Ctrl Pts',(-18.2079758853082,16.380359521441,6.64517424754474));
#40211=CARTESIAN_POINT('Ctrl Pts',(-18.2394674114616,16.4465321648978,6.10098516902028));
#40212=CARTESIAN_POINT('Ctrl Pts',(-17.902318925834,16.8718247643677,6.18495289829289));
#40213=CARTESIAN_POINT('Ctrl Pts',(-18.2182873888224,16.3884062672933,6.64618778634462));
#40214=CARTESIAN_POINT('Ctrl Pts',(-18.250014828929,16.4555003709746,6.10275580857727));
#40215=CARTESIAN_POINT('Ctrl Pts',(-17.9061857359879,16.8748259873231,6.18554544534619));
#40216=CARTESIAN_POINT('Ctrl Pts',(-18.2485461467234,16.4132319441657,6.6493107176117));
#40217=CARTESIAN_POINT('Ctrl Pts',(-18.2808046004885,16.4830834508249,6.10820167945361));
#40218=CARTESIAN_POINT('Ctrl Pts',(-17.917532774601,16.884085261647,6.18737355202065));
#40219=CARTESIAN_POINT('Ctrl Pts',(-18.2678192302634,16.4306946934602,6.65150224599118));
#40220=CARTESIAN_POINT('Ctrl Pts',(-18.3002353052696,16.5024028462849,6.11201600815278));
#40221=CARTESIAN_POINT('Ctrl Pts',(-17.9247601784908,16.8905983462382,6.18865946417705));
#40222=CARTESIAN_POINT('Ctrl Pts',(-18.304585320563,16.4674258171909,6.65609825686814));
#40223=CARTESIAN_POINT('Ctrl Pts',(-18.3369000788844,16.5428190986578,6.11999559900783));
#40224=CARTESIAN_POINT('Ctrl Pts',(-17.9385474613616,16.9042978717687,6.19136423273484));
#40225=CARTESIAN_POINT('Ctrl Pts',(-18.32207835827,16.4866941560064,6.65850274672427));
#40226=CARTESIAN_POINT('Ctrl Pts',(-18.3541350222299,16.5639050113827,6.12415870039582));
#40227=CARTESIAN_POINT('Ctrl Pts',(-17.9451073556682,16.9114842972485,6.19278308608398));
#40228=CARTESIAN_POINT('Ctrl Pts',(-18.3469582555341,16.5169758809527,6.6622690907101));
#40229=CARTESIAN_POINT('Ctrl Pts',(-18.3783360711151,16.5968717741023,6.13066749977414));
#40230=CARTESIAN_POINT('Ctrl Pts',(-17.9544373101362,16.9227782767883,6.1950129151889));
#40231=CARTESIAN_POINT('Ctrl Pts',(-18.3550268290823,16.5273031516405,6.66355157018222));
#40232=CARTESIAN_POINT('Ctrl Pts',(-18.3861205298441,16.6080723020181,6.13287887823903));
#40233=CARTESIAN_POINT('Ctrl Pts',(-17.9574630272311,16.9266299573578,6.19577337251102));
#40234=CARTESIAN_POINT('Ctrl Pts',(-18.3706915223259,16.5484153134749,6.66616886023153));
#40235=CARTESIAN_POINT('Ctrl Pts',(-18.4011144492354,16.6308981776041,6.13738550954182));
#40236=CARTESIAN_POINT('Ctrl Pts',(-17.9633372878401,16.934503971749,6.19732798011414));
#40237=CARTESIAN_POINT('Ctrl Pts',(-18.3782309891514,16.5591238170816,6.66749420161781));
#40238=CARTESIAN_POINT('Ctrl Pts',(-18.4082702147513,16.6424396756498,6.13966420751237));
#40239=CARTESIAN_POINT('Ctrl Pts',(-17.9661645847443,16.9384978169065,6.19811650573006));
#40240=CARTESIAN_POINT('Ctrl Pts',(-18.4144652239087,16.6133698763481,6.67419609590586));
#40241=CARTESIAN_POINT('Ctrl Pts',(-18.4422698693699,16.7005708871118,6.15114135485145));
#40242=CARTESIAN_POINT('Ctrl Pts',(-17.9797524369468,16.9587293525346,6.20211092300537));
#40243=CARTESIAN_POINT('Ctrl Pts',(-18.4388454391431,16.6590429087733,6.67980148969806));
#40244=CARTESIAN_POINT('Ctrl Pts',(-18.4642277040733,16.7490077862942,6.16070450371041));
#40245=CARTESIAN_POINT('Ctrl Pts',(-17.9888950132745,16.975763316277,6.20547402703715));
#40246=CARTESIAN_POINT('Ctrl Pts',(-18.4636539969267,16.7189339970101,6.68708985334279));
#40247=CARTESIAN_POINT('Ctrl Pts',(-18.4853233274594,16.811806410725,6.17310316266067));
#40248=CARTESIAN_POINT('Ctrl Pts',(-17.9981982137564,16.9980996869273,6.20988401283525));
#40249=CARTESIAN_POINT('Ctrl Pts',(-18.4683298236966,16.7310534611065,6.68856175184365));
#40250=CARTESIAN_POINT('Ctrl Pts',(-18.4892098083346,16.8244336013383,6.17559621456002));
#40251=CARTESIAN_POINT('Ctrl Pts',(-17.9999516535622,17.0026196231967,6.21077640735487));
#40252=CARTESIAN_POINT('Ctrl Pts',(-18.4771016880877,16.7555788545222,6.69153398968095));
#40253=CARTESIAN_POINT('Ctrl Pts',(-18.4963362162636,16.8498937457125,6.18062294324687));
#40254=CARTESIAN_POINT('Ctrl Pts',(-18.0032410966494,17.0117663114213,6.21258228557033));
#40255=CARTESIAN_POINT('Ctrl Pts',(-18.4812032176816,16.768003161379,6.69303654757409));
#40256=CARTESIAN_POINT('Ctrl Pts',(-18.4995813969772,16.8627446305905,6.18316016026802));
#40257=CARTESIAN_POINT('Ctrl Pts',(-18.0047791706222,17.0163999130041,6.21349712162379));
#40258=CARTESIAN_POINT('Ctrl Pts',(-18.4925821723103,16.8055904468549,6.69757219653477));
#40259=CARTESIAN_POINT('Ctrl Pts',(-18.5082993306589,16.9014403837458,6.19080006401661));
#40260=CARTESIAN_POINT('Ctrl Pts',(-18.0090462865719,17.030417917443,6.21626476912844));
#40261=CARTESIAN_POINT('Ctrl Pts',(-18.4988883625265,16.8308948943173,6.70061244451219));
#40262=CARTESIAN_POINT('Ctrl Pts',(-18.5127456724536,16.9273229004005,6.19591018385897));
#40263=CARTESIAN_POINT('Ctrl Pts',(-18.0114111023906,17.0398550445677,6.21812799020613));
#40264=CARTESIAN_POINT('Ctrl Pts',(-18.5089809331914,16.8819886542203,6.70672283022605));
#40265=CARTESIAN_POINT('Ctrl Pts',(-18.5189743166287,16.979189821447,6.20615053976939));
#40266=CARTESIAN_POINT('Ctrl Pts',(-18.0151958167961,17.0589100232433,6.22189011372466));
#40267=CARTESIAN_POINT('Ctrl Pts',(-18.5127673002267,16.9077779664103,6.70979297341625));
#40268=CARTESIAN_POINT('Ctrl Pts',(-18.5207667892184,17.0051710504343,6.21128014890083));
#40269=CARTESIAN_POINT('Ctrl Pts',(-18.0166157093195,17.0685278759537,6.22378901639444));
#40270=CARTESIAN_POINT('Ctrl Pts',(-18.51653149759,16.9468304737568,6.71441949514766));
#40271=CARTESIAN_POINT('Ctrl Pts',(-18.5214756795303,17.0442515895124,6.21899602293492));
#40272=CARTESIAN_POINT('Ctrl Pts',(-18.0180272756984,17.0830920314624,6.22666449334457));
#40273=CARTESIAN_POINT('Ctrl Pts',(-18.5174610536025,16.9598642331123,6.71595985693076));
#40274=CARTESIAN_POINT('Ctrl Pts',(-18.5213812087045,17.0572310011096,6.22155861565454));
#40275=CARTESIAN_POINT('Ctrl Pts',(-18.0183758583191,17.0879528012551,6.22762418039891));
#40276=CARTESIAN_POINT('Ctrl Pts',(-18.5186722537819,16.9858429775025,6.71902258829226));
#40277=CARTESIAN_POINT('Ctrl Pts',(-18.5205481857505,17.0830017716537,6.22664667288122));
#40278=CARTESIAN_POINT('Ctrl Pts',(-18.0188300652425,17.0976412129467,6.22953701389521));
#40279=CARTESIAN_POINT('Ctrl Pts',(-18.5189557766232,16.9988067822409,6.7205471885435));
#40280=CARTESIAN_POINT('Ctrl Pts',(-18.5198112791957,17.0958122032461,6.22917590299987));
#40281=CARTESIAN_POINT('Ctrl Pts',(-18.0189363807851,17.1024758738013,6.23049154612614));
#40282=CARTESIAN_POINT('Ctrl Pts',(-18.5187872011184,17.0634999017462,6.72813660661715));
#40283=CARTESIAN_POINT('Ctrl Pts',(-18.5145769287806,17.1593013447143,6.24171089431925));
#40284=CARTESIAN_POINT('Ctrl Pts',(-18.0188731754452,17.1266021766945,6.23525492755391));
#40285=CARTESIAN_POINT('Ctrl Pts',(-18.5136215290469,17.1148550403912,6.73410108134611));
#40286=CARTESIAN_POINT('Ctrl Pts',(-18.5054607669974,17.2090806073982,6.25153907298411));
#40287=CARTESIAN_POINT('Ctrl Pts',(-18.0169360523498,17.1457541379813,6.23903619885366));
#40288=CARTESIAN_POINT('Ctrl Pts',(-18.5008049385582,17.178543935026,6.74142244098528));
#40289=CARTESIAN_POINT('Ctrl Pts',(-18.4879750956344,17.2700726310465,6.26358104534826));
#40290=CARTESIAN_POINT('Ctrl Pts',(-18.0121298155278,17.1695056335805,6.24372558012852));
#40291=CARTESIAN_POINT('Ctrl Pts',(-18.4979208133035,17.1912562328885,6.74287997549926));
#40292=CARTESIAN_POINT('Ctrl Pts',(-18.4841868810595,17.2821639022754,6.26596828789697));
#40293=CARTESIAN_POINT('Ctrl Pts',(-18.0110482760138,17.1742464268863,6.24466157960121));
#40294=CARTESIAN_POINT('Ctrl Pts',(-18.4914973495927,17.2166287983916,6.74578145608233));
#40295=CARTESIAN_POINT('Ctrl Pts',(-18.4759981394833,17.3062060478485,6.27071505370745));
#40296=CARTESIAN_POINT('Ctrl Pts',(-18.0086394683647,17.1837085953516,6.24652974472097));
#40297=CARTESIAN_POINT('Ctrl Pts',(-18.4879753251126,17.2292171975606,6.74721717444261));
#40298=CARTESIAN_POINT('Ctrl Pts',(-18.4716211015665,17.3180893500614,6.27306123585199));
#40299=CARTESIAN_POINT('Ctrl Pts',(-18.0073187104683,17.1884031726981,6.24745661953651));
#40300=CARTESIAN_POINT('Ctrl Pts',(-18.4765353931923,17.2665465103297,6.75146357848355));
#40301=CARTESIAN_POINT('Ctrl Pts',(-18.4577271501903,17.3531629274733,6.27998599460963));
#40302=CARTESIAN_POINT('Ctrl Pts',(-18.0030287452838,17.2023243430448,6.25020514858282));
#40303=CARTESIAN_POINT('Ctrl Pts',(-18.4677297456344,17.2909162449736,6.75422091139731));
#40304=CARTESIAN_POINT('Ctrl Pts',(-18.4474068235007,17.3759132514684,6.28447770936899));
#40305=CARTESIAN_POINT('Ctrl Pts',(-17.9997266201643,17.2114124977806,6.25199947022725));
#40306=CARTESIAN_POINT('Ctrl Pts',(-18.4378487844442,17.3625079863937,6.76228026019661));
#40307=CARTESIAN_POINT('Ctrl Pts',(-18.4134691558281,17.4421491186173,6.29755500102144));
#40308=CARTESIAN_POINT('Ctrl Pts',(-17.9885212630024,17.2381110500616,6.25727070422638));
#40309=CARTESIAN_POINT('Ctrl Pts',(-18.413342249397,17.4082296127105,6.76737146292247));
#40310=CARTESIAN_POINT('Ctrl Pts',(-18.3868137642132,17.483931249389,6.30580426435083));
#40311=CARTESIAN_POINT('Ctrl Pts',(-17.979331323364,17.2551619032087,6.26063714282115));
#40312=CARTESIAN_POINT('Ctrl Pts',(-18.3693951615143,17.4736551525738,6.77458729194665));
#40313=CARTESIAN_POINT('Ctrl Pts',(-18.3405991802905,17.5430486220348,6.31747611462008));
#40314=CARTESIAN_POINT('Ctrl Pts',(-17.9628511456172,17.279560906992,6.26545436500358));
#40315=CARTESIAN_POINT('Ctrl Pts',(-18.3537632469114,17.4945975063259,6.77688492238546));
#40316=CARTESIAN_POINT('Ctrl Pts',(-18.3244286783927,17.5618163081471,6.32118151647404));
#40317=CARTESIAN_POINT('Ctrl Pts',(-17.9569891815114,17.2873709068913,6.26699633389272));
#40318=CARTESIAN_POINT('Ctrl Pts',(-18.3206591277799,17.5347184100098,6.78126667754031));
#40319=CARTESIAN_POINT('Ctrl Pts',(-18.2906282613387,17.5975559035035,6.32823777061752));
#40320=CARTESIAN_POINT('Ctrl Pts',(-17.9445751422903,17.3023331556006,6.26995040845338));
#40321=CARTESIAN_POINT('Ctrl Pts',(-18.3031766385638,17.5539118752031,6.78335243318941));
#40322=CARTESIAN_POINT('Ctrl Pts',(-18.2729880315817,17.6145513152006,6.33159326311853));
#40323=CARTESIAN_POINT('Ctrl Pts',(-17.9380192073362,17.3094909634119,6.27136361166745));
#40324=CARTESIAN_POINT('Ctrl Pts',(-18.2663596953146,17.590573120573,6.78731950209393));
#40325=CARTESIAN_POINT('Ctrl Pts',(-18.2362359266378,17.6468363652653,6.33796746842275));
#40326=CARTESIAN_POINT('Ctrl Pts',(-17.9242128511607,17.3231630449985,6.2740629618247));
#40327=CARTESIAN_POINT('Ctrl Pts',(-18.2470253297619,17.6080409781332,6.78920081264864));
#40328=CARTESIAN_POINT('Ctrl Pts',(-18.2171237375768,17.6621351487866,6.3409879868012));
#40329=CARTESIAN_POINT('Ctrl Pts',(-17.9169624698265,17.3296773557345,6.27534911606522));
#40330=CARTESIAN_POINT('Ctrl Pts',(-18.2166010903152,17.6329170950227,6.79186951328928));
#40331=CARTESIAN_POINT('Ctrl Pts',(-18.1872989485619,17.683828532514,6.34527102434781));
#40332=CARTESIAN_POINT('Ctrl Pts',(-17.9055533732547,17.3389544402554,6.27718073909949));
#40333=CARTESIAN_POINT('Ctrl Pts',(-18.2062168750825,17.6409916724233,6.79273390499216));
#40334=CARTESIAN_POINT('Ctrl Pts',(-18.1771687996823,17.6908479022576,6.34665689501433));
#40335=CARTESIAN_POINT('Ctrl Pts',(-17.9016592934025,17.3419657104848,6.27777526983833));
#40336=CARTESIAN_POINT('Ctrl Pts',(-18.1849835178449,17.656672005178,6.79440927725295));
#40337=CARTESIAN_POINT('Ctrl Pts',(-18.1565384222284,17.7044471017748,6.34934185568567));
#40338=CARTESIAN_POINT('Ctrl Pts',(-17.8936967872377,17.3478134207786,6.27892981368751));
#40339=CARTESIAN_POINT('Ctrl Pts',(-18.1742117514745,17.6642209160496,6.79521418404731));
#40340=CARTESIAN_POINT('Ctrl Pts',(-18.1461128939455,17.7109787537895,6.35063143370503));
#40341=CARTESIAN_POINT('Ctrl Pts',(-17.8896573717566,17.3506286544074,6.27948563990098));
#40342=CARTESIAN_POINT('Ctrl Pts',(-18.1196129973381,17.7005236924937,6.7990781174034));
#40343=CARTESIAN_POINT('Ctrl Pts',(-18.0935526247991,17.7422665507531,6.35680874614416));
#40344=CARTESIAN_POINT('Ctrl Pts',(-17.8691828474184,17.3641671857882,6.2821586225467));
#40345=CARTESIAN_POINT('Ctrl Pts',(-18.073566038191,17.7250092175285,6.8016618385873));
#40346=CARTESIAN_POINT('Ctrl Pts',(-18.0497217046225,17.7632251779753,6.36094671689349));
#40347=CARTESIAN_POINT('Ctrl Pts',(-17.8519152345038,17.3732987063331,6.2839615061283));
#40348=CARTESIAN_POINT('Ctrl Pts',(-18.0130701585827,17.7499642230801,6.80428434438707));
#40349=CARTESIAN_POINT('Ctrl Pts',(-17.9926453915806,17.7844819967742,6.36514356115633));
#40350=CARTESIAN_POINT('Ctrl Pts',(-17.8292292752308,17.3826053354479,6.28579896230536));
#40351=CARTESIAN_POINT('Ctrl Pts',(-18.0008227990897,17.7546700742571,6.80477818859267));
#40352=CARTESIAN_POINT('Ctrl Pts',(-17.9811297306172,17.7884796711135,6.36593284278751));
#40353=CARTESIAN_POINT('Ctrl Pts',(-17.8246365175473,17.3843603279786,6.28614545960597));
#40354=CARTESIAN_POINT('Ctrl Pts',(-17.9760268452319,17.7635021372388,6.80570402970065));
#40355=CARTESIAN_POINT('Ctrl Pts',(-17.9578627436139,17.7959726092415,6.36741221252255));
#40356=CARTESIAN_POINT('Ctrl Pts',(-17.8153380323659,17.3876541288755,6.28679577184356));
#40357=CARTESIAN_POINT('Ctrl Pts',(-17.9634548231814,17.7676353220123,6.80613675524105));
#40358=CARTESIAN_POINT('Ctrl Pts',(-17.9460886325703,17.7994744891973,6.36810360689066));
#40359=CARTESIAN_POINT('Ctrl Pts',(-17.8106235240595,17.3891955494437,6.28710010252115));
#40360=CARTESIAN_POINT('Ctrl Pts',(-17.9254344120959,17.7790973746866,6.80733565050496));
#40361=CARTESIAN_POINT('Ctrl Pts',(-17.9105547741728,17.8091716890774,6.37001817548471));
#40362=CARTESIAN_POINT('Ctrl Pts',(-17.7963658737417,17.3934701994542,6.28794406889925));
#40363=CARTESIAN_POINT('Ctrl Pts',(-17.8999087430931,17.7854283478246,6.80799626184293));
#40364=CARTESIAN_POINT('Ctrl Pts',(-17.886766663715,17.8145173455381,6.37107359623513));
#40365=CARTESIAN_POINT('Ctrl Pts',(-17.7867937446671,17.3958312544259,6.28841022425892));
#40366=CARTESIAN_POINT('Ctrl Pts',(-17.8228126864582,17.8006160211639,6.80957942969772));
#40367=CARTESIAN_POINT('Ctrl Pts',(-17.8151219476809,17.8273163816643,6.37360057648762));
#40368=CARTESIAN_POINT('Ctrl Pts',(-17.7578827253461,17.4014953443393,6.28952851498163));
#40369=CARTESIAN_POINT('Ctrl Pts',(-17.7707282072719,17.8057036316249,6.81010758629701));
#40370=CARTESIAN_POINT('Ctrl Pts',(-17.7668735570122,17.8315930628393,6.37444494388912));
#40371=CARTESIAN_POINT('Ctrl Pts',(-17.7383510443547,17.4033927296949,6.28990312563806));
#40372=CARTESIAN_POINT('Ctrl Pts',(-17.7113425373793,17.8056309224566,6.81010002580354));
#40373=CARTESIAN_POINT('Ctrl Pts',(-17.7119066821582,17.8315319119423,6.37443287054956));
#40374=CARTESIAN_POINT('Ctrl Pts',(-17.7160814181658,17.4033655966885,6.28989776862753));
#40375=CARTESIAN_POINT('Ctrl Pts',(-17.7047330456674,17.8055415663399,6.81009073748399));
#40376=CARTESIAN_POINT('Ctrl Pts',(-17.7057888706203,17.8314568157848,6.37441804392472));
#40377=CARTESIAN_POINT('Ctrl Pts',(-17.7136028587132,17.4033322762928,6.28989119000853));
#40378=CARTESIAN_POINT('Ctrl Pts',(-17.6914916361947,17.8051984797874,6.81005506963536));
#40379=CARTESIAN_POINT('Ctrl Pts',(-17.6935317272033,17.8311684204133,6.37436110452697));
#40380=CARTESIAN_POINT('Ctrl Pts',(-17.7086373302776,17.4032043210795,6.28986592714545));
#40381=CARTESIAN_POINT('Ctrl Pts',(-17.6848569462331,17.8049443436771,6.81002864903746));
#40382=CARTESIAN_POINT('Ctrl Pts',(-17.6873896796574,17.8309547927005,6.37431892689686));
#40383=CARTESIAN_POINT('Ctrl Pts',(-17.7061493215936,17.4031095435898,6.28984721473285));
#40384=CARTESIAN_POINT('Ctrl Pts',(-17.6650316986901,17.8039394480878,6.80992416632294));
#40385=CARTESIAN_POINT('Ctrl Pts',(-17.669033565516,17.8301099792034,6.37415213097543));
#40386=CARTESIAN_POINT('Ctrl Pts',(-17.6987148534351,17.402734784112,6.28977322402055));
#40387=CARTESIAN_POINT('Ctrl Pts',(-17.65188297285,17.8029458235526,6.80982084423287));
#40388=CARTESIAN_POINT('Ctrl Pts',(-17.6568553794863,17.8292744610696,6.37398717028588));
#40389=CARTESIAN_POINT('Ctrl Pts',(-17.6937840817574,17.4023642144883,6.28970006053293));
#40390=CARTESIAN_POINT('Ctrl Pts',(-17.6126371335032,17.7990126660086,6.80941167670247));
#40391=CARTESIAN_POINT('Ctrl Pts',(-17.6204837103719,17.825965596934,6.37333388403476));
#40392=CARTESIAN_POINT('Ctrl Pts',(-17.6790668911251,17.4008973914905,6.28941045804156));
#40393=CARTESIAN_POINT('Ctrl Pts',(-17.5867398984557,17.7951231176127,6.80900689352775));
#40394=CARTESIAN_POINT('Ctrl Pts',(-17.596453210412,17.8226910680451,6.37268737676991));
#40395=CARTESIAN_POINT('Ctrl Pts',(-17.6693554286528,17.3994468177432,6.28912406372419));
#40396=CARTESIAN_POINT('Ctrl Pts',(-17.5354697949089,17.7848516081068,6.80793609188225));
#40397=CARTESIAN_POINT('Ctrl Pts',(-17.5487818608033,17.8140306147149,6.37097749843788));
#40398=CARTESIAN_POINT('Ctrl Pts',(-17.6501291396514,17.3956161693061,6.28836775888534));
#40399=CARTESIAN_POINT('Ctrl Pts',(-17.5100969352081,17.7784696191355,6.80727007507948));
#40400=CARTESIAN_POINT('Ctrl Pts',(-17.5251318472474,17.8086411999732,6.36991343826254));
#40401=CARTESIAN_POINT('Ctrl Pts',(-17.6406143159052,17.3932360814621,6.28789784576675));
#40402=CARTESIAN_POINT('Ctrl Pts',(-17.4724356982661,17.7670045961486,6.80607073498154));
#40403=CARTESIAN_POINT('Ctrl Pts',(-17.4899271035391,17.7989402787506,6.36799813494449));
#40404=CARTESIAN_POINT('Ctrl Pts',(-17.6264913542181,17.3889603296644,6.28705366185705));
#40405=CARTESIAN_POINT('Ctrl Pts',(-17.4599484159706,17.7628670210704,6.80563750504227));
#40406=CARTESIAN_POINT('Ctrl Pts',(-17.4782302202683,17.7954342534171,6.36730592213287));
#40407=CARTESIAN_POINT('Ctrl Pts',(-17.6218086213275,17.3874172771144,6.28674900896883));
#40408=CARTESIAN_POINT('Ctrl Pts',(-17.4351090516651,17.7539492007634,6.8047025599668));
#40409=CARTESIAN_POINT('Ctrl Pts',(-17.454917776984,17.7878675018479,6.36581197902636));
#40410=CARTESIAN_POINT('Ctrl Pts',(-17.6124938623285,17.384091480323,6.28609237961543));
#40411=CARTESIAN_POINT('Ctrl Pts',(-17.4227335316578,17.7491576061505,6.804199652638));
#40412=CARTESIAN_POINT('Ctrl Pts',(-17.4432789672747,17.7837963825994,6.36500819678485));
#40413=CARTESIAN_POINT('Ctrl Pts',(-17.6078530426073,17.38230451645,6.28573957004644));
#40414=CARTESIAN_POINT('Ctrl Pts',(-17.3618547466598,17.7238403969658,6.8015386718093));
#40415=CARTESIAN_POINT('Ctrl Pts',(-17.3858250678238,17.7622268875734,6.36074961922872));
#40416=CARTESIAN_POINT('Ctrl Pts',(-17.5850234902864,17.3728628177143,6.28387544637182));
#40417=CARTESIAN_POINT('Ctrl Pts',(-17.3158627238175,17.6991343295047,6.79893094285691));
#40418=CARTESIAN_POINT('Ctrl Pts',(-17.3420267744581,17.7410737731548,6.35657324986094));
#40419=CARTESIAN_POINT('Ctrl Pts',(-17.5677764852266,17.3636490384775,6.28205632202897));
#40420=CARTESIAN_POINT('Ctrl Pts',(-17.2508193911024,17.6555966201116,6.7942958684358));
#40421=CARTESIAN_POINT('Ctrl Pts',(-17.2793471455071,17.7035182827478,6.34915847411566));
#40422=CARTESIAN_POINT('Ctrl Pts',(-17.5433852397352,17.3474123674201,6.27885063163761));
#40423=CARTESIAN_POINT('Ctrl Pts',(-17.2298005184759,17.6399964301089,6.79262936990691));
#40424=CARTESIAN_POINT('Ctrl Pts',(-17.2589173832124,17.6899870750125,6.34648693741537));
#40425=CARTESIAN_POINT('Ctrl Pts',(-17.5355031559793,17.3415945569023,6.27770199105668));
#40426=CARTESIAN_POINT('Ctrl Pts',(-17.204378613571,17.619097401045,6.79038682430432));
#40427=CARTESIAN_POINT('Ctrl Pts',(-17.2340263963876,17.6717874399427,6.34289368883238));
#40428=CARTESIAN_POINT('Ctrl Pts',(-17.5259699480092,17.3338006396197,6.27616319744218));
#40429=CARTESIAN_POINT('Ctrl Pts',(-17.1993309492766,17.6148421450605,6.78992974985876));
#40430=CARTESIAN_POINT('Ctrl Pts',(-17.2290682897225,17.6680734413416,6.34216041477718));
#40431=CARTESIAN_POINT('Ctrl Pts',(-17.5240770741103,17.3322137206402,6.27584988377669));
#40432=CARTESIAN_POINT('Ctrl Pts',(-17.1893716918988,17.6062334486389,6.78900404892269));
#40433=CARTESIAN_POINT('Ctrl Pts',(-17.2192636543449,17.6605500551435,6.34067503352136));
#40434=CARTESIAN_POINT('Ctrl Pts',(-17.5203423496229,17.3290032721058,6.27521602822943));
#40435=CARTESIAN_POINT('Ctrl Pts',(-17.1844557566987,17.6018767026284,6.78853506940883));
#40436=CARTESIAN_POINT('Ctrl Pts',(-17.2144128912708,17.6567376554324,6.33992233162338));
#40437=CARTESIAN_POINT('Ctrl Pts',(-17.5184988766973,17.3273785031339,6.27489524164313));
#40438=CARTESIAN_POINT('Ctrl Pts',(-17.169896855944,17.5886510409319,6.78710983089398));
#40439=CARTESIAN_POINT('Ctrl Pts',(-17.2000081285538,17.6451450983018,6.33763355279219));
#40440=CARTESIAN_POINT('Ctrl Pts',(-17.5130392850471,17.3224462500153,6.27392144126411));
#40441=CARTESIAN_POINT('Ctrl Pts',(-17.1604426857215,17.5796268087842,6.78613528430944));
#40442=CARTESIAN_POINT('Ctrl Pts',(-17.1906117770433,17.6372170607117,6.33606827910802));
#40443=CARTESIAN_POINT('Ctrl Pts',(-17.5094939755331,17.3190808343234,6.27325698974518));
#40444=CARTESIAN_POINT('Ctrl Pts',(-17.1144092624932,17.5334875838914,6.78114111890133));
#40445=CARTESIAN_POINT('Ctrl Pts',(-17.1445255959529,17.5964801911601,6.32802538713625));
#40446=CARTESIAN_POINT('Ctrl Pts',(-17.4922314331161,17.3018741366695,6.26985978195909));
#40447=CARTESIAN_POINT('Ctrl Pts',(-17.0815070486393,17.4933474524288,6.77676052830464));
#40448=CARTESIAN_POINT('Ctrl Pts',(-17.1109009441881,17.5607248183131,6.32096601796079));
#40449=CARTESIAN_POINT('Ctrl Pts',(-17.4798931004167,17.2869047271829,6.26690429360894));
#40450=CARTESIAN_POINT('Ctrl Pts',(-17.0453050933139,17.4391198002594,6.77077798629523));
#40451=CARTESIAN_POINT('Ctrl Pts',(-17.0729618602987,17.5119192000139,6.31133007096938));
#40452=CARTESIAN_POINT('Ctrl Pts',(-17.4663173790063,17.2666817095338,6.26291155808251));
#40453=CARTESIAN_POINT('Ctrl Pts',(-17.0383132060228,17.4280698300166,6.76955593094628));
#40454=CARTESIAN_POINT('Ctrl Pts',(-17.065556626733,17.5019159878677,6.30935508478244));
#40455=CARTESIAN_POINT('Ctrl Pts',(-17.4636954152817,17.2625608716606,6.2620979596344));
#40456=CARTESIAN_POINT('Ctrl Pts',(-17.0248360913008,17.4055530530904,6.76705920363801));
#40457=CARTESIAN_POINT('Ctrl Pts',(-17.0511605700457,17.4814635711966,6.30531705781432));
#40458=CARTESIAN_POINT('Ctrl Pts',(-17.4586415045071,17.2541637364834,6.26044006957447));
#40459=CARTESIAN_POINT('Ctrl Pts',(-17.018385745669,17.3941425328792,6.76579076471037));
#40460=CARTESIAN_POINT('Ctrl Pts',(-17.044207273457,17.4710642956499,6.30326387477087));
#40461=CARTESIAN_POINT('Ctrl Pts',(-17.4562226243632,17.2499084384684,6.25959992396146));
#40462=CARTESIAN_POINT('Ctrl Pts',(-16.9999748915757,17.3596229038005,6.76194338591157));
#40463=CARTESIAN_POINT('Ctrl Pts',(-17.0241507155953,17.4394666729185,6.29702539181943));
#40464=CARTESIAN_POINT('Ctrl Pts',(-17.449318544805,17.237035119937,6.25705827774745));
#40465=CARTESIAN_POINT('Ctrl Pts',(-16.9889119861745,17.3361594967524,6.75931504519851));
#40466=CARTESIAN_POINT('Ctrl Pts',(-17.0118468913603,17.4178612762011,6.29275972600569));
#40467=CARTESIAN_POINT('Ctrl Pts',(-17.4451699630122,17.2282849645212,6.25533068906623));
#40468=CARTESIAN_POINT('Ctrl Pts',(-16.969151536231,17.2883531218114,6.75393133468145));
#40469=CARTESIAN_POINT('Ctrl Pts',(-16.9893185039968,17.3735255531602,6.28400629367688));
#40470=CARTESIAN_POINT('Ctrl Pts',(-17.4377597911824,17.2104566385494,6.25181074996914));
#40471=CARTESIAN_POINT('Ctrl Pts',(-16.9604540998271,17.2640101175317,6.75117596780138));
#40472=CARTESIAN_POINT('Ctrl Pts',(-16.979100694343,17.3507885344851,6.27951720585606));
#40473=CARTESIAN_POINT('Ctrl Pts',(-17.4344982506951,17.2013784496697,6.25001839593549));
#40474=CARTESIAN_POINT('Ctrl Pts',(-16.9454368141968,17.2144400485736,6.74553518479638));
#40475=CARTESIAN_POINT('Ctrl Pts',(-16.9607944578447,17.3041453864073,6.27030820660447));
#40476=CARTESIAN_POINT('Ctrl Pts',(-17.4288667753564,17.1828923505283,6.24636858926135));
#40477=CARTESIAN_POINT('Ctrl Pts',(-16.9391152612491,17.1892056047591,6.74264892813991));
#40478=CARTESIAN_POINT('Ctrl Pts',(-16.9527111071462,17.2802251876746,6.26558551739275));
#40479=CARTESIAN_POINT('Ctrl Pts',(-17.4264961901478,17.173481691707,6.24451059395842));
#40480=CARTESIAN_POINT('Ctrl Pts',(-16.9340264307573,17.163528852123,6.73969634090002));
#40481=CARTESIAN_POINT('Ctrl Pts',(-16.9457712867961,17.2557485214382,6.26075296190838));
#40482=CARTESIAN_POINT('Ctrl Pts',(-17.4245878781802,17.16390605946,6.24262002709426));
#40483=CARTESIAN_POINT('Origin',(-37.718924746634,17.5,-2.5));
#40484=CARTESIAN_POINT('Ctrl Pts',(-36.918924746634,26.,0.));
#40485=CARTESIAN_POINT('Ctrl Pts',(-36.7522580799673,26.,5.19615242270663));
#40486=CARTESIAN_POINT('Ctrl Pts',(-36.5855914133007,30.5,7.79422863405995));
#40487=CARTESIAN_POINT('Ctrl Pts',(-36.418924746634,35.,10.3923048454133));
#40488=CARTESIAN_POINT('Ctrl Pts',(-36.2522580799673,39.5,7.79422863405995));
#40489=CARTESIAN_POINT('Ctrl Pts',(-36.0855914133007,44.,5.19615242270663));
#40490=CARTESIAN_POINT('Ctrl Pts',(-35.918924746634,44.,1.10218211923262E-15));
#40491=CARTESIAN_POINT('Ctrl Pts',(-35.7522580799673,44.,-5.19615242270663));
#40492=CARTESIAN_POINT('Ctrl Pts',(-35.5855914133007,39.5,-7.79422863405995));
#40493=CARTESIAN_POINT('Ctrl Pts',(-35.418924746634,35.,-10.3923048454133));
#40494=CARTESIAN_POINT('Ctrl Pts',(-35.2522580799673,30.5,-7.79422863405995));
#40495=CARTESIAN_POINT('Ctrl Pts',(-35.0855914133007,26.,-5.19615242270663));
#40496=CARTESIAN_POINT('Ctrl Pts',(-34.918924746634,26.,0.));
#40497=CARTESIAN_POINT('Ctrl Pts',(-34.7522580799673,26.,5.19615242270663));
#40498=CARTESIAN_POINT('Ctrl Pts',(-34.5855914133007,30.5,7.79422863405995));
#40499=CARTESIAN_POINT('Ctrl Pts',(-34.418924746634,35.,10.3923048454133));
#40500=CARTESIAN_POINT('Ctrl Pts',(-34.2522580799673,39.5,7.79422863405995));
#40501=CARTESIAN_POINT('Ctrl Pts',(-34.0855914133007,44.,5.19615242270663));
#40502=CARTESIAN_POINT('Ctrl Pts',(-33.918924746634,44.,1.10218211923262E-15));
#40503=CARTESIAN_POINT('Ctrl Pts',(-33.7522580799673,44.,-5.19615242270663));
#40504=CARTESIAN_POINT('Ctrl Pts',(-33.5855914133007,39.5,-7.79422863405995));
#40505=CARTESIAN_POINT('Ctrl Pts',(-33.418924746634,35.,-10.3923048454133));
#40506=CARTESIAN_POINT('Ctrl Pts',(-33.2522580799673,30.5,-7.79422863405995));
#40507=CARTESIAN_POINT('Ctrl Pts',(-33.0855914133007,26.,-5.19615242270663));
#40508=CARTESIAN_POINT('Ctrl Pts',(-32.918924746634,26.,0.));
#40509=CARTESIAN_POINT('Ctrl Pts',(-32.7522580799673,26.,5.19615242270663));
#40510=CARTESIAN_POINT('Ctrl Pts',(-32.5855914133007,30.5,7.79422863405995));
#40511=CARTESIAN_POINT('Ctrl Pts',(-32.418924746634,35.,10.3923048454133));
#40512=CARTESIAN_POINT('Ctrl Pts',(-32.2522580799673,39.5,7.79422863405995));
#40513=CARTESIAN_POINT('Ctrl Pts',(-32.0855914133007,44.,5.19615242270663));
#40514=CARTESIAN_POINT('Ctrl Pts',(-31.918924746634,44.,1.10218211923262E-15));
#40515=CARTESIAN_POINT('Ctrl Pts',(-31.7522580799673,44.,-5.19615242270663));
#40516=CARTESIAN_POINT('Ctrl Pts',(-31.5855914133007,39.5,-7.79422863405995));
#40517=CARTESIAN_POINT('Ctrl Pts',(-31.418924746634,35.,-10.3923048454133));
#40518=CARTESIAN_POINT('Ctrl Pts',(-31.2522580799673,30.5,-7.79422863405995));
#40519=CARTESIAN_POINT('Ctrl Pts',(-31.0855914133007,26.,-5.19615242270663));
#40520=CARTESIAN_POINT('Ctrl Pts',(-30.918924746634,26.,0.));
#40521=CARTESIAN_POINT('Ctrl Pts',(-30.7522580799673,26.,5.19615242270663));
#40522=CARTESIAN_POINT('Ctrl Pts',(-30.5855914133007,30.5,7.79422863405995));
#40523=CARTESIAN_POINT('Ctrl Pts',(-30.418924746634,35.,10.3923048454133));
#40524=CARTESIAN_POINT('Ctrl Pts',(-30.2522580799673,39.5,7.79422863405995));
#40525=CARTESIAN_POINT('Ctrl Pts',(-30.0855914133007,44.,5.19615242270663));
#40526=CARTESIAN_POINT('Ctrl Pts',(-29.918924746634,44.,1.10218211923262E-15));
#40527=CARTESIAN_POINT('Ctrl Pts',(-29.7522580799673,44.,-5.19615242270663));
#40528=CARTESIAN_POINT('Ctrl Pts',(-29.5855914133007,39.5,-7.79422863405995));
#40529=CARTESIAN_POINT('Ctrl Pts',(-29.418924746634,35.,-10.3923048454133));
#40530=CARTESIAN_POINT('Ctrl Pts',(-29.2522580799673,30.5,-7.79422863405995));
#40531=CARTESIAN_POINT('Ctrl Pts',(-29.0855914133007,26.,-5.19615242270663));
#40532=CARTESIAN_POINT('Ctrl Pts',(-28.918924746634,26.,0.));
#40533=CARTESIAN_POINT('Ctrl Pts',(-28.7522580799673,26.,5.19615242270663));
#40534=CARTESIAN_POINT('Ctrl Pts',(-28.5855914133007,30.5,7.79422863405995));
#40535=CARTESIAN_POINT('Ctrl Pts',(-28.418924746634,35.,10.3923048454133));
#40536=CARTESIAN_POINT('Ctrl Pts',(-28.2522580799673,39.5,7.79422863405995));
#40537=CARTESIAN_POINT('Ctrl Pts',(-28.0855914133007,44.,5.19615242270663));
#40538=CARTESIAN_POINT('Ctrl Pts',(-27.918924746634,44.,1.10218211923262E-15));
#40539=CARTESIAN_POINT('Ctrl Pts',(-27.7522580799673,44.,-5.19615242270663));
#40540=CARTESIAN_POINT('Ctrl Pts',(-27.5855914133007,39.5,-7.79422863405995));
#40541=CARTESIAN_POINT('Ctrl Pts',(-27.418924746634,35.,-10.3923048454133));
#40542=CARTESIAN_POINT('Ctrl Pts',(-27.2522580799673,30.5,-7.79422863405995));
#40543=CARTESIAN_POINT('Ctrl Pts',(-27.0855914133007,26.,-5.19615242270663));
#40544=CARTESIAN_POINT('Ctrl Pts',(-26.918924746634,26.,0.));
#40545=CARTESIAN_POINT('Ctrl Pts',(-26.7522580799673,26.,5.19615242270663));
#40546=CARTESIAN_POINT('Ctrl Pts',(-26.5855914133007,30.5,7.79422863405995));
#40547=CARTESIAN_POINT('Ctrl Pts',(-26.418924746634,35.,10.3923048454133));
#40548=CARTESIAN_POINT('Ctrl Pts',(-26.2522580799673,39.5,7.79422863405995));
#40549=CARTESIAN_POINT('Ctrl Pts',(-26.0855914133007,44.,5.19615242270663));
#40550=CARTESIAN_POINT('Ctrl Pts',(-25.918924746634,44.,1.10218211923262E-15));
#40551=CARTESIAN_POINT('Ctrl Pts',(-25.7522580799673,44.,-5.19615242270663));
#40552=CARTESIAN_POINT('Ctrl Pts',(-25.5855914133007,39.5,-7.79422863405995));
#40553=CARTESIAN_POINT('Ctrl Pts',(-25.418924746634,35.,-10.3923048454133));
#40554=CARTESIAN_POINT('Ctrl Pts',(-25.2522580799673,30.5,-7.79422863405995));
#40555=CARTESIAN_POINT('Ctrl Pts',(-25.0855914133007,26.,-5.19615242270663));
#40556=CARTESIAN_POINT('Ctrl Pts',(-24.918924746634,26.,0.));
#40557=CARTESIAN_POINT('Ctrl Pts',(-24.7522580799673,26.,5.19615242270663));
#40558=CARTESIAN_POINT('Ctrl Pts',(-24.5855914133007,30.5,7.79422863405995));
#40559=CARTESIAN_POINT('Ctrl Pts',(-24.418924746634,35.,10.3923048454133));
#40560=CARTESIAN_POINT('Ctrl Pts',(-24.2522580799673,39.5,7.79422863405995));
#40561=CARTESIAN_POINT('Ctrl Pts',(-24.0855914133007,44.,5.19615242270663));
#40562=CARTESIAN_POINT('Ctrl Pts',(-23.918924746634,44.,1.10218211923262E-15));
#40563=CARTESIAN_POINT('Ctrl Pts',(-23.7522580799673,44.,-5.19615242270663));
#40564=CARTESIAN_POINT('Ctrl Pts',(-23.5855914133007,39.5,-7.79422863405995));
#40565=CARTESIAN_POINT('Ctrl Pts',(-23.418924746634,35.,-10.3923048454133));
#40566=CARTESIAN_POINT('Ctrl Pts',(-23.2522580799673,30.5,-7.79422863405995));
#40567=CARTESIAN_POINT('Ctrl Pts',(-23.0855914133007,26.,-5.19615242270663));
#40568=CARTESIAN_POINT('Ctrl Pts',(-22.918924746634,26.,0.));
#40569=CARTESIAN_POINT('Ctrl Pts',(-22.7522580799673,26.,5.19615242270663));
#40570=CARTESIAN_POINT('Ctrl Pts',(-22.5855914133007,30.5,7.79422863405995));
#40571=CARTESIAN_POINT('Ctrl Pts',(-22.418924746634,35.,10.3923048454133));
#40572=CARTESIAN_POINT('Ctrl Pts',(-22.2522580799674,39.5,7.79422863405995));
#40573=CARTESIAN_POINT('Ctrl Pts',(-22.0855914133007,44.,5.19615242270663));
#40574=CARTESIAN_POINT('Ctrl Pts',(-21.918924746634,44.,1.10218211923262E-15));
#40575=CARTESIAN_POINT('Ctrl Pts',(-21.7522580799673,44.,-5.19615242270663));
#40576=CARTESIAN_POINT('Ctrl Pts',(-21.5855914133006,39.5,-7.79422863405995));
#40577=CARTESIAN_POINT('Ctrl Pts',(-21.418924746634,35.,-10.3923048454133));
#40578=CARTESIAN_POINT('Ctrl Pts',(-21.2522580799673,30.5,-7.79422863405995));
#40579=CARTESIAN_POINT('Ctrl Pts',(-21.0855914133007,26.,-5.19615242270663));
#40580=CARTESIAN_POINT('Ctrl Pts',(-20.918924746634,26.,0.));
#40581=CARTESIAN_POINT('Ctrl Pts',(-20.7522580799673,26.,5.19615242270663));
#40582=CARTESIAN_POINT('Ctrl Pts',(-20.5855914133006,30.5,7.79422863405995));
#40583=CARTESIAN_POINT('Ctrl Pts',(-20.418924746634,35.,10.3923048454133));
#40584=CARTESIAN_POINT('Ctrl Pts',(-20.2522580799673,39.5,7.79422863405995));
#40585=CARTESIAN_POINT('Ctrl Pts',(-20.0855914133007,44.,5.19615242270663));
#40586=CARTESIAN_POINT('Ctrl Pts',(-19.918924746634,44.,1.10218211923262E-15));
#40587=CARTESIAN_POINT('Ctrl Pts',(-19.7522580799674,44.,-5.19615242270663));
#40588=CARTESIAN_POINT('Ctrl Pts',(-19.5855914133006,39.5,-7.79422863405995));
#40589=CARTESIAN_POINT('Ctrl Pts',(-19.418924746634,35.,-10.3923048454133));
#40590=CARTESIAN_POINT('Ctrl Pts',(-19.2522580799674,30.5,-7.79422863405995));
#40591=CARTESIAN_POINT('Ctrl Pts',(-19.0855914133007,26.,-5.19615242270663));
#40592=CARTESIAN_POINT('Ctrl Pts',(-18.918924746634,26.,0.));
#40593=CARTESIAN_POINT('Ctrl Pts',(-18.7522580799673,26.,5.19615242270663));
#40594=CARTESIAN_POINT('Ctrl Pts',(-18.5855914133006,30.5,7.79422863405995));
#40595=CARTESIAN_POINT('Ctrl Pts',(-18.418924746634,35.,10.3923048454133));
#40596=CARTESIAN_POINT('Ctrl Pts',(-18.2522580799673,39.5,7.79422863405995));
#40597=CARTESIAN_POINT('Ctrl Pts',(-18.0855914133006,44.,5.19615242270663));
#40598=CARTESIAN_POINT('Ctrl Pts',(-17.918924746634,44.,1.10218211923262E-15));
#40599=CARTESIAN_POINT('Ctrl Pts',(-17.7522580799673,44.,-5.19615242270663));
#40600=CARTESIAN_POINT('Ctrl Pts',(-17.5855914133006,39.5,-7.79422863405995));
#40601=CARTESIAN_POINT('Ctrl Pts',(-17.418924746634,35.,-10.3923048454133));
#40602=CARTESIAN_POINT('Ctrl Pts',(-17.2522580799673,30.5,-7.79422863405995));
#40603=CARTESIAN_POINT('Ctrl Pts',(-17.0855914133007,26.,-5.19615242270663));
#40604=CARTESIAN_POINT('Ctrl Pts',(-16.918924746634,26.,0.));
#40605=CARTESIAN_POINT('Ctrl Pts',(-36.918924746634,24.4,0.));
#40606=CARTESIAN_POINT('Ctrl Pts',(-36.7522580799673,24.4,6.11991285341003));
#40607=CARTESIAN_POINT('Ctrl Pts',(-36.5855914133007,29.7,9.17986928011504));
#40608=CARTESIAN_POINT('Ctrl Pts',(-36.418924746634,35.,12.2398257068201));
#40609=CARTESIAN_POINT('Ctrl Pts',(-36.2522580799673,40.3,9.17986928011504));
#40610=CARTESIAN_POINT('Ctrl Pts',(-36.0855914133007,45.6,6.11991285341004));
#40611=CARTESIAN_POINT('Ctrl Pts',(-35.918924746634,45.6,1.29812560709619E-15));
#40612=CARTESIAN_POINT('Ctrl Pts',(-35.7522580799673,45.6,-6.11991285341003));
#40613=CARTESIAN_POINT('Ctrl Pts',(-35.5855914133007,40.3,-9.17986928011504));
#40614=CARTESIAN_POINT('Ctrl Pts',(-35.418924746634,35.,-12.2398257068201));
#40615=CARTESIAN_POINT('Ctrl Pts',(-35.2522580799673,29.7,-9.17986928011506));
#40616=CARTESIAN_POINT('Ctrl Pts',(-35.0855914133007,24.4,-6.11991285341004));
#40617=CARTESIAN_POINT('Ctrl Pts',(-34.918924746634,24.4,0.));
#40618=CARTESIAN_POINT('Ctrl Pts',(-34.7522580799673,24.4,6.11991285341003));
#40619=CARTESIAN_POINT('Ctrl Pts',(-34.5855914133007,29.7,9.17986928011504));
#40620=CARTESIAN_POINT('Ctrl Pts',(-34.418924746634,35.,12.2398257068201));
#40621=CARTESIAN_POINT('Ctrl Pts',(-34.2522580799673,40.3,9.17986928011504));
#40622=CARTESIAN_POINT('Ctrl Pts',(-34.0855914133007,45.6,6.11991285341004));
#40623=CARTESIAN_POINT('Ctrl Pts',(-33.918924746634,45.6,1.29812560709619E-15));
#40624=CARTESIAN_POINT('Ctrl Pts',(-33.7522580799673,45.6,-6.11991285341003));
#40625=CARTESIAN_POINT('Ctrl Pts',(-33.5855914133007,40.3,-9.17986928011504));
#40626=CARTESIAN_POINT('Ctrl Pts',(-33.418924746634,35.,-12.2398257068201));
#40627=CARTESIAN_POINT('Ctrl Pts',(-33.2522580799673,29.7,-9.17986928011506));
#40628=CARTESIAN_POINT('Ctrl Pts',(-33.0855914133007,24.4,-6.11991285341004));
#40629=CARTESIAN_POINT('Ctrl Pts',(-32.918924746634,24.4,0.));
#40630=CARTESIAN_POINT('Ctrl Pts',(-32.7522580799673,24.4,6.11991285341003));
#40631=CARTESIAN_POINT('Ctrl Pts',(-32.5855914133007,29.7,9.17986928011504));
#40632=CARTESIAN_POINT('Ctrl Pts',(-32.418924746634,35.,12.2398257068201));
#40633=CARTESIAN_POINT('Ctrl Pts',(-32.2522580799673,40.3,9.17986928011504));
#40634=CARTESIAN_POINT('Ctrl Pts',(-32.0855914133007,45.6,6.11991285341004));
#40635=CARTESIAN_POINT('Ctrl Pts',(-31.918924746634,45.6,1.29812560709619E-15));
#40636=CARTESIAN_POINT('Ctrl Pts',(-31.7522580799673,45.6,-6.11991285341003));
#40637=CARTESIAN_POINT('Ctrl Pts',(-31.5855914133007,40.3,-9.17986928011504));
#40638=CARTESIAN_POINT('Ctrl Pts',(-31.418924746634,35.,-12.2398257068201));
#40639=CARTESIAN_POINT('Ctrl Pts',(-31.2522580799673,29.7,-9.17986928011506));
#40640=CARTESIAN_POINT('Ctrl Pts',(-31.0855914133007,24.4,-6.11991285341004));
#40641=CARTESIAN_POINT('Ctrl Pts',(-30.918924746634,24.4,0.));
#40642=CARTESIAN_POINT('Ctrl Pts',(-30.7522580799673,24.4,6.11991285341003));
#40643=CARTESIAN_POINT('Ctrl Pts',(-30.5855914133007,29.7,9.17986928011504));
#40644=CARTESIAN_POINT('Ctrl Pts',(-30.418924746634,35.,12.2398257068201));
#40645=CARTESIAN_POINT('Ctrl Pts',(-30.2522580799673,40.3,9.17986928011504));
#40646=CARTESIAN_POINT('Ctrl Pts',(-30.0855914133007,45.6,6.11991285341004));
#40647=CARTESIAN_POINT('Ctrl Pts',(-29.918924746634,45.6,1.29812560709619E-15));
#40648=CARTESIAN_POINT('Ctrl Pts',(-29.7522580799673,45.6,-6.11991285341003));
#40649=CARTESIAN_POINT('Ctrl Pts',(-29.5855914133007,40.3,-9.17986928011504));
#40650=CARTESIAN_POINT('Ctrl Pts',(-29.418924746634,35.,-12.2398257068201));
#40651=CARTESIAN_POINT('Ctrl Pts',(-29.2522580799673,29.7,-9.17986928011506));
#40652=CARTESIAN_POINT('Ctrl Pts',(-29.0855914133007,24.4,-6.11991285341004));
#40653=CARTESIAN_POINT('Ctrl Pts',(-28.918924746634,24.4,0.));
#40654=CARTESIAN_POINT('Ctrl Pts',(-28.7522580799673,24.4,6.11991285341003));
#40655=CARTESIAN_POINT('Ctrl Pts',(-28.5855914133007,29.7,9.17986928011504));
#40656=CARTESIAN_POINT('Ctrl Pts',(-28.418924746634,35.,12.2398257068201));
#40657=CARTESIAN_POINT('Ctrl Pts',(-28.2522580799673,40.3,9.17986928011504));
#40658=CARTESIAN_POINT('Ctrl Pts',(-28.0855914133007,45.6,6.11991285341004));
#40659=CARTESIAN_POINT('Ctrl Pts',(-27.918924746634,45.6,1.29812560709619E-15));
#40660=CARTESIAN_POINT('Ctrl Pts',(-27.7522580799673,45.6,-6.11991285341003));
#40661=CARTESIAN_POINT('Ctrl Pts',(-27.5855914133007,40.3,-9.17986928011504));
#40662=CARTESIAN_POINT('Ctrl Pts',(-27.418924746634,35.,-12.2398257068201));
#40663=CARTESIAN_POINT('Ctrl Pts',(-27.2522580799673,29.7,-9.17986928011506));
#40664=CARTESIAN_POINT('Ctrl Pts',(-27.0855914133007,24.4,-6.11991285341004));
#40665=CARTESIAN_POINT('Ctrl Pts',(-26.918924746634,24.4,0.));
#40666=CARTESIAN_POINT('Ctrl Pts',(-26.7522580799673,24.4,6.11991285341003));
#40667=CARTESIAN_POINT('Ctrl Pts',(-26.5855914133007,29.7,9.17986928011504));
#40668=CARTESIAN_POINT('Ctrl Pts',(-26.418924746634,35.,12.2398257068201));
#40669=CARTESIAN_POINT('Ctrl Pts',(-26.2522580799673,40.3,9.17986928011504));
#40670=CARTESIAN_POINT('Ctrl Pts',(-26.0855914133007,45.6,6.11991285341004));
#40671=CARTESIAN_POINT('Ctrl Pts',(-25.918924746634,45.6,1.29812560709619E-15));
#40672=CARTESIAN_POINT('Ctrl Pts',(-25.7522580799673,45.6,-6.11991285341003));
#40673=CARTESIAN_POINT('Ctrl Pts',(-25.5855914133007,40.3,-9.17986928011504));
#40674=CARTESIAN_POINT('Ctrl Pts',(-25.418924746634,35.,-12.2398257068201));
#40675=CARTESIAN_POINT('Ctrl Pts',(-25.2522580799673,29.7,-9.17986928011506));
#40676=CARTESIAN_POINT('Ctrl Pts',(-25.0855914133007,24.4,-6.11991285341004));
#40677=CARTESIAN_POINT('Ctrl Pts',(-24.918924746634,24.4,0.));
#40678=CARTESIAN_POINT('Ctrl Pts',(-24.7522580799673,24.4,6.11991285341003));
#40679=CARTESIAN_POINT('Ctrl Pts',(-24.5855914133007,29.7,9.17986928011504));
#40680=CARTESIAN_POINT('Ctrl Pts',(-24.418924746634,35.,12.2398257068201));
#40681=CARTESIAN_POINT('Ctrl Pts',(-24.2522580799673,40.3,9.17986928011504));
#40682=CARTESIAN_POINT('Ctrl Pts',(-24.0855914133007,45.6,6.11991285341004));
#40683=CARTESIAN_POINT('Ctrl Pts',(-23.918924746634,45.6,1.29812560709619E-15));
#40684=CARTESIAN_POINT('Ctrl Pts',(-23.7522580799673,45.6,-6.11991285341003));
#40685=CARTESIAN_POINT('Ctrl Pts',(-23.5855914133007,40.3,-9.17986928011504));
#40686=CARTESIAN_POINT('Ctrl Pts',(-23.418924746634,35.,-12.2398257068201));
#40687=CARTESIAN_POINT('Ctrl Pts',(-23.2522580799673,29.7,-9.17986928011506));
#40688=CARTESIAN_POINT('Ctrl Pts',(-23.0855914133007,24.4,-6.11991285341004));
#40689=CARTESIAN_POINT('Ctrl Pts',(-22.918924746634,24.4,0.));
#40690=CARTESIAN_POINT('Ctrl Pts',(-22.7522580799673,24.4,6.11991285341003));
#40691=CARTESIAN_POINT('Ctrl Pts',(-22.5855914133007,29.7,9.17986928011504));
#40692=CARTESIAN_POINT('Ctrl Pts',(-22.418924746634,35.,12.2398257068201));
#40693=CARTESIAN_POINT('Ctrl Pts',(-22.2522580799673,40.3,9.17986928011504));
#40694=CARTESIAN_POINT('Ctrl Pts',(-22.0855914133007,45.6,6.11991285341004));
#40695=CARTESIAN_POINT('Ctrl Pts',(-21.918924746634,45.6,1.29812560709619E-15));
#40696=CARTESIAN_POINT('Ctrl Pts',(-21.7522580799673,45.6,-6.11991285341003));
#40697=CARTESIAN_POINT('Ctrl Pts',(-21.5855914133007,40.3,-9.17986928011504));
#40698=CARTESIAN_POINT('Ctrl Pts',(-21.418924746634,35.,-12.2398257068201));
#40699=CARTESIAN_POINT('Ctrl Pts',(-21.2522580799673,29.7,-9.17986928011506));
#40700=CARTESIAN_POINT('Ctrl Pts',(-21.0855914133007,24.4,-6.11991285341004));
#40701=CARTESIAN_POINT('Ctrl Pts',(-20.918924746634,24.4,0.));
#40702=CARTESIAN_POINT('Ctrl Pts',(-20.7522580799673,24.4,6.11991285341003));
#40703=CARTESIAN_POINT('Ctrl Pts',(-20.5855914133007,29.7,9.17986928011504));
#40704=CARTESIAN_POINT('Ctrl Pts',(-20.418924746634,35.,12.2398257068201));
#40705=CARTESIAN_POINT('Ctrl Pts',(-20.2522580799673,40.3,9.17986928011504));
#40706=CARTESIAN_POINT('Ctrl Pts',(-20.0855914133007,45.6,6.11991285341004));
#40707=CARTESIAN_POINT('Ctrl Pts',(-19.918924746634,45.6,1.29812560709619E-15));
#40708=CARTESIAN_POINT('Ctrl Pts',(-19.7522580799673,45.6,-6.11991285341003));
#40709=CARTESIAN_POINT('Ctrl Pts',(-19.5855914133007,40.3,-9.17986928011504));
#40710=CARTESIAN_POINT('Ctrl Pts',(-19.418924746634,35.,-12.2398257068201));
#40711=CARTESIAN_POINT('Ctrl Pts',(-19.2522580799673,29.7,-9.17986928011506));
#40712=CARTESIAN_POINT('Ctrl Pts',(-19.0855914133006,24.4,-6.11991285341004));
#40713=CARTESIAN_POINT('Ctrl Pts',(-18.918924746634,24.4,0.));
#40714=CARTESIAN_POINT('Ctrl Pts',(-18.7522580799673,24.4,6.11991285341003));
#40715=CARTESIAN_POINT('Ctrl Pts',(-18.5855914133007,29.7,9.17986928011504));
#40716=CARTESIAN_POINT('Ctrl Pts',(-18.418924746634,35.,12.2398257068201));
#40717=CARTESIAN_POINT('Ctrl Pts',(-18.2522580799673,40.3,9.17986928011504));
#40718=CARTESIAN_POINT('Ctrl Pts',(-18.0855914133007,45.6,6.11991285341004));
#40719=CARTESIAN_POINT('Ctrl Pts',(-17.918924746634,45.6,1.29812560709619E-15));
#40720=CARTESIAN_POINT('Ctrl Pts',(-17.7522580799674,45.6,-6.11991285341003));
#40721=CARTESIAN_POINT('Ctrl Pts',(-17.5855914133007,40.3,-9.17986928011504));
#40722=CARTESIAN_POINT('Ctrl Pts',(-17.418924746634,35.,-12.2398257068201));
#40723=CARTESIAN_POINT('Ctrl Pts',(-17.2522580799674,29.7,-9.17986928011506));
#40724=CARTESIAN_POINT('Ctrl Pts',(-17.0855914133007,24.4,-6.11991285341004));
#40725=CARTESIAN_POINT('Ctrl Pts',(-16.918924746634,24.4,0.));
#40726=CARTESIAN_POINT('Ctrl Pts',(-38.518924746634,24.4,0.));
#40727=CARTESIAN_POINT('Ctrl Pts',(-38.3522580799673,24.4,6.11991285341003));
#40728=CARTESIAN_POINT('Ctrl Pts',(-38.1855914133007,29.7,9.17986928011504));
#40729=CARTESIAN_POINT('Ctrl Pts',(-38.018924746634,35.,12.2398257068201));
#40730=CARTESIAN_POINT('Ctrl Pts',(-37.8522580799673,40.3,9.17986928011504));
#40731=CARTESIAN_POINT('Ctrl Pts',(-37.6855914133007,45.6,6.11991285341004));
#40732=CARTESIAN_POINT('Ctrl Pts',(-37.518924746634,45.6,1.29812560709619E-15));
#40733=CARTESIAN_POINT('Ctrl Pts',(-37.3522580799673,45.6,-6.11991285341003));
#40734=CARTESIAN_POINT('Ctrl Pts',(-37.1855914133007,40.3,-9.17986928011504));
#40735=CARTESIAN_POINT('Ctrl Pts',(-37.018924746634,35.,-12.2398257068201));
#40736=CARTESIAN_POINT('Ctrl Pts',(-36.8522580799673,29.7,-9.17986928011506));
#40737=CARTESIAN_POINT('Ctrl Pts',(-36.6855914133007,24.4,-6.11991285341004));
#40738=CARTESIAN_POINT('Ctrl Pts',(-36.518924746634,24.4,0.));
#40739=CARTESIAN_POINT('Ctrl Pts',(-36.3522580799673,24.4,6.11991285341003));
#40740=CARTESIAN_POINT('Ctrl Pts',(-36.1855914133007,29.7,9.17986928011504));
#40741=CARTESIAN_POINT('Ctrl Pts',(-36.018924746634,35.,12.2398257068201));
#40742=CARTESIAN_POINT('Ctrl Pts',(-35.8522580799673,40.3,9.17986928011504));
#40743=CARTESIAN_POINT('Ctrl Pts',(-35.6855914133007,45.6,6.11991285341004));
#40744=CARTESIAN_POINT('Ctrl Pts',(-35.518924746634,45.6,1.29812560709619E-15));
#40745=CARTESIAN_POINT('Ctrl Pts',(-35.3522580799673,45.6,-6.11991285341003));
#40746=CARTESIAN_POINT('Ctrl Pts',(-35.1855914133007,40.3,-9.17986928011504));
#40747=CARTESIAN_POINT('Ctrl Pts',(-35.018924746634,35.,-12.2398257068201));
#40748=CARTESIAN_POINT('Ctrl Pts',(-34.8522580799673,29.7,-9.17986928011506));
#40749=CARTESIAN_POINT('Ctrl Pts',(-34.6855914133007,24.4,-6.11991285341004));
#40750=CARTESIAN_POINT('Ctrl Pts',(-34.518924746634,24.4,0.));
#40751=CARTESIAN_POINT('Ctrl Pts',(-34.3522580799673,24.4,6.11991285341003));
#40752=CARTESIAN_POINT('Ctrl Pts',(-34.1855914133007,29.7,9.17986928011504));
#40753=CARTESIAN_POINT('Ctrl Pts',(-34.018924746634,35.,12.2398257068201));
#40754=CARTESIAN_POINT('Ctrl Pts',(-33.8522580799673,40.3,9.17986928011504));
#40755=CARTESIAN_POINT('Ctrl Pts',(-33.6855914133007,45.6,6.11991285341004));
#40756=CARTESIAN_POINT('Ctrl Pts',(-33.518924746634,45.6,1.29812560709619E-15));
#40757=CARTESIAN_POINT('Ctrl Pts',(-33.3522580799673,45.6,-6.11991285341003));
#40758=CARTESIAN_POINT('Ctrl Pts',(-33.1855914133007,40.3,-9.17986928011504));
#40759=CARTESIAN_POINT('Ctrl Pts',(-33.018924746634,35.,-12.2398257068201));
#40760=CARTESIAN_POINT('Ctrl Pts',(-32.8522580799673,29.7,-9.17986928011506));
#40761=CARTESIAN_POINT('Ctrl Pts',(-32.6855914133007,24.4,-6.11991285341004));
#40762=CARTESIAN_POINT('Ctrl Pts',(-32.518924746634,24.4,0.));
#40763=CARTESIAN_POINT('Ctrl Pts',(-32.3522580799673,24.4,6.11991285341003));
#40764=CARTESIAN_POINT('Ctrl Pts',(-32.1855914133007,29.7,9.17986928011504));
#40765=CARTESIAN_POINT('Ctrl Pts',(-32.018924746634,35.,12.2398257068201));
#40766=CARTESIAN_POINT('Ctrl Pts',(-31.8522580799674,40.3,9.17986928011504));
#40767=CARTESIAN_POINT('Ctrl Pts',(-31.6855914133007,45.6,6.11991285341004));
#40768=CARTESIAN_POINT('Ctrl Pts',(-31.518924746634,45.6,1.29812560709619E-15));
#40769=CARTESIAN_POINT('Ctrl Pts',(-31.3522580799673,45.6,-6.11991285341003));
#40770=CARTESIAN_POINT('Ctrl Pts',(-31.1855914133007,40.3,-9.17986928011504));
#40771=CARTESIAN_POINT('Ctrl Pts',(-31.018924746634,35.,-12.2398257068201));
#40772=CARTESIAN_POINT('Ctrl Pts',(-30.8522580799673,29.7,-9.17986928011506));
#40773=CARTESIAN_POINT('Ctrl Pts',(-30.6855914133007,24.4,-6.11991285341004));
#40774=CARTESIAN_POINT('Ctrl Pts',(-30.518924746634,24.4,0.));
#40775=CARTESIAN_POINT('Ctrl Pts',(-30.3522580799673,24.4,6.11991285341003));
#40776=CARTESIAN_POINT('Ctrl Pts',(-30.1855914133007,29.7,9.17986928011504));
#40777=CARTESIAN_POINT('Ctrl Pts',(-30.018924746634,35.,12.2398257068201));
#40778=CARTESIAN_POINT('Ctrl Pts',(-29.8522580799673,40.3,9.17986928011504));
#40779=CARTESIAN_POINT('Ctrl Pts',(-29.6855914133007,45.6,6.11991285341004));
#40780=CARTESIAN_POINT('Ctrl Pts',(-29.518924746634,45.6,1.29812560709619E-15));
#40781=CARTESIAN_POINT('Ctrl Pts',(-29.3522580799673,45.6,-6.11991285341003));
#40782=CARTESIAN_POINT('Ctrl Pts',(-29.1855914133007,40.3,-9.17986928011504));
#40783=CARTESIAN_POINT('Ctrl Pts',(-29.018924746634,35.,-12.2398257068201));
#40784=CARTESIAN_POINT('Ctrl Pts',(-28.8522580799673,29.7,-9.17986928011506));
#40785=CARTESIAN_POINT('Ctrl Pts',(-28.6855914133007,24.4,-6.11991285341004));
#40786=CARTESIAN_POINT('Ctrl Pts',(-28.518924746634,24.4,0.));
#40787=CARTESIAN_POINT('Ctrl Pts',(-28.3522580799673,24.4,6.11991285341003));
#40788=CARTESIAN_POINT('Ctrl Pts',(-28.1855914133007,29.7,9.17986928011504));
#40789=CARTESIAN_POINT('Ctrl Pts',(-28.018924746634,35.,12.2398257068201));
#40790=CARTESIAN_POINT('Ctrl Pts',(-27.8522580799673,40.3,9.17986928011504));
#40791=CARTESIAN_POINT('Ctrl Pts',(-27.6855914133007,45.6,6.11991285341004));
#40792=CARTESIAN_POINT('Ctrl Pts',(-27.518924746634,45.6,1.29812560709619E-15));
#40793=CARTESIAN_POINT('Ctrl Pts',(-27.3522580799673,45.6,-6.11991285341003));
#40794=CARTESIAN_POINT('Ctrl Pts',(-27.1855914133007,40.3,-9.17986928011504));
#40795=CARTESIAN_POINT('Ctrl Pts',(-27.018924746634,35.,-12.2398257068201));
#40796=CARTESIAN_POINT('Ctrl Pts',(-26.8522580799673,29.7,-9.17986928011506));
#40797=CARTESIAN_POINT('Ctrl Pts',(-26.6855914133007,24.4,-6.11991285341004));
#40798=CARTESIAN_POINT('Ctrl Pts',(-26.518924746634,24.4,0.));
#40799=CARTESIAN_POINT('Ctrl Pts',(-26.3522580799673,24.4,6.11991285341003));
#40800=CARTESIAN_POINT('Ctrl Pts',(-26.1855914133007,29.7,9.17986928011504));
#40801=CARTESIAN_POINT('Ctrl Pts',(-26.018924746634,35.,12.2398257068201));
#40802=CARTESIAN_POINT('Ctrl Pts',(-25.8522580799673,40.3,9.17986928011504));
#40803=CARTESIAN_POINT('Ctrl Pts',(-25.6855914133007,45.6,6.11991285341004));
#40804=CARTESIAN_POINT('Ctrl Pts',(-25.518924746634,45.6,1.29812560709619E-15));
#40805=CARTESIAN_POINT('Ctrl Pts',(-25.3522580799673,45.6,-6.11991285341003));
#40806=CARTESIAN_POINT('Ctrl Pts',(-25.1855914133007,40.3,-9.17986928011504));
#40807=CARTESIAN_POINT('Ctrl Pts',(-25.018924746634,35.,-12.2398257068201));
#40808=CARTESIAN_POINT('Ctrl Pts',(-24.8522580799673,29.7,-9.17986928011506));
#40809=CARTESIAN_POINT('Ctrl Pts',(-24.6855914133007,24.4,-6.11991285341004));
#40810=CARTESIAN_POINT('Ctrl Pts',(-24.518924746634,24.4,0.));
#40811=CARTESIAN_POINT('Ctrl Pts',(-24.3522580799673,24.4,6.11991285341003));
#40812=CARTESIAN_POINT('Ctrl Pts',(-24.1855914133007,29.7,9.17986928011504));
#40813=CARTESIAN_POINT('Ctrl Pts',(-24.018924746634,35.,12.2398257068201));
#40814=CARTESIAN_POINT('Ctrl Pts',(-23.8522580799674,40.3,9.17986928011504));
#40815=CARTESIAN_POINT('Ctrl Pts',(-23.6855914133007,45.6,6.11991285341004));
#40816=CARTESIAN_POINT('Ctrl Pts',(-23.518924746634,45.6,1.29812560709619E-15));
#40817=CARTESIAN_POINT('Ctrl Pts',(-23.3522580799673,45.6,-6.11991285341003));
#40818=CARTESIAN_POINT('Ctrl Pts',(-23.1855914133007,40.3,-9.17986928011504));
#40819=CARTESIAN_POINT('Ctrl Pts',(-23.018924746634,35.,-12.2398257068201));
#40820=CARTESIAN_POINT('Ctrl Pts',(-22.8522580799673,29.7,-9.17986928011506));
#40821=CARTESIAN_POINT('Ctrl Pts',(-22.6855914133007,24.4,-6.11991285341004));
#40822=CARTESIAN_POINT('Ctrl Pts',(-22.518924746634,24.4,0.));
#40823=CARTESIAN_POINT('Ctrl Pts',(-22.3522580799673,24.4,6.11991285341003));
#40824=CARTESIAN_POINT('Ctrl Pts',(-22.1855914133007,29.7,9.17986928011504));
#40825=CARTESIAN_POINT('Ctrl Pts',(-22.018924746634,35.,12.2398257068201));
#40826=CARTESIAN_POINT('Ctrl Pts',(-21.8522580799673,40.3,9.17986928011504));
#40827=CARTESIAN_POINT('Ctrl Pts',(-21.6855914133007,45.6,6.11991285341004));
#40828=CARTESIAN_POINT('Ctrl Pts',(-21.518924746634,45.6,1.29812560709619E-15));
#40829=CARTESIAN_POINT('Ctrl Pts',(-21.3522580799673,45.6,-6.11991285341003));
#40830=CARTESIAN_POINT('Ctrl Pts',(-21.1855914133007,40.3,-9.17986928011504));
#40831=CARTESIAN_POINT('Ctrl Pts',(-21.018924746634,35.,-12.2398257068201));
#40832=CARTESIAN_POINT('Ctrl Pts',(-20.8522580799674,29.7,-9.17986928011506));
#40833=CARTESIAN_POINT('Ctrl Pts',(-20.6855914133006,24.4,-6.11991285341004));
#40834=CARTESIAN_POINT('Ctrl Pts',(-20.518924746634,24.4,0.));
#40835=CARTESIAN_POINT('Ctrl Pts',(-20.3522580799673,24.4,6.11991285341003));
#40836=CARTESIAN_POINT('Ctrl Pts',(-20.1855914133007,29.7,9.17986928011504));
#40837=CARTESIAN_POINT('Ctrl Pts',(-20.018924746634,35.,12.2398257068201));
#40838=CARTESIAN_POINT('Ctrl Pts',(-19.8522580799673,40.3,9.17986928011504));
#40839=CARTESIAN_POINT('Ctrl Pts',(-19.6855914133007,45.6,6.11991285341004));
#40840=CARTESIAN_POINT('Ctrl Pts',(-19.518924746634,45.6,1.29812560709619E-15));
#40841=CARTESIAN_POINT('Ctrl Pts',(-19.3522580799673,45.6,-6.11991285341003));
#40842=CARTESIAN_POINT('Ctrl Pts',(-19.1855914133007,40.3,-9.17986928011504));
#40843=CARTESIAN_POINT('Ctrl Pts',(-19.018924746634,35.,-12.2398257068201));
#40844=CARTESIAN_POINT('Ctrl Pts',(-18.8522580799673,29.7,-9.17986928011506));
#40845=CARTESIAN_POINT('Ctrl Pts',(-18.6855914133007,24.4,-6.11991285341004));
#40846=CARTESIAN_POINT('Ctrl Pts',(-18.518924746634,24.4,0.));
#40847=CARTESIAN_POINT('Ctrl Pts',(-38.518924746634,26.,0.));
#40848=CARTESIAN_POINT('Ctrl Pts',(-38.3522580799673,26.,5.19615242270663));
#40849=CARTESIAN_POINT('Ctrl Pts',(-38.1855914133007,30.5,7.79422863405995));
#40850=CARTESIAN_POINT('Ctrl Pts',(-38.018924746634,35.,10.3923048454133));
#40851=CARTESIAN_POINT('Ctrl Pts',(-37.8522580799673,39.5,7.79422863405995));
#40852=CARTESIAN_POINT('Ctrl Pts',(-37.6855914133007,44.,5.19615242270663));
#40853=CARTESIAN_POINT('Ctrl Pts',(-37.518924746634,44.,1.10218211923262E-15));
#40854=CARTESIAN_POINT('Ctrl Pts',(-37.3522580799673,44.,-5.19615242270663));
#40855=CARTESIAN_POINT('Ctrl Pts',(-37.1855914133007,39.5,-7.79422863405995));
#40856=CARTESIAN_POINT('Ctrl Pts',(-37.018924746634,35.,-10.3923048454133));
#40857=CARTESIAN_POINT('Ctrl Pts',(-36.8522580799673,30.5,-7.79422863405995));
#40858=CARTESIAN_POINT('Ctrl Pts',(-36.6855914133007,26.,-5.19615242270663));
#40859=CARTESIAN_POINT('Ctrl Pts',(-36.518924746634,26.,0.));
#40860=CARTESIAN_POINT('Ctrl Pts',(-36.3522580799673,26.,5.19615242270663));
#40861=CARTESIAN_POINT('Ctrl Pts',(-36.1855914133007,30.5,7.79422863405995));
#40862=CARTESIAN_POINT('Ctrl Pts',(-36.018924746634,35.,10.3923048454133));
#40863=CARTESIAN_POINT('Ctrl Pts',(-35.8522580799673,39.5,7.79422863405995));
#40864=CARTESIAN_POINT('Ctrl Pts',(-35.6855914133007,44.,5.19615242270663));
#40865=CARTESIAN_POINT('Ctrl Pts',(-35.518924746634,44.,1.10218211923262E-15));
#40866=CARTESIAN_POINT('Ctrl Pts',(-35.3522580799673,44.,-5.19615242270663));
#40867=CARTESIAN_POINT('Ctrl Pts',(-35.1855914133007,39.5,-7.79422863405995));
#40868=CARTESIAN_POINT('Ctrl Pts',(-35.018924746634,35.,-10.3923048454133));
#40869=CARTESIAN_POINT('Ctrl Pts',(-34.8522580799673,30.5,-7.79422863405995));
#40870=CARTESIAN_POINT('Ctrl Pts',(-34.6855914133007,26.,-5.19615242270663));
#40871=CARTESIAN_POINT('Ctrl Pts',(-34.518924746634,26.,0.));
#40872=CARTESIAN_POINT('Ctrl Pts',(-34.3522580799673,26.,5.19615242270663));
#40873=CARTESIAN_POINT('Ctrl Pts',(-34.1855914133007,30.5,7.79422863405995));
#40874=CARTESIAN_POINT('Ctrl Pts',(-34.018924746634,35.,10.3923048454133));
#40875=CARTESIAN_POINT('Ctrl Pts',(-33.8522580799673,39.5,7.79422863405995));
#40876=CARTESIAN_POINT('Ctrl Pts',(-33.6855914133007,44.,5.19615242270663));
#40877=CARTESIAN_POINT('Ctrl Pts',(-33.518924746634,44.,1.10218211923262E-15));
#40878=CARTESIAN_POINT('Ctrl Pts',(-33.3522580799673,44.,-5.19615242270663));
#40879=CARTESIAN_POINT('Ctrl Pts',(-33.1855914133007,39.5,-7.79422863405995));
#40880=CARTESIAN_POINT('Ctrl Pts',(-33.018924746634,35.,-10.3923048454133));
#40881=CARTESIAN_POINT('Ctrl Pts',(-32.8522580799673,30.5,-7.79422863405995));
#40882=CARTESIAN_POINT('Ctrl Pts',(-32.6855914133007,26.,-5.19615242270663));
#40883=CARTESIAN_POINT('Ctrl Pts',(-32.518924746634,26.,0.));
#40884=CARTESIAN_POINT('Ctrl Pts',(-32.3522580799673,26.,5.19615242270663));
#40885=CARTESIAN_POINT('Ctrl Pts',(-32.1855914133007,30.5,7.79422863405995));
#40886=CARTESIAN_POINT('Ctrl Pts',(-32.018924746634,35.,10.3923048454133));
#40887=CARTESIAN_POINT('Ctrl Pts',(-31.8522580799673,39.5,7.79422863405995));
#40888=CARTESIAN_POINT('Ctrl Pts',(-31.6855914133007,44.,5.19615242270663));
#40889=CARTESIAN_POINT('Ctrl Pts',(-31.518924746634,44.,1.10218211923262E-15));
#40890=CARTESIAN_POINT('Ctrl Pts',(-31.3522580799673,44.,-5.19615242270663));
#40891=CARTESIAN_POINT('Ctrl Pts',(-31.1855914133007,39.5,-7.79422863405995));
#40892=CARTESIAN_POINT('Ctrl Pts',(-31.018924746634,35.,-10.3923048454133));
#40893=CARTESIAN_POINT('Ctrl Pts',(-30.8522580799673,30.5,-7.79422863405995));
#40894=CARTESIAN_POINT('Ctrl Pts',(-30.6855914133007,26.,-5.19615242270663));
#40895=CARTESIAN_POINT('Ctrl Pts',(-30.518924746634,26.,0.));
#40896=CARTESIAN_POINT('Ctrl Pts',(-30.3522580799673,26.,5.19615242270663));
#40897=CARTESIAN_POINT('Ctrl Pts',(-30.1855914133007,30.5,7.79422863405995));
#40898=CARTESIAN_POINT('Ctrl Pts',(-30.018924746634,35.,10.3923048454133));
#40899=CARTESIAN_POINT('Ctrl Pts',(-29.8522580799673,39.5,7.79422863405995));
#40900=CARTESIAN_POINT('Ctrl Pts',(-29.6855914133007,44.,5.19615242270663));
#40901=CARTESIAN_POINT('Ctrl Pts',(-29.518924746634,44.,1.10218211923262E-15));
#40902=CARTESIAN_POINT('Ctrl Pts',(-29.3522580799673,44.,-5.19615242270663));
#40903=CARTESIAN_POINT('Ctrl Pts',(-29.1855914133007,39.5,-7.79422863405995));
#40904=CARTESIAN_POINT('Ctrl Pts',(-29.018924746634,35.,-10.3923048454133));
#40905=CARTESIAN_POINT('Ctrl Pts',(-28.8522580799673,30.5,-7.79422863405995));
#40906=CARTESIAN_POINT('Ctrl Pts',(-28.6855914133007,26.,-5.19615242270663));
#40907=CARTESIAN_POINT('Ctrl Pts',(-28.518924746634,26.,0.));
#40908=CARTESIAN_POINT('Ctrl Pts',(-28.3522580799673,26.,5.19615242270663));
#40909=CARTESIAN_POINT('Ctrl Pts',(-28.1855914133007,30.5,7.79422863405995));
#40910=CARTESIAN_POINT('Ctrl Pts',(-28.018924746634,35.,10.3923048454133));
#40911=CARTESIAN_POINT('Ctrl Pts',(-27.8522580799673,39.5,7.79422863405995));
#40912=CARTESIAN_POINT('Ctrl Pts',(-27.6855914133007,44.,5.19615242270663));
#40913=CARTESIAN_POINT('Ctrl Pts',(-27.518924746634,44.,1.10218211923262E-15));
#40914=CARTESIAN_POINT('Ctrl Pts',(-27.3522580799673,44.,-5.19615242270663));
#40915=CARTESIAN_POINT('Ctrl Pts',(-27.1855914133007,39.5,-7.79422863405995));
#40916=CARTESIAN_POINT('Ctrl Pts',(-27.018924746634,35.,-10.3923048454133));
#40917=CARTESIAN_POINT('Ctrl Pts',(-26.8522580799673,30.5,-7.79422863405995));
#40918=CARTESIAN_POINT('Ctrl Pts',(-26.6855914133007,26.,-5.19615242270663));
#40919=CARTESIAN_POINT('Ctrl Pts',(-26.518924746634,26.,0.));
#40920=CARTESIAN_POINT('Ctrl Pts',(-26.3522580799673,26.,5.19615242270663));
#40921=CARTESIAN_POINT('Ctrl Pts',(-26.1855914133007,30.5,7.79422863405995));
#40922=CARTESIAN_POINT('Ctrl Pts',(-26.018924746634,35.,10.3923048454133));
#40923=CARTESIAN_POINT('Ctrl Pts',(-25.8522580799673,39.5,7.79422863405995));
#40924=CARTESIAN_POINT('Ctrl Pts',(-25.6855914133007,44.,5.19615242270663));
#40925=CARTESIAN_POINT('Ctrl Pts',(-25.518924746634,44.,1.10218211923262E-15));
#40926=CARTESIAN_POINT('Ctrl Pts',(-25.3522580799673,44.,-5.19615242270663));
#40927=CARTESIAN_POINT('Ctrl Pts',(-25.1855914133007,39.5,-7.79422863405995));
#40928=CARTESIAN_POINT('Ctrl Pts',(-25.018924746634,35.,-10.3923048454133));
#40929=CARTESIAN_POINT('Ctrl Pts',(-24.8522580799673,30.5,-7.79422863405995));
#40930=CARTESIAN_POINT('Ctrl Pts',(-24.6855914133007,26.,-5.19615242270663));
#40931=CARTESIAN_POINT('Ctrl Pts',(-24.518924746634,26.,0.));
#40932=CARTESIAN_POINT('Ctrl Pts',(-24.3522580799673,26.,5.19615242270663));
#40933=CARTESIAN_POINT('Ctrl Pts',(-24.1855914133007,30.5,7.79422863405995));
#40934=CARTESIAN_POINT('Ctrl Pts',(-24.018924746634,35.,10.3923048454133));
#40935=CARTESIAN_POINT('Ctrl Pts',(-23.8522580799673,39.5,7.79422863405995));
#40936=CARTESIAN_POINT('Ctrl Pts',(-23.6855914133007,44.,5.19615242270663));
#40937=CARTESIAN_POINT('Ctrl Pts',(-23.518924746634,44.,1.10218211923262E-15));
#40938=CARTESIAN_POINT('Ctrl Pts',(-23.3522580799673,44.,-5.19615242270663));
#40939=CARTESIAN_POINT('Ctrl Pts',(-23.1855914133007,39.5,-7.79422863405995));
#40940=CARTESIAN_POINT('Ctrl Pts',(-23.018924746634,35.,-10.3923048454133));
#40941=CARTESIAN_POINT('Ctrl Pts',(-22.8522580799673,30.5,-7.79422863405995));
#40942=CARTESIAN_POINT('Ctrl Pts',(-22.6855914133007,26.,-5.19615242270663));
#40943=CARTESIAN_POINT('Ctrl Pts',(-22.518924746634,26.,0.));
#40944=CARTESIAN_POINT('Ctrl Pts',(-22.3522580799673,26.,5.19615242270663));
#40945=CARTESIAN_POINT('Ctrl Pts',(-22.1855914133007,30.5,7.79422863405995));
#40946=CARTESIAN_POINT('Ctrl Pts',(-22.018924746634,35.,10.3923048454133));
#40947=CARTESIAN_POINT('Ctrl Pts',(-21.8522580799673,39.5,7.79422863405995));
#40948=CARTESIAN_POINT('Ctrl Pts',(-21.6855914133007,44.,5.19615242270663));
#40949=CARTESIAN_POINT('Ctrl Pts',(-21.518924746634,44.,1.10218211923262E-15));
#40950=CARTESIAN_POINT('Ctrl Pts',(-21.3522580799673,44.,-5.19615242270663));
#40951=CARTESIAN_POINT('Ctrl Pts',(-21.1855914133006,39.5,-7.79422863405995));
#40952=CARTESIAN_POINT('Ctrl Pts',(-21.018924746634,35.,-10.3923048454133));
#40953=CARTESIAN_POINT('Ctrl Pts',(-20.8522580799673,30.5,-7.79422863405995));
#40954=CARTESIAN_POINT('Ctrl Pts',(-20.6855914133007,26.,-5.19615242270663));
#40955=CARTESIAN_POINT('Ctrl Pts',(-20.518924746634,26.,0.));
#40956=CARTESIAN_POINT('Ctrl Pts',(-20.3522580799673,26.,5.19615242270663));
#40957=CARTESIAN_POINT('Ctrl Pts',(-20.1855914133006,30.5,7.79422863405995));
#40958=CARTESIAN_POINT('Ctrl Pts',(-20.018924746634,35.,10.3923048454133));
#40959=CARTESIAN_POINT('Ctrl Pts',(-19.8522580799674,39.5,7.79422863405995));
#40960=CARTESIAN_POINT('Ctrl Pts',(-19.6855914133006,44.,5.19615242270663));
#40961=CARTESIAN_POINT('Ctrl Pts',(-19.518924746634,44.,1.10218211923262E-15));
#40962=CARTESIAN_POINT('Ctrl Pts',(-19.3522580799673,44.,-5.19615242270663));
#40963=CARTESIAN_POINT('Ctrl Pts',(-19.1855914133007,39.5,-7.79422863405995));
#40964=CARTESIAN_POINT('Ctrl Pts',(-19.018924746634,35.,-10.3923048454133));
#40965=CARTESIAN_POINT('Ctrl Pts',(-18.8522580799674,30.5,-7.79422863405995));
#40966=CARTESIAN_POINT('Ctrl Pts',(-18.6855914133007,26.,-5.19615242270663));
#40967=CARTESIAN_POINT('Ctrl Pts',(-18.518924746634,26.,0.));
#40968=CARTESIAN_POINT('Ctrl Pts',(-38.518924746634,27.6,0.));
#40969=CARTESIAN_POINT('Ctrl Pts',(-38.3522580799673,27.6,4.27239199200323));
#40970=CARTESIAN_POINT('Ctrl Pts',(-38.1855914133007,31.3,6.40858798800485));
#40971=CARTESIAN_POINT('Ctrl Pts',(-38.018924746634,35.,8.54478398400645));
#40972=CARTESIAN_POINT('Ctrl Pts',(-37.8522580799673,38.7,6.40858798800485));
#40973=CARTESIAN_POINT('Ctrl Pts',(-37.6855914133007,42.4,4.27239199200323));
#40974=CARTESIAN_POINT('Ctrl Pts',(-37.518924746634,42.4,9.06238631369041E-16));
#40975=CARTESIAN_POINT('Ctrl Pts',(-37.3522580799673,42.4,-4.27239199200323));
#40976=CARTESIAN_POINT('Ctrl Pts',(-37.1855914133007,38.7,-6.40858798800485));
#40977=CARTESIAN_POINT('Ctrl Pts',(-37.018924746634,35.,-8.54478398400645));
#40978=CARTESIAN_POINT('Ctrl Pts',(-36.8522580799673,31.3,-6.40858798800485));
#40979=CARTESIAN_POINT('Ctrl Pts',(-36.6855914133007,27.6,-4.27239199200323));
#40980=CARTESIAN_POINT('Ctrl Pts',(-36.518924746634,27.6,0.));
#40981=CARTESIAN_POINT('Ctrl Pts',(-36.3522580799673,27.6,4.27239199200323));
#40982=CARTESIAN_POINT('Ctrl Pts',(-36.1855914133007,31.3,6.40858798800485));
#40983=CARTESIAN_POINT('Ctrl Pts',(-36.018924746634,35.,8.54478398400645));
#40984=CARTESIAN_POINT('Ctrl Pts',(-35.8522580799673,38.7,6.40858798800485));
#40985=CARTESIAN_POINT('Ctrl Pts',(-35.6855914133007,42.4,4.27239199200323));
#40986=CARTESIAN_POINT('Ctrl Pts',(-35.518924746634,42.4,9.06238631369041E-16));
#40987=CARTESIAN_POINT('Ctrl Pts',(-35.3522580799673,42.4,-4.27239199200323));
#40988=CARTESIAN_POINT('Ctrl Pts',(-35.1855914133007,38.7,-6.40858798800485));
#40989=CARTESIAN_POINT('Ctrl Pts',(-35.018924746634,35.,-8.54478398400645));
#40990=CARTESIAN_POINT('Ctrl Pts',(-34.8522580799673,31.3,-6.40858798800485));
#40991=CARTESIAN_POINT('Ctrl Pts',(-34.6855914133007,27.6,-4.27239199200323));
#40992=CARTESIAN_POINT('Ctrl Pts',(-34.518924746634,27.6,0.));
#40993=CARTESIAN_POINT('Ctrl Pts',(-34.3522580799673,27.6,4.27239199200323));
#40994=CARTESIAN_POINT('Ctrl Pts',(-34.1855914133007,31.3,6.40858798800485));
#40995=CARTESIAN_POINT('Ctrl Pts',(-34.018924746634,35.,8.54478398400645));
#40996=CARTESIAN_POINT('Ctrl Pts',(-33.8522580799673,38.7,6.40858798800485));
#40997=CARTESIAN_POINT('Ctrl Pts',(-33.6855914133007,42.4,4.27239199200323));
#40998=CARTESIAN_POINT('Ctrl Pts',(-33.518924746634,42.4,9.06238631369041E-16));
#40999=CARTESIAN_POINT('Ctrl Pts',(-33.3522580799673,42.4,-4.27239199200323));
#41000=CARTESIAN_POINT('Ctrl Pts',(-33.1855914133007,38.7,-6.40858798800485));
#41001=CARTESIAN_POINT('Ctrl Pts',(-33.018924746634,35.,-8.54478398400645));
#41002=CARTESIAN_POINT('Ctrl Pts',(-32.8522580799673,31.3,-6.40858798800485));
#41003=CARTESIAN_POINT('Ctrl Pts',(-32.6855914133007,27.6,-4.27239199200323));
#41004=CARTESIAN_POINT('Ctrl Pts',(-32.518924746634,27.6,0.));
#41005=CARTESIAN_POINT('Ctrl Pts',(-32.3522580799673,27.6,4.27239199200323));
#41006=CARTESIAN_POINT('Ctrl Pts',(-32.1855914133007,31.3,6.40858798800485));
#41007=CARTESIAN_POINT('Ctrl Pts',(-32.018924746634,35.,8.54478398400645));
#41008=CARTESIAN_POINT('Ctrl Pts',(-31.8522580799674,38.7,6.40858798800485));
#41009=CARTESIAN_POINT('Ctrl Pts',(-31.6855914133007,42.4,4.27239199200323));
#41010=CARTESIAN_POINT('Ctrl Pts',(-31.518924746634,42.4,9.06238631369041E-16));
#41011=CARTESIAN_POINT('Ctrl Pts',(-31.3522580799673,42.4,-4.27239199200323));
#41012=CARTESIAN_POINT('Ctrl Pts',(-31.1855914133007,38.7,-6.40858798800485));
#41013=CARTESIAN_POINT('Ctrl Pts',(-31.018924746634,35.,-8.54478398400645));
#41014=CARTESIAN_POINT('Ctrl Pts',(-30.8522580799673,31.3,-6.40858798800485));
#41015=CARTESIAN_POINT('Ctrl Pts',(-30.6855914133007,27.6,-4.27239199200323));
#41016=CARTESIAN_POINT('Ctrl Pts',(-30.518924746634,27.6,0.));
#41017=CARTESIAN_POINT('Ctrl Pts',(-30.3522580799673,27.6,4.27239199200323));
#41018=CARTESIAN_POINT('Ctrl Pts',(-30.1855914133007,31.3,6.40858798800485));
#41019=CARTESIAN_POINT('Ctrl Pts',(-30.018924746634,35.,8.54478398400645));
#41020=CARTESIAN_POINT('Ctrl Pts',(-29.8522580799673,38.7,6.40858798800485));
#41021=CARTESIAN_POINT('Ctrl Pts',(-29.6855914133007,42.4,4.27239199200323));
#41022=CARTESIAN_POINT('Ctrl Pts',(-29.518924746634,42.4,9.06238631369041E-16));
#41023=CARTESIAN_POINT('Ctrl Pts',(-29.3522580799673,42.4,-4.27239199200323));
#41024=CARTESIAN_POINT('Ctrl Pts',(-29.1855914133007,38.7,-6.40858798800485));
#41025=CARTESIAN_POINT('Ctrl Pts',(-29.018924746634,35.,-8.54478398400645));
#41026=CARTESIAN_POINT('Ctrl Pts',(-28.8522580799673,31.3,-6.40858798800485));
#41027=CARTESIAN_POINT('Ctrl Pts',(-28.6855914133007,27.6,-4.27239199200323));
#41028=CARTESIAN_POINT('Ctrl Pts',(-28.518924746634,27.6,0.));
#41029=CARTESIAN_POINT('Ctrl Pts',(-28.3522580799673,27.6,4.27239199200323));
#41030=CARTESIAN_POINT('Ctrl Pts',(-28.1855914133007,31.3,6.40858798800485));
#41031=CARTESIAN_POINT('Ctrl Pts',(-28.018924746634,35.,8.54478398400645));
#41032=CARTESIAN_POINT('Ctrl Pts',(-27.8522580799673,38.7,6.40858798800485));
#41033=CARTESIAN_POINT('Ctrl Pts',(-27.6855914133007,42.4,4.27239199200323));
#41034=CARTESIAN_POINT('Ctrl Pts',(-27.518924746634,42.4,9.06238631369041E-16));
#41035=CARTESIAN_POINT('Ctrl Pts',(-27.3522580799673,42.4,-4.27239199200323));
#41036=CARTESIAN_POINT('Ctrl Pts',(-27.1855914133007,38.7,-6.40858798800485));
#41037=CARTESIAN_POINT('Ctrl Pts',(-27.018924746634,35.,-8.54478398400645));
#41038=CARTESIAN_POINT('Ctrl Pts',(-26.8522580799673,31.3,-6.40858798800485));
#41039=CARTESIAN_POINT('Ctrl Pts',(-26.6855914133007,27.6,-4.27239199200323));
#41040=CARTESIAN_POINT('Ctrl Pts',(-26.518924746634,27.6,0.));
#41041=CARTESIAN_POINT('Ctrl Pts',(-26.3522580799673,27.6,4.27239199200323));
#41042=CARTESIAN_POINT('Ctrl Pts',(-26.1855914133007,31.3,6.40858798800485));
#41043=CARTESIAN_POINT('Ctrl Pts',(-26.018924746634,35.,8.54478398400645));
#41044=CARTESIAN_POINT('Ctrl Pts',(-25.8522580799673,38.7,6.40858798800485));
#41045=CARTESIAN_POINT('Ctrl Pts',(-25.6855914133007,42.4,4.27239199200323));
#41046=CARTESIAN_POINT('Ctrl Pts',(-25.518924746634,42.4,9.06238631369041E-16));
#41047=CARTESIAN_POINT('Ctrl Pts',(-25.3522580799673,42.4,-4.27239199200323));
#41048=CARTESIAN_POINT('Ctrl Pts',(-25.1855914133007,38.7,-6.40858798800485));
#41049=CARTESIAN_POINT('Ctrl Pts',(-25.018924746634,35.,-8.54478398400645));
#41050=CARTESIAN_POINT('Ctrl Pts',(-24.8522580799673,31.3,-6.40858798800485));
#41051=CARTESIAN_POINT('Ctrl Pts',(-24.6855914133007,27.6,-4.27239199200323));
#41052=CARTESIAN_POINT('Ctrl Pts',(-24.518924746634,27.6,0.));
#41053=CARTESIAN_POINT('Ctrl Pts',(-24.3522580799673,27.6,4.27239199200323));
#41054=CARTESIAN_POINT('Ctrl Pts',(-24.1855914133007,31.3,6.40858798800485));
#41055=CARTESIAN_POINT('Ctrl Pts',(-24.018924746634,35.,8.54478398400645));
#41056=CARTESIAN_POINT('Ctrl Pts',(-23.8522580799674,38.7,6.40858798800485));
#41057=CARTESIAN_POINT('Ctrl Pts',(-23.6855914133007,42.4,4.27239199200323));
#41058=CARTESIAN_POINT('Ctrl Pts',(-23.518924746634,42.4,9.06238631369041E-16));
#41059=CARTESIAN_POINT('Ctrl Pts',(-23.3522580799673,42.4,-4.27239199200323));
#41060=CARTESIAN_POINT('Ctrl Pts',(-23.1855914133007,38.7,-6.40858798800485));
#41061=CARTESIAN_POINT('Ctrl Pts',(-23.018924746634,35.,-8.54478398400645));
#41062=CARTESIAN_POINT('Ctrl Pts',(-22.8522580799673,31.3,-6.40858798800485));
#41063=CARTESIAN_POINT('Ctrl Pts',(-22.6855914133007,27.6,-4.27239199200323));
#41064=CARTESIAN_POINT('Ctrl Pts',(-22.518924746634,27.6,0.));
#41065=CARTESIAN_POINT('Ctrl Pts',(-22.3522580799673,27.6,4.27239199200323));
#41066=CARTESIAN_POINT('Ctrl Pts',(-22.1855914133007,31.3,6.40858798800485));
#41067=CARTESIAN_POINT('Ctrl Pts',(-22.018924746634,35.,8.54478398400645));
#41068=CARTESIAN_POINT('Ctrl Pts',(-21.8522580799673,38.7,6.40858798800485));
#41069=CARTESIAN_POINT('Ctrl Pts',(-21.6855914133007,42.4,4.27239199200323));
#41070=CARTESIAN_POINT('Ctrl Pts',(-21.518924746634,42.4,9.06238631369041E-16));
#41071=CARTESIAN_POINT('Ctrl Pts',(-21.3522580799673,42.4,-4.27239199200323));
#41072=CARTESIAN_POINT('Ctrl Pts',(-21.1855914133007,38.7,-6.40858798800485));
#41073=CARTESIAN_POINT('Ctrl Pts',(-21.018924746634,35.,-8.54478398400645));
#41074=CARTESIAN_POINT('Ctrl Pts',(-20.8522580799674,31.3,-6.40858798800485));
#41075=CARTESIAN_POINT('Ctrl Pts',(-20.6855914133006,27.6,-4.27239199200323));
#41076=CARTESIAN_POINT('Ctrl Pts',(-20.518924746634,27.6,0.));
#41077=CARTESIAN_POINT('Ctrl Pts',(-20.3522580799673,27.6,4.27239199200323));
#41078=CARTESIAN_POINT('Ctrl Pts',(-20.1855914133007,31.3,6.40858798800485));
#41079=CARTESIAN_POINT('Ctrl Pts',(-20.018924746634,35.,8.54478398400645));
#41080=CARTESIAN_POINT('Ctrl Pts',(-19.8522580799673,38.7,6.40858798800485));
#41081=CARTESIAN_POINT('Ctrl Pts',(-19.6855914133007,42.4,4.27239199200323));
#41082=CARTESIAN_POINT('Ctrl Pts',(-19.518924746634,42.4,9.06238631369041E-16));
#41083=CARTESIAN_POINT('Ctrl Pts',(-19.3522580799673,42.4,-4.27239199200323));
#41084=CARTESIAN_POINT('Ctrl Pts',(-19.1855914133007,38.7,-6.40858798800485));
#41085=CARTESIAN_POINT('Ctrl Pts',(-19.018924746634,35.,-8.54478398400645));
#41086=CARTESIAN_POINT('Ctrl Pts',(-18.8522580799673,31.3,-6.40858798800485));
#41087=CARTESIAN_POINT('Ctrl Pts',(-18.6855914133007,27.6,-4.27239199200323));
#41088=CARTESIAN_POINT('Ctrl Pts',(-18.518924746634,27.6,0.));
#41089=CARTESIAN_POINT('Ctrl Pts',(-36.918924746634,27.6,0.));
#41090=CARTESIAN_POINT('Ctrl Pts',(-36.7522580799673,27.6,4.27239199200323));
#41091=CARTESIAN_POINT('Ctrl Pts',(-36.5855914133007,31.3,6.40858798800485));
#41092=CARTESIAN_POINT('Ctrl Pts',(-36.418924746634,35.,8.54478398400645));
#41093=CARTESIAN_POINT('Ctrl Pts',(-36.2522580799673,38.7,6.40858798800485));
#41094=CARTESIAN_POINT('Ctrl Pts',(-36.0855914133007,42.4,4.27239199200323));
#41095=CARTESIAN_POINT('Ctrl Pts',(-35.918924746634,42.4,9.06238631369041E-16));
#41096=CARTESIAN_POINT('Ctrl Pts',(-35.7522580799673,42.4,-4.27239199200323));
#41097=CARTESIAN_POINT('Ctrl Pts',(-35.5855914133007,38.7,-6.40858798800485));
#41098=CARTESIAN_POINT('Ctrl Pts',(-35.418924746634,35.,-8.54478398400645));
#41099=CARTESIAN_POINT('Ctrl Pts',(-35.2522580799673,31.3,-6.40858798800485));
#41100=CARTESIAN_POINT('Ctrl Pts',(-35.0855914133007,27.6,-4.27239199200323));
#41101=CARTESIAN_POINT('Ctrl Pts',(-34.918924746634,27.6,0.));
#41102=CARTESIAN_POINT('Ctrl Pts',(-34.7522580799673,27.6,4.27239199200323));
#41103=CARTESIAN_POINT('Ctrl Pts',(-34.5855914133007,31.3,6.40858798800485));
#41104=CARTESIAN_POINT('Ctrl Pts',(-34.418924746634,35.,8.54478398400645));
#41105=CARTESIAN_POINT('Ctrl Pts',(-34.2522580799673,38.7,6.40858798800485));
#41106=CARTESIAN_POINT('Ctrl Pts',(-34.0855914133007,42.4,4.27239199200323));
#41107=CARTESIAN_POINT('Ctrl Pts',(-33.918924746634,42.4,9.06238631369041E-16));
#41108=CARTESIAN_POINT('Ctrl Pts',(-33.7522580799673,42.4,-4.27239199200323));
#41109=CARTESIAN_POINT('Ctrl Pts',(-33.5855914133007,38.7,-6.40858798800485));
#41110=CARTESIAN_POINT('Ctrl Pts',(-33.418924746634,35.,-8.54478398400645));
#41111=CARTESIAN_POINT('Ctrl Pts',(-33.2522580799673,31.3,-6.40858798800485));
#41112=CARTESIAN_POINT('Ctrl Pts',(-33.0855914133007,27.6,-4.27239199200323));
#41113=CARTESIAN_POINT('Ctrl Pts',(-32.918924746634,27.6,0.));
#41114=CARTESIAN_POINT('Ctrl Pts',(-32.7522580799673,27.6,4.27239199200323));
#41115=CARTESIAN_POINT('Ctrl Pts',(-32.5855914133007,31.3,6.40858798800485));
#41116=CARTESIAN_POINT('Ctrl Pts',(-32.418924746634,35.,8.54478398400645));
#41117=CARTESIAN_POINT('Ctrl Pts',(-32.2522580799673,38.7,6.40858798800485));
#41118=CARTESIAN_POINT('Ctrl Pts',(-32.0855914133007,42.4,4.27239199200323));
#41119=CARTESIAN_POINT('Ctrl Pts',(-31.918924746634,42.4,9.06238631369041E-16));
#41120=CARTESIAN_POINT('Ctrl Pts',(-31.7522580799673,42.4,-4.27239199200323));
#41121=CARTESIAN_POINT('Ctrl Pts',(-31.5855914133007,38.7,-6.40858798800485));
#41122=CARTESIAN_POINT('Ctrl Pts',(-31.418924746634,35.,-8.54478398400645));
#41123=CARTESIAN_POINT('Ctrl Pts',(-31.2522580799673,31.3,-6.40858798800485));
#41124=CARTESIAN_POINT('Ctrl Pts',(-31.0855914133007,27.6,-4.27239199200323));
#41125=CARTESIAN_POINT('Ctrl Pts',(-30.918924746634,27.6,0.));
#41126=CARTESIAN_POINT('Ctrl Pts',(-30.7522580799673,27.6,4.27239199200323));
#41127=CARTESIAN_POINT('Ctrl Pts',(-30.5855914133007,31.3,6.40858798800485));
#41128=CARTESIAN_POINT('Ctrl Pts',(-30.418924746634,35.,8.54478398400645));
#41129=CARTESIAN_POINT('Ctrl Pts',(-30.2522580799673,38.7,6.40858798800485));
#41130=CARTESIAN_POINT('Ctrl Pts',(-30.0855914133007,42.4,4.27239199200323));
#41131=CARTESIAN_POINT('Ctrl Pts',(-29.918924746634,42.4,9.06238631369041E-16));
#41132=CARTESIAN_POINT('Ctrl Pts',(-29.7522580799673,42.4,-4.27239199200323));
#41133=CARTESIAN_POINT('Ctrl Pts',(-29.5855914133007,38.7,-6.40858798800485));
#41134=CARTESIAN_POINT('Ctrl Pts',(-29.418924746634,35.,-8.54478398400645));
#41135=CARTESIAN_POINT('Ctrl Pts',(-29.2522580799673,31.3,-6.40858798800485));
#41136=CARTESIAN_POINT('Ctrl Pts',(-29.0855914133007,27.6,-4.27239199200323));
#41137=CARTESIAN_POINT('Ctrl Pts',(-28.918924746634,27.6,0.));
#41138=CARTESIAN_POINT('Ctrl Pts',(-28.7522580799673,27.6,4.27239199200323));
#41139=CARTESIAN_POINT('Ctrl Pts',(-28.5855914133007,31.3,6.40858798800485));
#41140=CARTESIAN_POINT('Ctrl Pts',(-28.418924746634,35.,8.54478398400645));
#41141=CARTESIAN_POINT('Ctrl Pts',(-28.2522580799673,38.7,6.40858798800485));
#41142=CARTESIAN_POINT('Ctrl Pts',(-28.0855914133007,42.4,4.27239199200323));
#41143=CARTESIAN_POINT('Ctrl Pts',(-27.918924746634,42.4,9.06238631369041E-16));
#41144=CARTESIAN_POINT('Ctrl Pts',(-27.7522580799673,42.4,-4.27239199200323));
#41145=CARTESIAN_POINT('Ctrl Pts',(-27.5855914133007,38.7,-6.40858798800485));
#41146=CARTESIAN_POINT('Ctrl Pts',(-27.418924746634,35.,-8.54478398400645));
#41147=CARTESIAN_POINT('Ctrl Pts',(-27.2522580799673,31.3,-6.40858798800485));
#41148=CARTESIAN_POINT('Ctrl Pts',(-27.0855914133007,27.6,-4.27239199200323));
#41149=CARTESIAN_POINT('Ctrl Pts',(-26.918924746634,27.6,0.));
#41150=CARTESIAN_POINT('Ctrl Pts',(-26.7522580799673,27.6,4.27239199200323));
#41151=CARTESIAN_POINT('Ctrl Pts',(-26.5855914133007,31.3,6.40858798800485));
#41152=CARTESIAN_POINT('Ctrl Pts',(-26.418924746634,35.,8.54478398400645));
#41153=CARTESIAN_POINT('Ctrl Pts',(-26.2522580799673,38.7,6.40858798800485));
#41154=CARTESIAN_POINT('Ctrl Pts',(-26.0855914133007,42.4,4.27239199200323));
#41155=CARTESIAN_POINT('Ctrl Pts',(-25.918924746634,42.4,9.06238631369041E-16));
#41156=CARTESIAN_POINT('Ctrl Pts',(-25.7522580799673,42.4,-4.27239199200323));
#41157=CARTESIAN_POINT('Ctrl Pts',(-25.5855914133007,38.7,-6.40858798800485));
#41158=CARTESIAN_POINT('Ctrl Pts',(-25.418924746634,35.,-8.54478398400645));
#41159=CARTESIAN_POINT('Ctrl Pts',(-25.2522580799673,31.3,-6.40858798800485));
#41160=CARTESIAN_POINT('Ctrl Pts',(-25.0855914133007,27.6,-4.27239199200323));
#41161=CARTESIAN_POINT('Ctrl Pts',(-24.918924746634,27.6,0.));
#41162=CARTESIAN_POINT('Ctrl Pts',(-24.7522580799673,27.6,4.27239199200323));
#41163=CARTESIAN_POINT('Ctrl Pts',(-24.5855914133007,31.3,6.40858798800485));
#41164=CARTESIAN_POINT('Ctrl Pts',(-24.418924746634,35.,8.54478398400645));
#41165=CARTESIAN_POINT('Ctrl Pts',(-24.2522580799673,38.7,6.40858798800485));
#41166=CARTESIAN_POINT('Ctrl Pts',(-24.0855914133007,42.4,4.27239199200323));
#41167=CARTESIAN_POINT('Ctrl Pts',(-23.918924746634,42.4,9.06238631369041E-16));
#41168=CARTESIAN_POINT('Ctrl Pts',(-23.7522580799673,42.4,-4.27239199200323));
#41169=CARTESIAN_POINT('Ctrl Pts',(-23.5855914133007,38.7,-6.40858798800485));
#41170=CARTESIAN_POINT('Ctrl Pts',(-23.418924746634,35.,-8.54478398400645));
#41171=CARTESIAN_POINT('Ctrl Pts',(-23.2522580799673,31.3,-6.40858798800485));
#41172=CARTESIAN_POINT('Ctrl Pts',(-23.0855914133007,27.6,-4.27239199200323));
#41173=CARTESIAN_POINT('Ctrl Pts',(-22.918924746634,27.6,0.));
#41174=CARTESIAN_POINT('Ctrl Pts',(-22.7522580799673,27.6,4.27239199200323));
#41175=CARTESIAN_POINT('Ctrl Pts',(-22.5855914133007,31.3,6.40858798800485));
#41176=CARTESIAN_POINT('Ctrl Pts',(-22.418924746634,35.,8.54478398400645));
#41177=CARTESIAN_POINT('Ctrl Pts',(-22.2522580799673,38.7,6.40858798800485));
#41178=CARTESIAN_POINT('Ctrl Pts',(-22.0855914133007,42.4,4.27239199200323));
#41179=CARTESIAN_POINT('Ctrl Pts',(-21.918924746634,42.4,9.06238631369041E-16));
#41180=CARTESIAN_POINT('Ctrl Pts',(-21.7522580799673,42.4,-4.27239199200323));
#41181=CARTESIAN_POINT('Ctrl Pts',(-21.5855914133007,38.7,-6.40858798800485));
#41182=CARTESIAN_POINT('Ctrl Pts',(-21.418924746634,35.,-8.54478398400645));
#41183=CARTESIAN_POINT('Ctrl Pts',(-21.2522580799673,31.3,-6.40858798800485));
#41184=CARTESIAN_POINT('Ctrl Pts',(-21.0855914133007,27.6,-4.27239199200323));
#41185=CARTESIAN_POINT('Ctrl Pts',(-20.918924746634,27.6,0.));
#41186=CARTESIAN_POINT('Ctrl Pts',(-20.7522580799673,27.6,4.27239199200323));
#41187=CARTESIAN_POINT('Ctrl Pts',(-20.5855914133007,31.3,6.40858798800485));
#41188=CARTESIAN_POINT('Ctrl Pts',(-20.418924746634,35.,8.54478398400645));
#41189=CARTESIAN_POINT('Ctrl Pts',(-20.2522580799673,38.7,6.40858798800485));
#41190=CARTESIAN_POINT('Ctrl Pts',(-20.0855914133007,42.4,4.27239199200323));
#41191=CARTESIAN_POINT('Ctrl Pts',(-19.918924746634,42.4,9.06238631369041E-16));
#41192=CARTESIAN_POINT('Ctrl Pts',(-19.7522580799673,42.4,-4.27239199200323));
#41193=CARTESIAN_POINT('Ctrl Pts',(-19.5855914133007,38.7,-6.40858798800485));
#41194=CARTESIAN_POINT('Ctrl Pts',(-19.418924746634,35.,-8.54478398400645));
#41195=CARTESIAN_POINT('Ctrl Pts',(-19.2522580799673,31.3,-6.40858798800485));
#41196=CARTESIAN_POINT('Ctrl Pts',(-19.0855914133006,27.6,-4.27239199200323));
#41197=CARTESIAN_POINT('Ctrl Pts',(-18.918924746634,27.6,0.));
#41198=CARTESIAN_POINT('Ctrl Pts',(-18.7522580799673,27.6,4.27239199200323));
#41199=CARTESIAN_POINT('Ctrl Pts',(-18.5855914133007,31.3,6.40858798800485));
#41200=CARTESIAN_POINT('Ctrl Pts',(-18.418924746634,35.,8.54478398400645));
#41201=CARTESIAN_POINT('Ctrl Pts',(-18.2522580799673,38.7,6.40858798800485));
#41202=CARTESIAN_POINT('Ctrl Pts',(-18.0855914133007,42.4,4.27239199200323));
#41203=CARTESIAN_POINT('Ctrl Pts',(-17.918924746634,42.4,9.06238631369041E-16));
#41204=CARTESIAN_POINT('Ctrl Pts',(-17.7522580799673,42.4,-4.27239199200323));
#41205=CARTESIAN_POINT('Ctrl Pts',(-17.5855914133007,38.7,-6.40858798800485));
#41206=CARTESIAN_POINT('Ctrl Pts',(-17.418924746634,35.,-8.54478398400645));
#41207=CARTESIAN_POINT('Ctrl Pts',(-17.2522580799674,31.3,-6.40858798800485));
#41208=CARTESIAN_POINT('Ctrl Pts',(-17.0855914133007,27.6,-4.27239199200323));
#41209=CARTESIAN_POINT('Ctrl Pts',(-16.918924746634,27.6,0.));
#41210=CARTESIAN_POINT('Ctrl Pts',(-36.918924746634,26.,0.));
#41211=CARTESIAN_POINT('Ctrl Pts',(-36.7522580799673,26.,5.19615242270663));
#41212=CARTESIAN_POINT('Ctrl Pts',(-36.5855914133007,30.5,7.79422863405995));
#41213=CARTESIAN_POINT('Ctrl Pts',(-36.418924746634,35.,10.3923048454133));
#41214=CARTESIAN_POINT('Ctrl Pts',(-36.2522580799673,39.5,7.79422863405995));
#41215=CARTESIAN_POINT('Ctrl Pts',(-36.0855914133007,44.,5.19615242270663));
#41216=CARTESIAN_POINT('Ctrl Pts',(-35.918924746634,44.,1.10218211923262E-15));
#41217=CARTESIAN_POINT('Ctrl Pts',(-35.7522580799673,44.,-5.19615242270663));
#41218=CARTESIAN_POINT('Ctrl Pts',(-35.5855914133007,39.5,-7.79422863405995));
#41219=CARTESIAN_POINT('Ctrl Pts',(-35.418924746634,35.,-10.3923048454133));
#41220=CARTESIAN_POINT('Ctrl Pts',(-35.2522580799673,30.5,-7.79422863405995));
#41221=CARTESIAN_POINT('Ctrl Pts',(-35.0855914133007,26.,-5.19615242270663));
#41222=CARTESIAN_POINT('Ctrl Pts',(-34.918924746634,26.,0.));
#41223=CARTESIAN_POINT('Ctrl Pts',(-34.7522580799673,26.,5.19615242270663));
#41224=CARTESIAN_POINT('Ctrl Pts',(-34.5855914133007,30.5,7.79422863405995));
#41225=CARTESIAN_POINT('Ctrl Pts',(-34.418924746634,35.,10.3923048454133));
#41226=CARTESIAN_POINT('Ctrl Pts',(-34.2522580799673,39.5,7.79422863405995));
#41227=CARTESIAN_POINT('Ctrl Pts',(-34.0855914133007,44.,5.19615242270663));
#41228=CARTESIAN_POINT('Ctrl Pts',(-33.918924746634,44.,1.10218211923262E-15));
#41229=CARTESIAN_POINT('Ctrl Pts',(-33.7522580799673,44.,-5.19615242270663));
#41230=CARTESIAN_POINT('Ctrl Pts',(-33.5855914133007,39.5,-7.79422863405995));
#41231=CARTESIAN_POINT('Ctrl Pts',(-33.418924746634,35.,-10.3923048454133));
#41232=CARTESIAN_POINT('Ctrl Pts',(-33.2522580799673,30.5,-7.79422863405995));
#41233=CARTESIAN_POINT('Ctrl Pts',(-33.0855914133007,26.,-5.19615242270663));
#41234=CARTESIAN_POINT('Ctrl Pts',(-32.918924746634,26.,0.));
#41235=CARTESIAN_POINT('Ctrl Pts',(-32.7522580799673,26.,5.19615242270663));
#41236=CARTESIAN_POINT('Ctrl Pts',(-32.5855914133007,30.5,7.79422863405995));
#41237=CARTESIAN_POINT('Ctrl Pts',(-32.418924746634,35.,10.3923048454133));
#41238=CARTESIAN_POINT('Ctrl Pts',(-32.2522580799673,39.5,7.79422863405995));
#41239=CARTESIAN_POINT('Ctrl Pts',(-32.0855914133007,44.,5.19615242270663));
#41240=CARTESIAN_POINT('Ctrl Pts',(-31.918924746634,44.,1.10218211923262E-15));
#41241=CARTESIAN_POINT('Ctrl Pts',(-31.7522580799673,44.,-5.19615242270663));
#41242=CARTESIAN_POINT('Ctrl Pts',(-31.5855914133007,39.5,-7.79422863405995));
#41243=CARTESIAN_POINT('Ctrl Pts',(-31.418924746634,35.,-10.3923048454133));
#41244=CARTESIAN_POINT('Ctrl Pts',(-31.2522580799673,30.5,-7.79422863405995));
#41245=CARTESIAN_POINT('Ctrl Pts',(-31.0855914133007,26.,-5.19615242270663));
#41246=CARTESIAN_POINT('Ctrl Pts',(-30.918924746634,26.,0.));
#41247=CARTESIAN_POINT('Ctrl Pts',(-30.7522580799673,26.,5.19615242270663));
#41248=CARTESIAN_POINT('Ctrl Pts',(-30.5855914133007,30.5,7.79422863405995));
#41249=CARTESIAN_POINT('Ctrl Pts',(-30.418924746634,35.,10.3923048454133));
#41250=CARTESIAN_POINT('Ctrl Pts',(-30.2522580799673,39.5,7.79422863405995));
#41251=CARTESIAN_POINT('Ctrl Pts',(-30.0855914133007,44.,5.19615242270663));
#41252=CARTESIAN_POINT('Ctrl Pts',(-29.918924746634,44.,1.10218211923262E-15));
#41253=CARTESIAN_POINT('Ctrl Pts',(-29.7522580799673,44.,-5.19615242270663));
#41254=CARTESIAN_POINT('Ctrl Pts',(-29.5855914133007,39.5,-7.79422863405995));
#41255=CARTESIAN_POINT('Ctrl Pts',(-29.418924746634,35.,-10.3923048454133));
#41256=CARTESIAN_POINT('Ctrl Pts',(-29.2522580799673,30.5,-7.79422863405995));
#41257=CARTESIAN_POINT('Ctrl Pts',(-29.0855914133007,26.,-5.19615242270663));
#41258=CARTESIAN_POINT('Ctrl Pts',(-28.918924746634,26.,0.));
#41259=CARTESIAN_POINT('Ctrl Pts',(-28.7522580799673,26.,5.19615242270663));
#41260=CARTESIAN_POINT('Ctrl Pts',(-28.5855914133007,30.5,7.79422863405995));
#41261=CARTESIAN_POINT('Ctrl Pts',(-28.418924746634,35.,10.3923048454133));
#41262=CARTESIAN_POINT('Ctrl Pts',(-28.2522580799673,39.5,7.79422863405995));
#41263=CARTESIAN_POINT('Ctrl Pts',(-28.0855914133007,44.,5.19615242270663));
#41264=CARTESIAN_POINT('Ctrl Pts',(-27.918924746634,44.,1.10218211923262E-15));
#41265=CARTESIAN_POINT('Ctrl Pts',(-27.7522580799673,44.,-5.19615242270663));
#41266=CARTESIAN_POINT('Ctrl Pts',(-27.5855914133007,39.5,-7.79422863405995));
#41267=CARTESIAN_POINT('Ctrl Pts',(-27.418924746634,35.,-10.3923048454133));
#41268=CARTESIAN_POINT('Ctrl Pts',(-27.2522580799673,30.5,-7.79422863405995));
#41269=CARTESIAN_POINT('Ctrl Pts',(-27.0855914133007,26.,-5.19615242270663));
#41270=CARTESIAN_POINT('Ctrl Pts',(-26.918924746634,26.,0.));
#41271=CARTESIAN_POINT('Ctrl Pts',(-26.7522580799673,26.,5.19615242270663));
#41272=CARTESIAN_POINT('Ctrl Pts',(-26.5855914133007,30.5,7.79422863405995));
#41273=CARTESIAN_POINT('Ctrl Pts',(-26.418924746634,35.,10.3923048454133));
#41274=CARTESIAN_POINT('Ctrl Pts',(-26.2522580799673,39.5,7.79422863405995));
#41275=CARTESIAN_POINT('Ctrl Pts',(-26.0855914133007,44.,5.19615242270663));
#41276=CARTESIAN_POINT('Ctrl Pts',(-25.918924746634,44.,1.10218211923262E-15));
#41277=CARTESIAN_POINT('Ctrl Pts',(-25.7522580799673,44.,-5.19615242270663));
#41278=CARTESIAN_POINT('Ctrl Pts',(-25.5855914133007,39.5,-7.79422863405995));
#41279=CARTESIAN_POINT('Ctrl Pts',(-25.418924746634,35.,-10.3923048454133));
#41280=CARTESIAN_POINT('Ctrl Pts',(-25.2522580799673,30.5,-7.79422863405995));
#41281=CARTESIAN_POINT('Ctrl Pts',(-25.0855914133007,26.,-5.19615242270663));
#41282=CARTESIAN_POINT('Ctrl Pts',(-24.918924746634,26.,0.));
#41283=CARTESIAN_POINT('Ctrl Pts',(-24.7522580799673,26.,5.19615242270663));
#41284=CARTESIAN_POINT('Ctrl Pts',(-24.5855914133007,30.5,7.79422863405995));
#41285=CARTESIAN_POINT('Ctrl Pts',(-24.418924746634,35.,10.3923048454133));
#41286=CARTESIAN_POINT('Ctrl Pts',(-24.2522580799673,39.5,7.79422863405995));
#41287=CARTESIAN_POINT('Ctrl Pts',(-24.0855914133007,44.,5.19615242270663));
#41288=CARTESIAN_POINT('Ctrl Pts',(-23.918924746634,44.,1.10218211923262E-15));
#41289=CARTESIAN_POINT('Ctrl Pts',(-23.7522580799673,44.,-5.19615242270663));
#41290=CARTESIAN_POINT('Ctrl Pts',(-23.5855914133007,39.5,-7.79422863405995));
#41291=CARTESIAN_POINT('Ctrl Pts',(-23.418924746634,35.,-10.3923048454133));
#41292=CARTESIAN_POINT('Ctrl Pts',(-23.2522580799673,30.5,-7.79422863405995));
#41293=CARTESIAN_POINT('Ctrl Pts',(-23.0855914133007,26.,-5.19615242270663));
#41294=CARTESIAN_POINT('Ctrl Pts',(-22.918924746634,26.,0.));
#41295=CARTESIAN_POINT('Ctrl Pts',(-22.7522580799673,26.,5.19615242270663));
#41296=CARTESIAN_POINT('Ctrl Pts',(-22.5855914133007,30.5,7.79422863405995));
#41297=CARTESIAN_POINT('Ctrl Pts',(-22.418924746634,35.,10.3923048454133));
#41298=CARTESIAN_POINT('Ctrl Pts',(-22.2522580799674,39.5,7.79422863405995));
#41299=CARTESIAN_POINT('Ctrl Pts',(-22.0855914133007,44.,5.19615242270663));
#41300=CARTESIAN_POINT('Ctrl Pts',(-21.918924746634,44.,1.10218211923262E-15));
#41301=CARTESIAN_POINT('Ctrl Pts',(-21.7522580799673,44.,-5.19615242270663));
#41302=CARTESIAN_POINT('Ctrl Pts',(-21.5855914133006,39.5,-7.79422863405995));
#41303=CARTESIAN_POINT('Ctrl Pts',(-21.418924746634,35.,-10.3923048454133));
#41304=CARTESIAN_POINT('Ctrl Pts',(-21.2522580799673,30.5,-7.79422863405995));
#41305=CARTESIAN_POINT('Ctrl Pts',(-21.0855914133007,26.,-5.19615242270663));
#41306=CARTESIAN_POINT('Ctrl Pts',(-20.918924746634,26.,0.));
#41307=CARTESIAN_POINT('Ctrl Pts',(-20.7522580799673,26.,5.19615242270663));
#41308=CARTESIAN_POINT('Ctrl Pts',(-20.5855914133006,30.5,7.79422863405995));
#41309=CARTESIAN_POINT('Ctrl Pts',(-20.418924746634,35.,10.3923048454133));
#41310=CARTESIAN_POINT('Ctrl Pts',(-20.2522580799673,39.5,7.79422863405995));
#41311=CARTESIAN_POINT('Ctrl Pts',(-20.0855914133007,44.,5.19615242270663));
#41312=CARTESIAN_POINT('Ctrl Pts',(-19.918924746634,44.,1.10218211923262E-15));
#41313=CARTESIAN_POINT('Ctrl Pts',(-19.7522580799674,44.,-5.19615242270663));
#41314=CARTESIAN_POINT('Ctrl Pts',(-19.5855914133006,39.5,-7.79422863405995));
#41315=CARTESIAN_POINT('Ctrl Pts',(-19.418924746634,35.,-10.3923048454133));
#41316=CARTESIAN_POINT('Ctrl Pts',(-19.2522580799674,30.5,-7.79422863405995));
#41317=CARTESIAN_POINT('Ctrl Pts',(-19.0855914133007,26.,-5.19615242270663));
#41318=CARTESIAN_POINT('Ctrl Pts',(-18.918924746634,26.,0.));
#41319=CARTESIAN_POINT('Ctrl Pts',(-18.7522580799673,26.,5.19615242270663));
#41320=CARTESIAN_POINT('Ctrl Pts',(-18.5855914133006,30.5,7.79422863405995));
#41321=CARTESIAN_POINT('Ctrl Pts',(-18.418924746634,35.,10.3923048454133));
#41322=CARTESIAN_POINT('Ctrl Pts',(-18.2522580799673,39.5,7.79422863405995));
#41323=CARTESIAN_POINT('Ctrl Pts',(-18.0855914133006,44.,5.19615242270663));
#41324=CARTESIAN_POINT('Ctrl Pts',(-17.918924746634,44.,1.10218211923262E-15));
#41325=CARTESIAN_POINT('Ctrl Pts',(-17.7522580799673,44.,-5.19615242270663));
#41326=CARTESIAN_POINT('Ctrl Pts',(-17.5855914133006,39.5,-7.79422863405995));
#41327=CARTESIAN_POINT('Ctrl Pts',(-17.418924746634,35.,-10.3923048454133));
#41328=CARTESIAN_POINT('Ctrl Pts',(-17.2522580799673,30.5,-7.79422863405995));
#41329=CARTESIAN_POINT('Ctrl Pts',(-17.0855914133007,26.,-5.19615242270663));
#41330=CARTESIAN_POINT('Ctrl Pts',(-16.918924746634,26.,0.));
#41331=CARTESIAN_POINT('Origin',(-42.,34.999999994595,6.55E-10));
#41332=CARTESIAN_POINT('',(-42.,38.0494565603535,5.1672831023974));
#41333=CARTESIAN_POINT('',(-42.,40.65404535889,-2.00792704445741));
#41334=CARTESIAN_POINT('Origin',(-46.,44.2399040040528,-4.98740151676925));
#41335=CARTESIAN_POINT('',(-42.5,40.1413699032525,-3.09294608072936));
#41336=CARTESIAN_POINT('',(-42.5,40.1413699032525,-3.09294608072936));
#41337=CARTESIAN_POINT('',(-45.5,40.1413699032525,-3.09294608072936));
#41338=CARTESIAN_POINT('',(-42.,40.1413699032525,-3.09294608072936));
#41339=CARTESIAN_POINT('',(-45.5,44.2399040040528,-4.98740151676925));
#41340=CARTESIAN_POINT('Origin',(-46.,44.7486243140984,-3.90055430318255));
#41341=CARTESIAN_POINT('',(-42.5,44.7486243140985,-3.90055430318256));
#41342=CARTESIAN_POINT('',(-46.,44.7486243140984,-3.90055430318255));
#41343=CARTESIAN_POINT('',(-45.5,44.7486243140984,-3.90055430318255));
#41344=CARTESIAN_POINT('Origin',(-46.,35.7752519450148,0.24718575365908));
#41345=CARTESIAN_POINT('',(-46.,39.9429588225849,9.26375507215795));
#41346=CARTESIAN_POINT('',(-42.5,38.0494565603535,5.1672831023974));
#41347=CARTESIAN_POINT('',(-45.5,35.7752519450148,0.24718575365908));
#41348=CARTESIAN_POINT('Origin',(-46.,34.6859864596583,0.750674286210626));
#41349=CARTESIAN_POINT('',(-45.5,36.9601910749969,5.67077163494895));
#41350=CARTESIAN_POINT('',(-42.5,36.9601910749969,5.67077163494895));
#41351=CARTESIAN_POINT('',(-42.,36.9601910749969,5.67077163494895));
#41352=CARTESIAN_POINT('',(-42.5,38.8536933372283,9.7672436047095));
#41353=CARTESIAN_POINT('',(-42.5,38.8536933372283,9.7672436047095));
#41354=CARTESIAN_POINT('',(-45.5,38.8536933372283,9.7672436047095));
#41355=CARTESIAN_POINT('',(-46.,38.8536933372283,9.7672436047095));
#41356=CARTESIAN_POINT('',(-45.5,34.6859864596583,0.750674286210626));
#41357=CARTESIAN_POINT('Origin',(-46.,32.151915435741,0.600000000655));
#41358=CARTESIAN_POINT('',(-45.5,29.3128914363174,1.91227514988591));
#41359=CARTESIAN_POINT('',(-42.5,29.3128914363174,1.91227514988591));
#41360=CARTESIAN_POINT('',(-42.,29.3128914363174,1.91227514988591));
#41361=CARTESIAN_POINT('',(-42.5,25.2143573355172,3.80673058592581));
#41362=CARTESIAN_POINT('',(-42.5,25.6691348322782,3.59651989114122));
#41363=CARTESIAN_POINT('',(-45.5,25.2143573355172,3.80673058592581));
#41364=CARTESIAN_POINT('',(-46.,25.2143573355172,3.80673058592581));
#41365=CARTESIAN_POINT('',(-45.5,32.151915435741,0.600000000655));
#41366=CARTESIAN_POINT('Origin',(-46.,34.6859864596583,0.750674286210626));
#41367=CARTESIAN_POINT('',(-45.5,25.7126140905746,4.89841434305227));
#41368=CARTESIAN_POINT('',(-42.5,25.7126140905746,4.89841434305227));
#41369=CARTESIAN_POINT('',(-46.,25.7126140905746,4.89841434305227));
#41370=CARTESIAN_POINT('',(-42.5,29.807193045783,3.00578708432712));
#41371=CARTESIAN_POINT('',(-42.5,29.807193045783,3.00578708432712));
#41372=CARTESIAN_POINT('',(-45.5,29.807193045783,3.00578708432712));
#41373=CARTESIAN_POINT('',(-42.,29.807193045783,3.00578708432712));
#41374=CARTESIAN_POINT('',(-45.5,34.6859864596583,0.750674286210626));
#41375=CARTESIAN_POINT('Origin',(-34.5,20.2255401693197,-2.54750793782168));
#41376=CARTESIAN_POINT('',(-38.5,20.2255401693197,-0.0980181950384988));
#41377=CARTESIAN_POINT('Origin',(-45.5,35.0208323137734,0.0450694010362789));
#41378=CARTESIAN_POINT('',(-46.,35.0208323137734,0.0450694010362797));
#41379=CARTESIAN_POINT('Origin',(-45.5,35.0907721183747,-0.0419573770576284));
#41380=CARTESIAN_POINT('',(-46.,35.0907721183747,-0.0419573770576286));
#41381=CARTESIAN_POINT('Origin',(-45.5,34.999999994595,6.55E-10));
#41382=CARTESIAN_POINT('',(-46.,25.0360004143143,4.66033393334341));
#41383=CARTESIAN_POINT('Ctrl Pts',(-46.,25.0360004143144,4.66033393334341));
#41384=CARTESIAN_POINT('Ctrl Pts',(-46.,25.0374024690213,4.66084598634663));
#41385=CARTESIAN_POINT('Ctrl Pts',(-45.9999966731511,25.0388045641603,4.66135793950374));
#41386=CARTESIAN_POINT('Ctrl Pts',(-45.9996492133389,25.1120391418205,4.68809241397306));
#41387=CARTESIAN_POINT('Ctrl Pts',(-45.9905781028549,25.1844197231217,4.7142058989083));
#41388=CARTESIAN_POINT('Ctrl Pts',(-45.9554702797948,25.3212199515064,4.76299808794914));
#41389=CARTESIAN_POINT('Ctrl Pts',(-45.929938447608,25.386863762187,4.78613722556436));
#41390=CARTESIAN_POINT('Ctrl Pts',(-45.8613791715261,25.5071706542225,4.82812523107859));
#41391=CARTESIAN_POINT('Ctrl Pts',(-45.8179795164162,25.5630011722499,4.84738471823477));
#41392=CARTESIAN_POINT('Ctrl Pts',(-45.7258076109511,25.6418150671328,4.87438209952366));
#41393=CARTESIAN_POINT('Ctrl Pts',(-45.6815277725054,25.6694803280007,4.88379024826762));
#41394=CARTESIAN_POINT('Ctrl Pts',(-45.5903579073579,25.7039748155375,4.89549515091947));
#41395=CARTESIAN_POINT('Ctrl Pts',(-45.5458624658048,25.712577506522,4.89840196573932));
#41396=CARTESIAN_POINT('Ctrl Pts',(-45.5001938310099,25.7126140518,4.8984143299332));
#41397=CARTESIAN_POINT('Ctrl Pts',(-45.5000969130038,25.7126140905746,4.89841434305228));
#41398=CARTESIAN_POINT('Ctrl Pts',(-45.5,25.7126140905746,4.89841434305228));
#41399=CARTESIAN_POINT('',(-46.,39.5243486999107,10.0264783850484));
#41400=CARTESIAN_POINT('Origin',(-46.,34.999999994595,6.55E-10));
#41401=CARTESIAN_POINT('Ctrl Pts',(-45.5,38.8536933372283,9.76724360470951));
#41402=CARTESIAN_POINT('Ctrl Pts',(-45.5475202328384,38.8536933372283,9.76724360470951));
#41403=CARTESIAN_POINT('Ctrl Pts',(-45.5938300790285,38.8628412828318,9.77091254431395));
#41404=CARTESIAN_POINT('Ctrl Pts',(-45.6926831164288,38.9011133206408,9.78620047778414));
#41405=CARTESIAN_POINT('Ctrl Pts',(-45.7416688429774,38.9337902963357,9.79922369582153));
#41406=CARTESIAN_POINT('Ctrl Pts',(-45.8419265836025,39.0270141336349,9.83609034985595));
#41407=CARTESIAN_POINT('Ctrl Pts',(-45.8908401903905,39.0968099336531,9.86350378153489));
#41408=CARTESIAN_POINT('Ctrl Pts',(-45.9741804024576,39.2809978199734,9.93476534492679));
#41409=CARTESIAN_POINT('Ctrl Pts',(-45.999416722443,39.399345156675,9.9798386246279));
#41410=CARTESIAN_POINT('Ctrl Pts',(-45.9999966732101,39.5215452282668,10.0254327281341));
#41411=CARTESIAN_POINT('Ctrl Pts',(-46.,39.5229469469093,10.0259556080299));
#41412=CARTESIAN_POINT('Ctrl Pts',(-46.,39.5243486999107,10.0264783850484));
#41413=CARTESIAN_POINT('Origin',(-45.5,34.999999994595,6.55E-10));
#41414=CARTESIAN_POINT('Origin',(-45.5,34.9092278708153,0.0419573783676288));
#41415=CARTESIAN_POINT('',(-46.,37.216502182775,5.03359891691694));
#41416=CARTESIAN_POINT('',(-46.,34.9092278708153,0.0419573783676291));
#41417=CARTESIAN_POINT('Ctrl Pts',(-45.5,36.9601910749969,5.67077163494895));
#41418=CARTESIAN_POINT('Ctrl Pts',(-45.548970157778,36.9601910749969,5.67077163494895));
#41419=CARTESIAN_POINT('Ctrl Pts',(-45.5969081567834,36.9639934004896,5.66185790620149));
#41420=CARTESIAN_POINT('Ctrl Pts',(-45.6935221969332,36.9791200174418,5.62617368236302));
#41421=CARTESIAN_POINT('Ctrl Pts',(-45.7398209612911,36.9910294096094,5.59799230724864));
#41422=CARTESIAN_POINT('Ctrl Pts',(-45.8328892935188,37.0240200249968,5.51906769418711));
#41423=CARTESIAN_POINT('Ctrl Pts',(-45.8753161788561,37.0465011132908,5.46473906324288));
#41424=CARTESIAN_POINT('Ctrl Pts',(-45.9385897729845,37.0925851272751,5.35135036405417));
#41425=CARTESIAN_POINT('Ctrl Pts',(-45.9609910872761,37.1161401001897,5.29255243634324));
#41426=CARTESIAN_POINT('Ctrl Pts',(-45.9918589780635,37.164790965817,5.16888552792546));
#41427=CARTESIAN_POINT('Ctrl Pts',(-45.9996751413526,37.1901469176321,5.10324005942292));
#41428=CARTESIAN_POINT('Ctrl Pts',(-45.9999966939211,37.2154612250376,5.03635122598603));
#41429=CARTESIAN_POINT('Ctrl Pts',(-46.,37.2159818012366,5.03497510643485));
#41430=CARTESIAN_POINT('Ctrl Pts',(-46.,37.2165021827753,5.03359891691704));
#41431=CARTESIAN_POINT('Origin',(-45.5,35.0208323137734,0.0450694010362796));
#41432=CARTESIAN_POINT('',(-46.,30.0285689416169,2.35263114162986));
#41433=CARTESIAN_POINT('Ctrl Pts',(-46.,30.0285689416169,2.35263114162986));
#41434=CARTESIAN_POINT('Ctrl Pts',(-46.,30.0280650993038,2.3540204371795));
#41435=CARTESIAN_POINT('Ctrl Pts',(-45.9999966944273,30.0275614528911,2.35540980745037));
#41436=CARTESIAN_POINT('Ctrl Pts',(-45.9996738586582,30.0029878258742,2.42322916399792));
#41437=CARTESIAN_POINT('Ctrl Pts',(-45.9917939389854,29.979263333268,2.49014276072554));
#41438=CARTESIAN_POINT('Ctrl Pts',(-45.9606603025493,29.9352867624643,2.61669625614254));
#41439=CARTESIAN_POINT('Ctrl Pts',(-45.938073114642,29.914713691535,2.67712605416832));
#41440=CARTESIAN_POINT('Ctrl Pts',(-45.8744779446781,29.8757270841149,2.79357023434024));
#41441=CARTESIAN_POINT('Ctrl Pts',(-45.8320302750286,29.8574143381371,2.84943977548591));
#41442=CARTESIAN_POINT('Ctrl Pts',(-45.7390416503862,29.8311027950442,2.93069950697313));
#41443=CARTESIAN_POINT('Ctrl Pts',(-45.6928616793168,29.8218160767511,2.95976786559309));
#41444=CARTESIAN_POINT('Ctrl Pts',(-45.5965455901766,29.8101006897299,2.9965789582576));
#41445=CARTESIAN_POINT('Ctrl Pts',(-45.5487893624249,29.807193045783,3.00578708432712));
#41446=CARTESIAN_POINT('Ctrl Pts',(-45.5,29.807193045783,3.00578708432712));
#41447=CARTESIAN_POINT('',(-46.,35.0208323137734,0.0450694010362801));
#41448=CARTESIAN_POINT('Origin',(-42.5,44.9584112026616,-3.44669368428398));
#41449=CARTESIAN_POINT('',(-42.,40.8638322474532,-1.55406642555884));
#41450=CARTESIAN_POINT('Origin',(-42.5,36.2291125639134,0.0373988650959357));
#41451=CARTESIAN_POINT('',(-42.,40.3968194414835,9.05396818359482));
#41452=CARTESIAN_POINT('Origin',(-42.5,34.999999994595,6.55E-10));
#41453=CARTESIAN_POINT('',(-42.,28.7102900092541,1.63998423847662));
#41454=CARTESIAN_POINT('Ctrl Pts',(-42.,28.7102900092541,1.63998423847662));
#41455=CARTESIAN_POINT('Ctrl Pts',(-42.,28.7115300500983,1.64057011650148));
#41456=CARTESIAN_POINT('Ctrl Pts',(-42.0000033207593,28.7127701523771,1.64115586956709));
#41457=CARTESIAN_POINT('Ctrl Pts',(-42.0004541950922,28.796981233661,1.68092188321178));
#41458=CARTESIAN_POINT('Ctrl Pts',(-42.0157573105942,28.8807676884173,1.71976480349444));
#41459=CARTESIAN_POINT('Ctrl Pts',(-42.0728019198682,29.0291511352119,1.78736590420412));
#41460=CARTESIAN_POINT('Ctrl Pts',(-42.1117195110958,29.0957873621205,1.81719592643935));
#41461=CARTESIAN_POINT('Ctrl Pts',(-42.2018967293794,29.195960411313,1.86148481105511));
#41462=CARTESIAN_POINT('Ctrl Pts',(-42.2479008339596,29.2336465552485,1.87794439145772));
#41463=CARTESIAN_POINT('Ctrl Pts',(-42.3442168820676,29.2851395596278,1.90031310744936));
#41464=CARTESIAN_POINT('Ctrl Pts',(-42.3916288820851,29.3014155492391,1.90732915008605));
#41465=CARTESIAN_POINT('Ctrl Pts',(-42.4610040616797,29.3114870702353,1.91167044475591));
#41466=CARTESIAN_POINT('Ctrl Pts',(-42.4805205119926,29.3128914363174,1.91227514988591));
#41467=CARTESIAN_POINT('Ctrl Pts',(-42.5,29.3128914363174,1.91227514988591));
#41468=CARTESIAN_POINT('',(-42.5,29.0300753719553,0.600000000655));
#41469=CARTESIAN_POINT('Origin',(-42.5,34.999999994595,6.55E-10));
#41470=CARTESIAN_POINT('',(-42.,28.5937530433762,1.100000000655));
#41471=CARTESIAN_POINT('Ctrl Pts',(-42.,28.5937530433762,1.100000000655));
#41472=CARTESIAN_POINT('Ctrl Pts',(-42.,28.5946398535677,1.09894794045397));
#41473=CARTESIAN_POINT('Ctrl Pts',(-42.0000033204919,28.5955267728317,1.0978959693116));
#41474=CARTESIAN_POINT('Ctrl Pts',(-42.0004662363704,28.6573726864835,1.02455603604737));
#41475=CARTESIAN_POINT('Ctrl Pts',(-42.0165992209748,28.7192952337357,0.952209618319868));
#41476=CARTESIAN_POINT('Ctrl Pts',(-42.0758441660175,28.8273260851525,0.82772417571545));
#41477=CARTESIAN_POINT('Ctrl Pts',(-42.1151456113167,28.8751198610887,0.773377665751314));
#41478=CARTESIAN_POINT('Ctrl Pts',(-42.2056695167071,28.9469442910977,0.692456560469139));
#41479=CARTESIAN_POINT('Ctrl Pts',(-42.2516602512676,28.9739516189116,0.662301438777017));
#41480=CARTESIAN_POINT('Ctrl Pts',(-42.34779518891,29.0107522579474,0.621371214703135));
#41481=CARTESIAN_POINT('Ctrl Pts',(-42.3950686181707,29.0223139734333,0.608583817890182));
#41482=CARTESIAN_POINT('Ctrl Pts',(-42.4631644468274,29.029156829769,0.601015248913021));
#41483=CARTESIAN_POINT('Ctrl Pts',(-42.4816022135789,29.0300753719553,0.600000000655));
#41484=CARTESIAN_POINT('Ctrl Pts',(-42.5,29.0300753719553,0.600000000655));
#41485=CARTESIAN_POINT('Origin',(-42.,34.999999994595,6.55E-10));
#41486=CARTESIAN_POINT('Origin',(-41.5,25.2185048259584,-6.04750793782168));
#41487=CARTESIAN_POINT('',(-41.5,25.2185048259584,-5.04750793782168));
#41488=CARTESIAN_POINT('',(-42.,25.2185048259584,-4.54750793782168));
#41489=CARTESIAN_POINT('Origin',(-41.5,25.2185048259584,-4.54750793782167));
#41490=CARTESIAN_POINT('',(-42.,26.4943520218675,-5.25870255454211));
#41491=CARTESIAN_POINT('Origin',(-42.,25.2185048259584,-6.04750793782168));
#41492=CARTESIAN_POINT('',(-41.5,26.0690696232311,-5.52163768230196));
#41493=CARTESIAN_POINT('Origin',(-41.5,26.4943520218675,-5.25870255454211));
#41494=CARTESIAN_POINT('Origin',(-41.5,25.2185048259584,-6.04750793782168));
#41495=CARTESIAN_POINT('Origin',(-41.5,34.999999994595,-4.54750793782168));
#41496=CARTESIAN_POINT('',(-42.,34.999999994595,-4.54750793782168));
#41497=CARTESIAN_POINT('',(-41.5,20.7255401693197,-5.04750793782167));
#41498=CARTESIAN_POINT('Origin',(-40.,34.999999994595,6.55E-10));
#41499=CARTESIAN_POINT('',(-40.,52.6486129734088,-3.5392739254555));
#41500=CARTESIAN_POINT('',(-40.,52.9941026808875,0.460726074544506));
#41501=CARTESIAN_POINT('Origin',(-40.,34.999999994595,6.54998265276524E-10));
#41502=CARTESIAN_POINT('',(-40.,56.5946168001448,0.460726074544506));
#41503=CARTESIAN_POINT('',(-40.,56.5946168001448,0.460726074544506));
#41504=CARTESIAN_POINT('',(-40.,56.5946168001448,-3.5392739254555));
#41505=CARTESIAN_POINT('',(-40.,56.5946168001448,-3.5392739254555));
#41506=CARTESIAN_POINT('',(-40.,48.5946168001447,-3.5392739254555));
#41507=CARTESIAN_POINT('Ctrl Pts',(-38.8535045584117,49.0947070026403,3.3142306281657));
#41508=CARTESIAN_POINT('Ctrl Pts',(-39.,49.09474437335,3.46068560589431));
#41509=CARTESIAN_POINT('Ctrl Pts',(-39.,49.0947972300504,3.66783283265958));
#41510=CARTESIAN_POINT('Ctrl Pts',(-38.8535080713606,49.067246177754,3.31424116296626));
#41511=CARTESIAN_POINT('Ctrl Pts',(-38.9999999999999,49.0559066742947,3.46069849069773));
#41512=CARTESIAN_POINT('Ctrl Pts',(-39.,49.0398679954685,3.66784688025153));
#41513=CARTESIAN_POINT('Ctrl Pts',(-38.8519073632856,49.0397855966119,3.30944090472416));
#41514=CARTESIAN_POINT('Ctrl Pts',(-39.,49.0169980247426,3.45482188858408));
#41515=CARTESIAN_POINT('Ctrl Pts',(-39.,48.9849392151471,3.66144599708733));
#41516=CARTESIAN_POINT('Ctrl Pts',(-38.8455443417981,48.9856360525285,3.29035917900804));
#41517=CARTESIAN_POINT('Ctrl Pts',(-39.,48.9409553642149,3.43158518892926));
#41518=CARTESIAN_POINT('Ctrl Pts',(-39.,48.8766256560199,3.63600161677062));
#41519=CARTESIAN_POINT('Ctrl Pts',(-38.8407855746403,48.9589470995131,3.27608834575365));
#41520=CARTESIAN_POINT('Ctrl Pts',(-39.,48.9036879387245,3.4141524411812));
#41521=CARTESIAN_POINT('Ctrl Pts',(-39.,48.8232408334419,3.61697226872685));
#41522=CARTESIAN_POINT('Ctrl Pts',(-38.8282385003299,48.9070311494151,3.23846128171868));
#41523=CARTESIAN_POINT('Ctrl Pts',(-39.,48.8324120146563,3.36848126327577));
#41524=CARTESIAN_POINT('Ctrl Pts',(-39.,48.7193964919575,3.56679887235799));
#41525=CARTESIAN_POINT('Ctrl Pts',(-38.8204503561327,48.8818047904229,3.21510553874763));
#41526=CARTESIAN_POINT('Ctrl Pts',(-39.,48.798299096021,3.34007866638608));
#41527=CARTESIAN_POINT('Ctrl Pts',(-39.,48.6689381953401,3.53565541494599));
#41528=CARTESIAN_POINT('Ctrl Pts',(-38.8020550847506,48.8334958478087,3.15993971871678));
#41529=CARTESIAN_POINT('Ctrl Pts',(-39.,48.7347624479236,3.27350216862877));
#41530=CARTESIAN_POINT('Ctrl Pts',(-39.,48.5723110828561,3.46209545845528));
#41531=CARTESIAN_POINT('Ctrl Pts',(-38.7914481963086,48.8104138547599,3.12813035637803));
#41532=CARTESIAN_POINT('Ctrl Pts',(-39.,48.7052783560689,3.2350973112));
#41533=CARTESIAN_POINT('Ctrl Pts',(-39.,48.5261434083848,3.41967982872211));
#41534=CARTESIAN_POINT('Ctrl Pts',(-38.7677022294448,48.7670175509742,3.05691688025654));
#41535=CARTESIAN_POINT('Ctrl Pts',(-39.,48.6522917384422,3.14989967862306));
#41536=CARTESIAN_POINT('Ctrl Pts',(-39.,48.4393457551925,3.32472194096288));
#41537=CARTESIAN_POINT('Ctrl Pts',(-38.754563458535,48.7467037654173,3.01751368713769));
#41538=CARTESIAN_POINT('Ctrl Pts',(-39.,48.6287878978116,3.10282744096632));
#41539=CARTESIAN_POINT('Ctrl Pts',(-39.,48.3987168054773,3.2721808091293));
#41540=CARTESIAN_POINT('Ctrl Pts',(-38.7261089954399,48.7093930151617,2.93217742113975));
#41541=CARTESIAN_POINT('Ctrl Pts',(-39.,48.5888782841862,3.00200407984343));
#41542=CARTESIAN_POINT('Ctrl Pts',(-39.,48.3240951111972,3.15839209372811));
#41543=CARTESIAN_POINT('Ctrl Pts',(-38.7107936702028,48.6923964942063,2.88624544697246));
#41544=CARTESIAN_POINT('Ctrl Pts',(-39.,48.5725424429904,2.94794928112244));
#41545=CARTESIAN_POINT('Ctrl Pts',(-39.,48.2901032541095,3.09714586388256));
#41546=CARTESIAN_POINT('Ctrl Pts',(-38.6784002298215,48.6621798063133,2.78909300074232));
#41547=CARTESIAN_POINT('Ctrl Pts',(-39.,48.5478707626514,2.83517053538946));
#41548=CARTESIAN_POINT('Ctrl Pts',(-39.,48.2296748519216,2.96760249981115));
#41549=CARTESIAN_POINT('Ctrl Pts',(-38.6613225297323,48.6489599882654,2.73787377156343));
#41550=CARTESIAN_POINT('Ctrl Pts',(-39.,48.5396844114206,2.77614897370115));
#41551=CARTESIAN_POINT('Ctrl Pts',(-39.,48.2032390273215,2.89930691056257));
#41552=CARTESIAN_POINT('Ctrl Pts',(-38.6258661281208,48.6266542170724,2.63153115721682));
#41553=CARTESIAN_POINT('Ctrl Pts',(-39.0000000000001,48.5319565439657,2.65572283557889));
#41554=CARTESIAN_POINT('Ctrl Pts',(-39.,48.1586375470106,2.75751099023676));
#41555=CARTESIAN_POINT('Ctrl Pts',(-38.6074878768702,48.6175685077662,2.57640912054356));
#41556=CARTESIAN_POINT('Ctrl Pts',(-39.,48.5326470103469,2.59406293637931));
#41557=CARTESIAN_POINT('Ctrl Pts',(-39.,48.140472424078,2.68401235333488));
#41558=CARTESIAN_POINT('Ctrl Pts',(-38.5699273237463,48.60377678196,2.46375077843951));
#41559=CARTESIAN_POINT('Ctrl Pts',(-39.,48.543008106918,2.47090089780404));
#41560=CARTESIAN_POINT('Ctrl Pts',(-39.,48.1129036282315,2.53379720651331));
#41561=CARTESIAN_POINT('Ctrl Pts',(-38.5507454934032,48.5990708976697,2.40621588532438));
#41562=CARTESIAN_POINT('Ctrl Pts',(-38.9999999999999,48.5529886102347,2.40922780847103));
#41563=CARTESIAN_POINT('Ctrl Pts',(-39.,48.1035002850315,2.4570824934803));
#41564=CARTESIAN_POINT('Ctrl Pts',(-38.5120964494218,48.5941663241322,2.29028699517654));
#41565=CARTESIAN_POINT('Ctrl Pts',(-39.0000000000001,48.5818825838363,2.28881570408228));
#41566=CARTESIAN_POINT('Ctrl Pts',(-39.,48.0937094722848,2.30250905646815));
#41567=CARTESIAN_POINT('Ctrl Pts',(-38.49262971406,48.5939676527499,2.23189443078616));
#41568=CARTESIAN_POINT('Ctrl Pts',(-38.9999999999999,48.6011682984858,2.23003752380745));
#41569=CARTESIAN_POINT('Ctrl Pts',(-39.,48.0933221199033,2.22465218259804));
#41570=CARTESIAN_POINT('Ctrl Pts',(-38.4539372108061,48.5980832374213,2.11582860920987));
#41571=CARTESIAN_POINT('Ctrl Pts',(-39.0000000000001,48.6481312853257,2.11840511180508));
#41572=CARTESIAN_POINT('Ctrl Pts',(-39.,48.1015739764395,2.06989921432186));
#41573=CARTESIAN_POINT('Ctrl Pts',(-38.4347119133934,48.6023973982706,2.05815676133583));
#41574=CARTESIAN_POINT('Ctrl Pts',(-38.9999999999999,48.6762114086241,2.06569441899641));
#41575=CARTESIAN_POINT('Ctrl Pts',(-39.,48.1102130866064,1.99300497221786));
#41576=CARTESIAN_POINT('Ctrl Pts',(-38.3970220794501,48.6154224582525,1.94509137355602));
#41577=CARTESIAN_POINT('Ctrl Pts',(-39.0000000000001,48.7395494710663,1.9693555563745));
#41578=CARTESIAN_POINT('Ctrl Pts',(-39.,48.1362845305971,1.84225608507716));
#41579=CARTESIAN_POINT('Ctrl Pts',(-38.3785579915537,48.6241331544289,1.88969917736693));
#41580=CARTESIAN_POINT('Ctrl Pts',(-38.9999999999999,48.7751847398666,1.92610272382598));
#41581=CARTESIAN_POINT('Ctrl Pts',(-39.,48.153716552592,1.76840324344311));
#41582=CARTESIAN_POINT('Ctrl Pts',(-38.3518067382149,48.6403205713055,1.80944249844404));
#41583=CARTESIAN_POINT('Ctrl Pts',(-39.,48.8316806212018,1.87113650918206));
#41584=CARTESIAN_POINT('Ctrl Pts',(-39.,48.1861062119123,1.66140116307555));
#41585=CARTESIAN_POINT('Ctrl Pts',(-38.3430469593461,48.6462356653694,1.78316168828865));
#41586=CARTESIAN_POINT('Ctrl Pts',(-39.,48.8514141523639,1.85423124984201));
#41587=CARTESIAN_POINT('Ctrl Pts',(-39.,48.1979412146227,1.62636250356297));
#41588=CARTESIAN_POINT('Ctrl Pts',(-38.3259012464104,48.6590644974859,1.73172063147388));
#41589=CARTESIAN_POINT('Ctrl Pts',(-39.,48.8917573484389,1.82394074538817));
#41590=CARTESIAN_POINT('Ctrl Pts',(-39.,48.2236080194775,1.55777972874027));
#41591=CARTESIAN_POINT('Ctrl Pts',(-38.3175153184177,48.6659782242293,1.70656040296349));
#41592=CARTESIAN_POINT('Ctrl Pts',(-39.,48.912387085206,1.81065038969406));
#41593=CARTESIAN_POINT('Ctrl Pts',(-39.,48.2374398092193,1.52423564661872));
#41594=CARTESIAN_POINT('Ctrl Pts',(-38.3011740677622,48.6807575825497,1.6575308483829));
#41595=CARTESIAN_POINT('Ctrl Pts',(-39.,48.9540184168853,1.78795051379182));
#41596=CARTESIAN_POINT('Ctrl Pts',(-39.,48.2670065486315,1.45886912201177));
#41597=CARTESIAN_POINT('Ctrl Pts',(-38.2932187499813,48.6886232026976,1.63366153687808));
#41598=CARTESIAN_POINT('Ctrl Pts',(-39.,48.9750223828953,1.7786505831365));
#41599=CARTESIAN_POINT('Ctrl Pts',(-39.,48.2827414843619,1.4270467103952));
#41600=CARTESIAN_POINT('Ctrl Pts',(-38.2777925604244,48.7052531688598,1.5873754255043));
#41601=CARTESIAN_POINT('Ctrl Pts',(-39.,49.0167801391035,1.76422804457118));
#41602=CARTESIAN_POINT('Ctrl Pts',(-39.,48.3160079917187,1.3653389668037));
#41603=CARTESIAN_POINT('Ctrl Pts',(-38.2703216923166,48.7140175036481,1.56495863655659));
#41604=CARTESIAN_POINT('Ctrl Pts',(-39.,49.0375135780982,1.75922619646151));
#41605=CARTESIAN_POINT('Ctrl Pts',(-39.,48.3335395481203,1.33545366312211));
#41606=CARTESIAN_POINT('Ctrl Pts',(-38.255914958235,48.7323856389745,1.52172935831263));
#41607=CARTESIAN_POINT('Ctrl Pts',(-39.,49.0779804973326,1.75359046880955));
#41608=CARTESIAN_POINT('Ctrl Pts',(-39.,48.370280609407,1.27782246142017));
#41609=CARTESIAN_POINT('Ctrl Pts',(-38.2489790947276,48.741989428833,1.50091687634094));
#41610=CARTESIAN_POINT('Ctrl Pts',(-39.,49.0976661851908,1.75308248268751));
#41611=CARTESIAN_POINT('Ctrl Pts',(-39.,48.3894900980617,1.25007658891254));
#41612=CARTESIAN_POINT('Ctrl Pts',(-38.2356892991005,48.7619715317674,1.46103715437746));
#41613=CARTESIAN_POINT('Ctrl Pts',(-39.,49.1351612200714,1.75646310440614));
#41614=CARTESIAN_POINT('Ctrl Pts',(-39.,48.4294569765608,1.19691209180873));
#41615=CARTESIAN_POINT('Ctrl Pts',(-38.2293353682963,48.7723498350628,1.44196991828834));
#41616=CARTESIAN_POINT('Ctrl Pts',(-39.,49.1528920190527,1.76047367398439));
#41617=CARTESIAN_POINT('Ctrl Pts',(-39.,48.4502143494671,1.17149348979916));
#41618=CARTESIAN_POINT('Ctrl Pts',(-38.2172524228879,48.7938107755338,1.40570983381058));
#41619=CARTESIAN_POINT('Ctrl Pts',(-39.,49.1854965841077,1.77268752052089));
#41620=CARTESIAN_POINT('Ctrl Pts',(-39.,48.4931364697057,1.12315562043586));
#41621=CARTESIAN_POINT('Ctrl Pts',(-38.2115234085426,48.8048934041713,1.38851698622487));
#41622=CARTESIAN_POINT('Ctrl Pts',(-39.,49.2002608324643,1.78099665448271));
#41623=CARTESIAN_POINT('Ctrl Pts',(-39.,48.5153011996989,1.10023637266547));
#41624=CARTESIAN_POINT('Ctrl Pts',(-38.2007290458784,48.8276880282294,1.35612215636338));
#41625=CARTESIAN_POINT('Ctrl Pts',(-39.,49.2259038684558,1.80129243318477));
#41626=CARTESIAN_POINT('Ctrl Pts',(-39.,48.5608879792475,1.05705237794022));
#41627=CARTESIAN_POINT('Ctrl Pts',(-38.195663662783,48.8394001036726,1.34092007054188));
#41628=CARTESIAN_POINT('Ctrl Pts',(-39.0000000000001,49.236644940001,1.81335075777812));
#41629=CARTESIAN_POINT('Ctrl Pts',(-39.,48.5843100738694,1.03678759836947));
#41630=CARTESIAN_POINT('Ctrl Pts',(-38.190947298471,48.851387088898,1.32676510440455));
#41631=CARTESIAN_POINT('Ctrl Pts',(-39.,49.2448593423298,1.82664018134291));
#41632=CARTESIAN_POINT('Ctrl Pts',(-39.,48.6082814197213,1.01791876511632));
#41633=CARTESIAN_POINT('',(-38.5000013347617,48.5946171140508,2.25361874077735));
#41634=CARTESIAN_POINT('',(-39.,48.5946168149163,1.02887446815399));
#41635=CARTESIAN_POINT('Ctrl Pts',(-38.5000036709582,48.5946177418629,2.25361738261186));
#41636=CARTESIAN_POINT('Ctrl Pts',(-38.5088353775067,48.5946177418629,2.23831416931868));
#41637=CARTESIAN_POINT('Ctrl Pts',(-38.5118644338839,48.5946168001396,2.23312624335332));
#41638=CARTESIAN_POINT('Ctrl Pts',(-38.6044346062607,48.5946168001396,2.07241374470279));
#41639=CARTESIAN_POINT('Ctrl Pts',(-38.7257091353047,48.5946168001447,1.86441097587205));
#41640=CARTESIAN_POINT('Ctrl Pts',(-38.8689400035351,48.5946168001447,1.56477839703979));
#41641=CARTESIAN_POINT('Ctrl Pts',(-38.916056425514,48.5946168001447,1.45350707240695));
#41642=CARTESIAN_POINT('Ctrl Pts',(-38.979760764433,48.5946168001447,1.24081758397416));
#41643=CARTESIAN_POINT('Ctrl Pts',(-39.000000003693,48.5946168001447,1.13498028931347));
#41644=CARTESIAN_POINT('Ctrl Pts',(-39.,48.5946168001447,1.02887446815399));
#41645=CARTESIAN_POINT('',(-38.8535533905933,49.0946168001447,3.31427946513778));
#41646=CARTESIAN_POINT('Origin',(-38.4999999999997,49.0946168001451,2.25361929335716));
#41647=CARTESIAN_POINT('',(-39.,49.0946168001447,3.66783285573106));
#41648=CARTESIAN_POINT('Origin',(-38.5,49.0946168001447,3.66783285573106));
#41649=CARTESIAN_POINT('Origin',(-39.,49.0946260151291,2.25361684509152));
#41650=CARTESIAN_POINT('Origin',(-38.5,34.999999994595,3.66783285573106));
#41651=CARTESIAN_POINT('',(-38.8535533905933,51.0871688613417,3.31427946513778));
#41652=CARTESIAN_POINT('',(-38.8535533905933,48.5946168001447,3.31427946513778));
#41653=CARTESIAN_POINT('',(-39.,51.0871688613417,3.66783285573106));
#41654=CARTESIAN_POINT('Origin',(-38.5,51.0871688613417,3.66783285573106));
#41655=CARTESIAN_POINT('',(-39.,34.999999994595,3.66783285573106));
#41656=CARTESIAN_POINT('Ctrl Pts',(-39.0004132136994,51.0650382190915,3.67320198015863));
#41657=CARTESIAN_POINT('Ctrl Pts',(-39.0026470813632,51.0568537778256,3.46336368637365));
#41658=CARTESIAN_POINT('Ctrl Pts',(-38.8543685602191,51.045166200389,3.31509463512307));
#41659=CARTESIAN_POINT('Ctrl Pts',(-38.9993650281416,51.0933835567273,3.66532101541981));
#41660=CARTESIAN_POINT('Ctrl Pts',(-38.9983197911702,51.0954158980446,3.45903672724059));
#41661=CARTESIAN_POINT('Ctrl Pts',(-38.8522723311024,51.0987408007483,3.31299840599475));
#41662=CARTESIAN_POINT('Ctrl Pts',(-39.0003073665066,51.1207747726147,3.6614931211168));
#41663=CARTESIAN_POINT('Ctrl Pts',(-38.9976874728413,51.1334658286751,3.45840463886212));
#41664=CARTESIAN_POINT('Ctrl Pts',(-38.8541571729459,51.1513558166005,3.31488324783015));
#41665=CARTESIAN_POINT('Ctrl Pts',(-39.0054754132473,51.1666975933268,3.66193564327231));
#41666=CARTESIAN_POINT('Ctrl Pts',(-39.0031011742983,51.1978659396949,3.46381856720568));
#41667=CARTESIAN_POINT('Ctrl Pts',(-38.8644936257713,51.2410601515156,3.32521970064757));
#41668=CARTESIAN_POINT('Ctrl Pts',(-39.0087733936485,51.1856684908119,3.66434215081685));
#41669=CARTESIAN_POINT('Ctrl Pts',(-39.0074314446558,51.2247144410629,3.46814888026069));
#41670=CARTESIAN_POINT('Ctrl Pts',(-38.8710897498968,51.2785995319265,3.33181582477153));
#41671=CARTESIAN_POINT('Ctrl Pts',(-39.0143549183491,51.2087029404423,3.6702511952005));
#41672=CARTESIAN_POINT('Ctrl Pts',(-39.0154875060493,51.2574656215126,3.47620492597015));
#41673=CARTESIAN_POINT('Ctrl Pts',(-38.8822530434418,51.3248177772951,3.34297911831711));
#41674=CARTESIAN_POINT('Ctrl Pts',(-39.0155448251913,51.2132751460628,3.67157941317018));
#41675=CARTESIAN_POINT('Ctrl Pts',(-39.0172324883617,51.2639770516779,3.47794990165795));
#41676=CARTESIAN_POINT('Ctrl Pts',(-38.8846329063861,51.3340250290864,3.3453589812617));
#41677=CARTESIAN_POINT('Ctrl Pts',(-39.0180473737812,51.2222620687329,3.67449946007851));
#41678=CARTESIAN_POINT('Ctrl Pts',(-39.0209519414425,51.2767911867937,3.48166933473724));
#41679=CARTESIAN_POINT('Ctrl Pts',(-38.8896381011801,51.3521883956118,3.35036417605639));
#41680=CARTESIAN_POINT('Ctrl Pts',(-39.019362676268,51.2266883046425,3.67609400270875));
#41681=CARTESIAN_POINT('Ctrl Pts',(-39.0229304708662,51.2831109734046,3.48364785077913));
#41682=CARTESIAN_POINT('Ctrl Pts',(-38.8922687593557,51.3611675700846,3.35299483423247));
#41683=CARTESIAN_POINT('Ctrl Pts',(-39.0234967000298,51.2397696792542,3.68127177968089));
#41684=CARTESIAN_POINT('Ctrl Pts',(-39.0292136522808,51.3018106261032,3.48993098214682));
#41685=CARTESIAN_POINT('Ctrl Pts',(-38.9005369597166,51.3878039362001,3.36126303459511));
#41686=CARTESIAN_POINT('Ctrl Pts',(-39.0265033515949,51.248227685921,3.68524877806938));
#41687=CARTESIAN_POINT('Ctrl Pts',(-39.0338657297898,51.3139294225388,3.49458301308925));
#41688=CARTESIAN_POINT('Ctrl Pts',(-38.9065503741551,51.4051602537286,3.36727644903522));
#41689=CARTESIAN_POINT('Ctrl Pts',(-39.0362506360782,51.2728396274532,3.69869584278333));
#41690=CARTESIAN_POINT('Ctrl Pts',(-39.0491554140162,51.3492559657486,3.50987251941062));
#41691=CARTESIAN_POINT('Ctrl Pts',(-38.9260452743275,51.4560647988364,3.38677134921394));
#41692=CARTESIAN_POINT('Ctrl Pts',(-39.0437160920884,51.2882342797459,3.7096765772377));
#41693=CARTESIAN_POINT('Ctrl Pts',(-39.0611272669598,51.3714257050568,3.52184420280592));
#41694=CARTESIAN_POINT('Ctrl Pts',(-38.9409764285494,51.4884526127531,3.40170250344182));
#41695=CARTESIAN_POINT('Ctrl Pts',(-39.0542165012263,51.306253347527,3.72581511285224));
#41696=CARTESIAN_POINT('Ctrl Pts',(-39.0781424378334,51.3973171852378,3.53885910063643));
#41697=CARTESIAN_POINT('Ctrl Pts',(-38.9619775702996,51.5270665421227,3.42270364520152));
#41698=CARTESIAN_POINT('Ctrl Pts',(-39.0563797411747,51.3098026213536,3.72917101376348));
#41699=CARTESIAN_POINT('Ctrl Pts',(-39.0816629307715,51.4024242807893,3.54237953564933));
#41700=CARTESIAN_POINT('Ctrl Pts',(-38.9663041175394,51.5347104471688,3.42703019244338));
#41701=CARTESIAN_POINT('Ctrl Pts',(-39.0607958470836,51.3167363106842,3.73608090526937));
#41702=CARTESIAN_POINT('Ctrl Pts',(-39.0888670320053,51.4123984763779,3.54958351557072));
#41703=CARTESIAN_POINT('Ctrl Pts',(-38.975136458622,51.5497194020163,3.43586253353023));
#41704=CARTESIAN_POINT('Ctrl Pts',(-39.0630486386578,51.3201214581943,3.73963462669351));
#41705=CARTESIAN_POINT('Ctrl Pts',(-39.0925510010862,51.4172668812864,3.55326742126279));
#41706=CARTESIAN_POINT('Ctrl Pts',(-38.9796421118285,51.5570858174706,3.44036818673893));
#41707=CARTESIAN_POINT('Ctrl Pts',(-39.0699366073489,51.3300401544233,3.75058117469492));
#41708=CARTESIAN_POINT('Ctrl Pts',(-39.1038433226588,51.4315326049623,3.56455954462027));
#41709=CARTESIAN_POINT('Ctrl Pts',(-38.9934182473023,51.5787851825119,3.45414432221952));
#41710=CARTESIAN_POINT('Ctrl Pts',(-39.0747012126549,51.3363372494979,3.75825902842783));
#41711=CARTESIAN_POINT('Ctrl Pts',(-39.1116821357186,51.4405754880574,3.57239821496679));
#41712=CARTESIAN_POINT('Ctrl Pts',(-39.0029476009635,51.5927187236375,3.46367367588575));
#41713=CARTESIAN_POINT('Ctrl Pts',(-39.0894825144253,51.3543368021546,3.78236118822114));
#41714=CARTESIAN_POINT('Ctrl Pts',(-39.1360937469245,51.4664061341308,3.5968093671278));
#41715=CARTESIAN_POINT('Ctrl Pts',(-39.0325106179011,51.6330150924322,3.49323669283907));
#41716=CARTESIAN_POINT('Ctrl Pts',(-39.099984848889,51.3651509597073,3.79984981751613));
#41717=CARTESIAN_POINT('Ctrl Pts',(-39.1535206447848,51.4818344395588,3.61423591843403));
#41718=CARTESIAN_POINT('Ctrl Pts',(-39.0535155850355,51.657879312988,3.51424165998539));
#41719=CARTESIAN_POINT('Ctrl Pts',(-39.1166298330874,51.3797350133674,3.82802206864364));
#41720=CARTESIAN_POINT('Ctrl Pts',(-39.1811244902722,51.5024247355477,3.64183918729206));
#41721=CARTESIAN_POINT('Ctrl Pts',(-39.0868060117716,51.6924247339652,3.54753208674103));
#41722=CARTESIAN_POINT('Ctrl Pts',(-39.1223391592955,51.3843292933444,3.83775804229266));
#41723=CARTESIAN_POINT('Ctrl Pts',(-39.1906195944728,51.5088870560383,3.6513340886733));
#41724=CARTESIAN_POINT('Ctrl Pts',(-39.0982248234841,51.7034975154818,3.55895089846032));
#41725=CARTESIAN_POINT('Ctrl Pts',(-39.1339020438763,51.3928845223354,3.85760749410021));
#41726=CARTESIAN_POINT('Ctrl Pts',(-39.2098534044357,51.5208432398919,3.67056747890522));
#41727=CARTESIAN_POINT('Ctrl Pts',(-39.1213509013222,51.7244996054785,3.58207697631249));
#41728=CARTESIAN_POINT('Ctrl Pts',(-39.1397709861723,51.396860516286,3.8677467521508));
#41729=CARTESIAN_POINT('Ctrl Pts',(-39.2196213133971,51.5263568494977,3.68033517032777));
#41730=CARTESIAN_POINT('Ctrl Pts',(-39.1330889487652,51.7344638113003,3.59381502376268));
#41731=CARTESIAN_POINT('Ctrl Pts',(-39.157621772381,51.4079454815182,3.89876073152793));
#41732=CARTESIAN_POINT('Ctrl Pts',(-39.2493801680053,51.5416207945294,3.71009334903438));
#41733=CARTESIAN_POINT('Ctrl Pts',(-39.1687909902807,51.7628597814416,3.62951706530047));
#41734=CARTESIAN_POINT('Ctrl Pts',(-39.1698466131479,51.4142147039408,3.92022917339187));
#41735=CARTESIAN_POINT('Ctrl Pts',(-39.269729837374,51.5500260923023,3.7304425387748));
#41736=CARTESIAN_POINT('Ctrl Pts',(-39.1932410033856,51.7798007004865,3.65396707842107));
#41737=CARTESIAN_POINT('Ctrl Pts',(-39.1948753371907,51.4247405914866,3.96457564423585));
#41738=CARTESIAN_POINT('Ctrl Pts',(-39.3112907465306,51.5636693356107,3.77200243192297));
#41739=CARTESIAN_POINT('Ctrl Pts',(-39.2432991138983,51.8101301358283,3.70402518896648));
#41740=CARTESIAN_POINT('Ctrl Pts',(-39.2076795776735,51.4289960250896,3.98745463026039));
#41741=CARTESIAN_POINT('Ctrl Pts',(-39.3325285954283,51.5688838290406,3.79323974347319));
#41742=CARTESIAN_POINT('Ctrl Pts',(-39.2689079376051,51.8235164183283,3.72963401269037));
#41743=CARTESIAN_POINT('Ctrl Pts',(-39.2240205469469,51.4331410531779,4.01687032803402));
#41744=CARTESIAN_POINT('Ctrl Pts',(-39.3594337885762,51.573511040252,3.82014423116445));
#41745=CARTESIAN_POINT('Ctrl Pts',(-39.3015903184586,51.8381899496214,3.76231639356608));
#41746=CARTESIAN_POINT('Ctrl Pts',(-39.2273055765702,51.433911163606,4.02279445562467));
#41747=CARTESIAN_POINT('Ctrl Pts',(-39.3648581334168,51.5743449115587,3.82556843254212));
#41748=CARTESIAN_POINT('Ctrl Pts',(-39.3081604657371,51.8410213644416,3.76888654084901));
#41749=CARTESIAN_POINT('Ctrl Pts',(-39.2339088376195,51.435335041245,4.03472357381184));
#41750=CARTESIAN_POINT('Ctrl Pts',(-39.375751971054,51.5758253293304,3.83646197951802));
#41751=CARTESIAN_POINT('Ctrl Pts',(-39.3213671634083,51.8464805041875,3.78209323852921));
#41752=CARTESIAN_POINT('Ctrl Pts',(-39.2372263299055,51.4359884597313,4.04072726345858));
#41753=CARTESIAN_POINT('Ctrl Pts',(-39.3812205639743,51.5764709767064,3.84193042525364));
#41754=CARTESIAN_POINT('Ctrl Pts',(-39.3280022373104,51.8491072615919,3.78872831243597));
#41755=CARTESIAN_POINT('Ctrl Pts',(-39.247178880307,51.4377685199949,4.05876895738201));
#41756=CARTESIAN_POINT('Ctrl Pts',(-39.3976316833915,51.5781249620217,3.8583410990863));
#41757=CARTESIAN_POINT('Ctrl Pts',(-39.3479076001771,51.8566508805564,3.8086336753163));
#41758=CARTESIAN_POINT('Ctrl Pts',(-39.2538303336714,51.4387188350674,4.07086701947127));
#41759=CARTESIAN_POINT('Ctrl Pts',(-39.408566396275,51.5788476114369,3.86927550987494));
#41760=CARTESIAN_POINT('Ctrl Pts',(-39.3612106868366,51.8612452314633,3.82193676198504));
#41761=CARTESIAN_POINT('Ctrl Pts',(-39.2738310197503,51.4409006831208,4.10736021368593));
#41762=CARTESIAN_POINT('Ctrl Pts',(-39.4414609831924,51.579951033028,3.90216917193513));
#41763=CARTESIAN_POINT('Ctrl Pts',(-39.4012125847243,51.8738020065102,3.86193865990074));
#41764=CARTESIAN_POINT('Ctrl Pts',(-39.287226430121,51.4414651042384,4.13195370041893));
#41765=CARTESIAN_POINT('Ctrl Pts',(-39.4633483665596,51.5792419677428,3.92405591822746));
#41766=CARTESIAN_POINT('Ctrl Pts',(-39.4280037683589,51.8805418579184,3.88872984355429));
#41767=CARTESIAN_POINT('Ctrl Pts',(-39.3141290116621,51.4409682547149,4.1816268682295));
#41768=CARTESIAN_POINT('Ctrl Pts',(-39.5070603581384,51.575219794606,3.9677665909243));
#41769=CARTESIAN_POINT('Ctrl Pts',(-39.481809658417,51.891062996906,3.94253573365096));
#41770=CARTESIAN_POINT('Ctrl Pts',(-39.3276362284429,51.4399063106198,4.20670677175969));
#41771=CARTESIAN_POINT('Ctrl Pts',(-39.5288968108741,51.5718749448291,3.98960236096735));
#41772=CARTESIAN_POINT('Ctrl Pts',(-39.5088244614836,51.8948429910834,3.9695505367372));
#41773=CARTESIAN_POINT('Ctrl Pts',(-39.354755051824,51.4362532171509,4.25732900698769));
#41774=CARTESIAN_POINT('Ctrl Pts',(-39.5724437164635,51.5627206322971,4.03314785302545));
#41775=CARTESIAN_POINT('Ctrl Pts',(-39.5630628536111,51.8996395002578,4.02378892890451));
#41776=CARTESIAN_POINT('Ctrl Pts',(-39.3683666837519,51.4336617002444,4.28287145663512));
#41777=CARTESIAN_POINT('Ctrl Pts',(-39.5941655928019,51.556877959299,4.05486899752503));
#41778=CARTESIAN_POINT('Ctrl Pts',(-39.5902864954815,51.9006553017652,4.05101257079516));
#41779=CARTESIAN_POINT('Ctrl Pts',(-39.3888590555512,51.428669185987,4.32152453598587));
#41780=CARTESIAN_POINT('Ctrl Pts',(-39.6265016106641,51.5463603767316,4.08720388162891));
#41781=CARTESIAN_POINT('Ctrl Pts',(-39.6312718225881,51.9001955452795,4.09199789793255));
#41782=CARTESIAN_POINT('Ctrl Pts',(-39.3957023535762,51.4268205187815,4.33446556245966));
#41783=CARTESIAN_POINT('Ctrl Pts',(-39.6372928076184,51.5425385825794,4.09799469263457));
#41784=CARTESIAN_POINT('Ctrl Pts',(-39.6449586117414,51.8997111781368,4.10568468709613));
#41785=CARTESIAN_POINT('Ctrl Pts',(-39.4094136202798,51.4227580259902,4.36046079000117));
#41786=CARTESIAN_POINT('Ctrl Pts',(-39.6588203038909,51.5342999415303,4.11952140291209));
#41787=CARTESIAN_POINT('Ctrl Pts',(-39.6723815340093,51.8980893379141,4.13310760938484));
#41788=CARTESIAN_POINT('Ctrl Pts',(-39.4162677663881,51.4205477358223,4.37348889242158));
#41789=CARTESIAN_POINT('Ctrl Pts',(-39.669535476702,51.5298861426874,4.13023617631423));
#41790=CARTESIAN_POINT('Ctrl Pts',(-39.6860900219729,51.8969524844333,4.146816097359));
#41791=CARTESIAN_POINT('Ctrl Pts',(-39.4503663607577,51.4086820482238,4.43846668905814));
#41792=CARTESIAN_POINT('Ctrl Pts',(-39.7231418979962,51.5062754902456,4.18384055660646));
#41793=CARTESIAN_POINT('Ctrl Pts',(-39.7542881428281,51.8897219185405,4.2150142182665));
#41794=CARTESIAN_POINT('Ctrl Pts',(-39.4772582375367,51.3965556312517,4.49023496260712));
#41795=CARTESIAN_POINT('Ctrl Pts',(-39.7642005002811,51.4831753452374,4.22489745473237));
#41796=CARTESIAN_POINT('Ctrl Pts',(-39.8080718615601,51.8790082051072,4.26879793704068));
#41797=CARTESIAN_POINT('Ctrl Pts',(-39.5038019361007,51.3820343130569,4.54185646265653));
#41798=CARTESIAN_POINT('Ctrl Pts',(-39.803134320195,51.4567542175855,4.26382949617694));
#41799=CARTESIAN_POINT('Ctrl Pts',(-39.861160938566,51.8638711179526,4.32188701408911));
#41800=CARTESIAN_POINT('Ctrl Pts',(-39.,51.0871688613417,3.66783285573106));
#41801=CARTESIAN_POINT('Ctrl Pts',(-39.,51.0995964745295,3.66526623270042));
#41802=CARTESIAN_POINT('Ctrl Pts',(-39.0003980980124,51.1120315517898,3.66346660688227));
#41803=CARTESIAN_POINT('Ctrl Pts',(-39.0012397064956,51.1244742900618,3.66251648874842));
#41804=CARTESIAN_POINT('Ctrl Pts',(-39.0017520306939,51.132048733567,3.66193810994057));
#41805=CARTESIAN_POINT('Ctrl Pts',(-39.0024288183487,51.1396258232086,3.66167471989657));
#41806=CARTESIAN_POINT('Ctrl Pts',(-39.0032819045167,51.1472062783665,3.66174775116153));
#41807=CARTESIAN_POINT('Ctrl Pts',(-39.003830205514,51.152078436981,3.66179469028316));
#41808=CARTESIAN_POINT('Ctrl Pts',(-39.0044513162621,51.1569520679716,3.66198055458152));
#41809=CARTESIAN_POINT('Ctrl Pts',(-39.0051494245821,51.1618268948852,3.66231306057799));
#41810=CARTESIAN_POINT('Ctrl Pts',(-39.0055954934587,51.1649417532861,3.66252552126937));
#41811=CARTESIAN_POINT('Ctrl Pts',(-39.006073011082,51.1680571554945,3.66279782153449));
#41812=CARTESIAN_POINT('Ctrl Pts',(-39.0065831559074,51.1711730884579,3.6631321412611));
#41813=CARTESIAN_POINT('Ctrl Pts',(-39.0070933007329,51.1742890214214,3.66346646098771));
#41814=CARTESIAN_POINT('Ctrl Pts',(-39.0076356421744,51.1774019318785,3.6638627061799));
#41815=CARTESIAN_POINT('Ctrl Pts',(-39.0082068784871,51.1804909131394,3.66431876730514));
#41816=CARTESIAN_POINT('Ctrl Pts',(-39.0093493511126,51.186668875661,3.66523088955563));
#41817=CARTESIAN_POINT('Ctrl Pts',(-39.0106111129066,51.1927743436604,3.66638458995328));
#41818=CARTESIAN_POINT('Ctrl Pts',(-39.0119924837342,51.1988072949574,3.66777962771153));
#41819=CARTESIAN_POINT('Ctrl Pts',(-39.0123974891622,51.2005761016917,3.66818864015996));
#41820=CARTESIAN_POINT('Ctrl Pts',(-39.0128129276482,51.2023393171679,3.66861857412582));
#41821=CARTESIAN_POINT('Ctrl Pts',(-39.0132386139189,51.2040960879642,3.66906923077199));
#41822=CARTESIAN_POINT('Ctrl Pts',(-39.0142648355865,51.2083312169324,3.67015564968387));
#41823=CARTESIAN_POINT('Ctrl Pts',(-39.0153512215115,51.2125280987449,3.67136380075719));
#41824=CARTESIAN_POINT('Ctrl Pts',(-39.0164841144222,51.216642004501,3.67267657739539));
#41825=CARTESIAN_POINT('Ctrl Pts',(-39.0165877103608,51.2170181953343,3.67279662257064));
#41826=CARTESIAN_POINT('Ctrl Pts',(-39.0166917083802,51.2173937442946,3.67291755655674));
#41827=CARTESIAN_POINT('Ctrl Pts',(-39.0167961002917,51.2177686258567,3.67303936883383));
#41828=CARTESIAN_POINT('Ctrl Pts',(-39.0180523386729,51.2222799007215,3.67450524157719));
#41829=CARTESIAN_POINT('Ctrl Pts',(-39.0193683093485,51.2267061299586,3.67610105605805));
#41830=CARTESIAN_POINT('Ctrl Pts',(-39.0207406841958,51.2310487629442,3.67781992804404));
#41831=CARTESIAN_POINT('Ctrl Pts',(-39.0210187256343,51.2319285749902,3.67816816937228));
#41832=CARTESIAN_POINT('Ctrl Pts',(-39.0212990800108,51.232804958106,3.67852145716376));
#41833=CARTESIAN_POINT('Ctrl Pts',(-39.0215817215748,51.2336779220825,3.6788797386022));
#41834=CARTESIAN_POINT('Ctrl Pts',(-39.0241236459549,51.2415288849186,3.68210192684084));
#41835=CARTESIAN_POINT('Ctrl Pts',(-39.0268515468469,51.2491069283234,3.68572893466199));
#41836=CARTESIAN_POINT('Ctrl Pts',(-39.0297524567615,51.2564317442274,3.68973091949866));
#41837=CARTESIAN_POINT('Ctrl Pts',(-39.0309454699727,51.2594441101403,3.6913767550888));
#41838=CARTESIAN_POINT('Ctrl Pts',(-39.0321676781911,51.2624137209571,3.6930858697691));
#41839=CARTESIAN_POINT('Ctrl Pts',(-39.0334184549677,51.2653416363956,3.69485679380877));
#41840=CARTESIAN_POINT('Ctrl Pts',(-39.0355645267475,51.2703653279237,3.69789532968244));
#41841=CARTESIAN_POINT('Ctrl Pts',(-39.0377946841974,51.2752663367985,3.70111548255788));
#41842=CARTESIAN_POINT('Ctrl Pts',(-39.0401058114859,51.2800494365045,3.70451004803446));
#41843=CARTESIAN_POINT('Ctrl Pts',(-39.0424169387745,51.2848325362106,3.70790461351104));
#41844=CARTESIAN_POINT('Ctrl Pts',(-39.0448144637063,51.2895066993963,3.71148200120225));
#41845=CARTESIAN_POINT('Ctrl Pts',(-39.0472643549682,51.294022166229,3.71518767696938));
#41846=CARTESIAN_POINT('Ctrl Pts',(-39.0488581606738,51.2969597565267,3.71759844812181));
#41847=CARTESIAN_POINT('Ctrl Pts',(-39.0504759635781,51.2998344601907,3.72006609450073));
#41848=CARTESIAN_POINT('Ctrl Pts',(-39.0521164252352,51.3026495570621,3.72258735743621));
#41849=CARTESIAN_POINT('Ctrl Pts',(-39.0529975712403,51.304161638342,3.72394161082802));
#41850=CARTESIAN_POINT('Ctrl Pts',(-39.053886084437,51.305657685124,3.72531266237347));
#41851=CARTESIAN_POINT('Ctrl Pts',(-39.0547804720049,51.307136108471,3.72669801456886));
#41852=CARTESIAN_POINT('Ctrl Pts',(-39.0560387467964,51.3092160376823,3.72864700604342));
#41853=CARTESIAN_POINT('Ctrl Pts',(-39.0573092698283,51.3112620946395,3.73062532617036));
#41854=CARTESIAN_POINT('Ctrl Pts',(-39.0585878042399,51.3132695017008,3.73262588877138));
#41855=CARTESIAN_POINT('Ctrl Pts',(-39.0599099821681,51.3153454327708,3.73469474174153));
#41856=CARTESIAN_POINT('Ctrl Pts',(-39.0612407201129,51.3173803278842,3.73678731392401));
#41857=CARTESIAN_POINT('Ctrl Pts',(-39.0625790831881,51.3193756616965,3.73890147686224));
#41858=CARTESIAN_POINT('Ctrl Pts',(-39.0634971743549,51.3207444220738,3.74035175172014));
#41859=CARTESIAN_POINT('Ctrl Pts',(-39.0644190730827,51.3220948885419,3.74181255620632));
#41860=CARTESIAN_POINT('Ctrl Pts',(-39.0653446285659,51.3234276913672,3.74328347395578));
#41861=CARTESIAN_POINT('Ctrl Pts',(-39.0697269764318,51.3297382861638,3.75024801943863));
#41862=CARTESIAN_POINT('Ctrl Pts',(-39.0741907292571,51.335653921141,3.75743801365242));
#41863=CARTESIAN_POINT('Ctrl Pts',(-39.0787251755062,51.3412317605606,3.7648214335795));
#41864=CARTESIAN_POINT('Ctrl Pts',(-39.0790259119933,51.3416016976466,3.7653111215478));
#41865=CARTESIAN_POINT('Ctrl Pts',(-39.0793269611165,51.3419701450682,3.76580166465627));
#41866=CARTESIAN_POINT('Ctrl Pts',(-39.0796283193631,51.3423371166535,3.76629305339742));
#41867=CARTESIAN_POINT('Ctrl Pts',(-39.0848304408808,51.3486718720562,3.77477552890059));
#41868=CARTESIAN_POINT('Ctrl Pts',(-39.0901237073089,51.3545686231568,3.78350778594277));
#41869=CARTESIAN_POINT('Ctrl Pts',(-39.095497076649,51.3600855765314,3.79245708285084));
#41870=CARTESIAN_POINT('Ctrl Pts',(-39.1006217790422,51.3653472182263,3.80099222726015));
#41871=CARTESIAN_POINT('Ctrl Pts',(-39.1058203796004,51.3702639537623,3.80972667229477));
#41872=CARTESIAN_POINT('Ctrl Pts',(-39.1110815409305,51.3748737334003,3.81863120842067));
#41873=CARTESIAN_POINT('Ctrl Pts',(-39.1116563965401,51.375377416431,3.81960415378795));
#41874=CARTESIAN_POINT('Ctrl Pts',(-39.1122321348346,51.3758774922222,3.82057937166501));
#41875=CARTESIAN_POINT('Ctrl Pts',(-39.1128086511915,51.376373938695,3.82155667121885));
#41876=CARTESIAN_POINT('Ctrl Pts',(-39.1157350897341,51.3788939367406,3.82651751412991));
#41877=CARTESIAN_POINT('Ctrl Pts',(-39.1186865170056,51.3813245163271,3.8315404301615));
#41878=CARTESIAN_POINT('Ctrl Pts',(-39.1216416073541,51.3836558244275,3.83658791440293));
#41879=CARTESIAN_POINT('Ctrl Pts',(-39.1237991846949,51.385357964443,3.84027319517036));
#41880=CARTESIAN_POINT('Ctrl Pts',(-39.1259597623763,51.3870081589385,3.84397323953785));
#41881=CARTESIAN_POINT('Ctrl Pts',(-39.1281206119593,51.388606926004,3.84768274132748));
#41882=CARTESIAN_POINT('Ctrl Pts',(-39.1289193344976,51.3891978839766,3.8490538977043));
#41883=CARTESIAN_POINT('Ctrl Pts',(-39.129718392079,51.3897821006618,3.85042684643276));
#41884=CARTESIAN_POINT('Ctrl Pts',(-39.130517872912,51.3903597745074,3.85180170705767));
#41885=CARTESIAN_POINT('Ctrl Pts',(-39.1355759629898,51.3940145542418,3.86050006303806));
#41886=CARTESIAN_POINT('Ctrl Pts',(-39.1406441791352,51.3974027997912,3.86926363808882));
#41887=CARTESIAN_POINT('Ctrl Pts',(-39.1457212999534,51.4005555854721,3.87808462932063));
#41888=CARTESIAN_POINT('Ctrl Pts',(-39.1465912344662,51.4010957965826,3.87959605380399));
#41889=CARTESIAN_POINT('Ctrl Pts',(-39.1474614280801,51.4016291023346,3.88110915797035));
#41890=CARTESIAN_POINT('Ctrl Pts',(-39.1483318837667,51.4021556272645,3.88262392648645));
#41891=CARTESIAN_POINT('Ctrl Pts',(-39.1586945751745,51.4084238560221,3.90065710029224));
#41892=CARTESIAN_POINT('Ctrl Pts',(-39.1690947653013,51.4137357364453,3.91892451423044));
#41893=CARTESIAN_POINT('Ctrl Pts',(-39.179525285691,51.4182657071134,3.93738118482275));
#41894=CARTESIAN_POINT('Ctrl Pts',(-39.1804702750404,51.4186761155949,3.93905333122413));
#41895=CARTESIAN_POINT('Ctrl Pts',(-39.1814155213493,51.4190800785542,3.9407270510575));
#41896=CARTESIAN_POINT('Ctrl Pts',(-39.1823610239388,51.4194777096985,3.9424023224895));
#41897=CARTESIAN_POINT('Ctrl Pts',(-39.1829649779349,51.4197317025709,3.94347242730691));
#41898=CARTESIAN_POINT('Ctrl Pts',(-39.1835690373468,51.4199831090079,3.944543167478));
#41899=CARTESIAN_POINT('Ctrl Pts',(-39.184173203649,51.4202319529509,3.94561454164697));
#41900=CARTESIAN_POINT('Ctrl Pts',(-39.1961630588975,51.4251703330717,3.96687627232667));
#41901=CARTESIAN_POINT('Ctrl Pts',(-39.2081930739204,51.4291022904702,3.98838303756631));
#41902=CARTESIAN_POINT('Ctrl Pts',(-39.2202572512408,51.4321859850981,4.01009600071619));
#41903=CARTESIAN_POINT('Ctrl Pts',(-39.2204222834166,51.4322281685657,4.01039302366748));
#41904=CARTESIAN_POINT('Ctrl Pts',(-39.2205873201454,51.4322701922361,4.01069008198365));
#41905=CARTESIAN_POINT('Ctrl Pts',(-39.2207523616119,51.4323120565271,4.01098717593383));
#41906=CARTESIAN_POINT('Ctrl Pts',(-39.2240348618836,51.4331446930114,4.01689606048839));
#41907=CARTESIAN_POINT('Ctrl Pts',(-39.2273192800592,51.4339141314245,4.02281915981079));
#41908=CARTESIAN_POINT('Ctrl Pts',(-39.2306072248842,51.4346231203129,4.02875898953522));
#41909=CARTESIAN_POINT('Ctrl Pts',(-39.2331963988375,51.435181431252,4.03343645622905));
#41910=CARTESIAN_POINT('Ctrl Pts',(-39.2357872865129,51.4357020312782,4.03812346513848));
#41911=CARTESIAN_POINT('Ctrl Pts',(-39.2383733317665,51.4361850310234,4.04280792575837));
#41912=CARTESIAN_POINT('Ctrl Pts',(-39.239097131351,51.4363202162118,4.04411904382396));
#41913=CARTESIAN_POINT('Ctrl Pts',(-39.2398206954841,51.4364524822294,4.04543022127291));
#41914=CARTESIAN_POINT('Ctrl Pts',(-39.2405438557811,51.436581821874,4.04674114905286));
#41915=CARTESIAN_POINT('Ctrl Pts',(-39.2458504974744,51.4375309325395,4.0563609028517));
#41916=CARTESIAN_POINT('Ctrl Pts',(-39.251145838485,51.4383249425886,4.06598604764607));
#41917=CARTESIAN_POINT('Ctrl Pts',(-39.2564276221927,51.4389741257984,4.07561075929201));
#41918=CARTESIAN_POINT('Ctrl Pts',(-39.2577849792638,51.4391409583438,4.07808419840524));
#41919=CARTESIAN_POINT('Ctrl Pts',(-39.2591415164243,51.4392982345284,4.08055774959127));
#41920=CARTESIAN_POINT('Ctrl Pts',(-39.260497242635,51.439446129712,4.08303140018469));
#41921=CARTESIAN_POINT('Ctrl Pts',(-39.2711302077067,51.4406060721175,4.10243224981992));
#41922=CARTESIAN_POINT('Ctrl Pts',(-39.2817131423343,51.4411909085124,4.1218386024189));
#41923=CARTESIAN_POINT('Ctrl Pts',(-39.2922518059041,51.4412652877384,4.14125077550199));
#41924=CARTESIAN_POINT('Ctrl Pts',(-39.2950635958798,51.4412851326419,4.14643008057427));
#41925=CARTESIAN_POINT('Ctrl Pts',(-39.2978722688055,51.4412685850813,4.15160990753937));
#41926=CARTESIAN_POINT('Ctrl Pts',(-39.3006778532916,51.4412167771412,4.15679013282812));
#41927=CARTESIAN_POINT('Ctrl Pts',(-39.3142541806936,51.4409660765973,4.18185743516235));
#41928=CARTESIAN_POINT('Ctrl Pts',(-39.3277581609359,51.4398899778444,4.20693402949082));
#41929=CARTESIAN_POINT('Ctrl Pts',(-39.3411957010275,51.4380798014802,4.23201782515537));
#41930=CARTESIAN_POINT('Ctrl Pts',(-39.3484511372291,51.4371024187871,4.24556151528739));
#41931=CARTESIAN_POINT('Ctrl Pts',(-39.3556872284612,51.4359106986094,4.25910740126514));
#41932=CARTESIAN_POINT('Ctrl Pts',(-39.3629052291215,51.4345145275482,4.272656587124));
#41933=CARTESIAN_POINT('Ctrl Pts',(-39.3692939295653,51.4332787672458,4.28464906174185));
#41934=CARTESIAN_POINT('Ctrl Pts',(-39.3756681854211,51.4318828504596,4.296643680088));
#41935=CARTESIAN_POINT('Ctrl Pts',(-39.3820282651167,51.4303333574907,4.30864017603793));
#41936=CARTESIAN_POINT('Ctrl Pts',(-39.3872902770699,51.4290513844788,4.31856547699404));
#41937=CARTESIAN_POINT('Ctrl Pts',(-39.3925425978744,51.42766410719,4.32849212439794));
#41938=CARTESIAN_POINT('Ctrl Pts',(-39.3977854414924,51.4261743730365,4.33842025616291));
#41939=CARTESIAN_POINT('Ctrl Pts',(-39.3993770212168,51.4257221316869,4.3414341574672));
#41940=CARTESIAN_POINT('Ctrl Pts',(-39.4009677741981,51.4252604370354,4.3444482776708));
#41941=CARTESIAN_POINT('Ctrl Pts',(-39.4025579934351,51.4247892753985,4.34746316990157));
#41942=CARTESIAN_POINT('Ctrl Pts',(-39.4067527024737,51.4235464367187,4.35541590710714));
#41943=CARTESIAN_POINT('Ctrl Pts',(-39.4109385157346,51.4222391034398,4.36336422205488));
#41944=CARTESIAN_POINT('Ctrl Pts',(-39.4151134316595,51.4208697596477,4.37130418161823));
#41945=CARTESIAN_POINT('Ctrl Pts',(-39.4177756300927,51.4199965768188,4.37636721720734));
#41946=CARTESIAN_POINT('Ctrl Pts',(-39.420434351826,51.4190978481754,4.38142864884858));
#41947=CARTESIAN_POINT('Ctrl Pts',(-39.4230874920304,51.4181746011217,4.38648444527947));
#41948=CARTESIAN_POINT('Ctrl Pts',(-39.4261723928398,51.4171011088206,4.39236300023734));
#41949=CARTESIAN_POINT('Ctrl Pts',(-39.4292518432436,51.4159941061449,4.39823785994851));
#41950=CARTESIAN_POINT('Ctrl Pts',(-39.4323256432954,51.4148540747936,4.40410862153796));
#41951=CARTESIAN_POINT('Ctrl Pts',(-39.4551952159076,51.4063720560127,4.44778804316367));
#41952=CARTESIAN_POINT('Ctrl Pts',(-39.4777471479169,51.3960634027247,4.49123179831034));
#41953=CARTESIAN_POINT('Ctrl Pts',(-39.500000018719,51.3840965499153,4.53446621502614));
#41954=CARTESIAN_POINT('Origin',(-39.8162486064498,50.8770797377211,4.27697468104505));
#41955=CARTESIAN_POINT('Origin',(-36.5,48.5946168001447,0.960726074544506));
#41956=CARTESIAN_POINT('',(-36.5,49.0946168001447,0.960726074544506));
#41957=CARTESIAN_POINT('',(-36.5,49.0946168001447,0.960726074544506));
#41958=CARTESIAN_POINT('',(-36.5,48.5946168001447,0.960726074544506));
#41959=CARTESIAN_POINT('Origin',(-29.,48.5946168001447,-3.5392739254555));
#41960=CARTESIAN_POINT('',(-36.7071067811865,48.5946168001447,0.460726074544506));
#41961=CARTESIAN_POINT('',(-30.8535533905933,48.5946168001447,-5.39282731604877));
#41962=CARTESIAN_POINT('',(-39.,48.5946168001447,-3.5392739254555));
#41963=CARTESIAN_POINT('',(-33.5,48.5946168001447,-3.5392739254555));
#41964=CARTESIAN_POINT('',(-29.,48.5946168001447,-3.5392739254555));
#41965=CARTESIAN_POINT('',(-33.5,48.5946168001447,0.960726074544506));
#41966=CARTESIAN_POINT('',(-29.,48.5946168001447,0.460726074544506));
#41967=CARTESIAN_POINT('Origin',(-34.5,21.2255401693197,-2.54750793782168));
#41968=CARTESIAN_POINT('',(-38.5,21.2255401693197,4.45249206217833));
#41969=CARTESIAN_POINT('Origin',(-38.5,39.9592920728172,13.6255430020507));
#41970=CARTESIAN_POINT('',(-39.,42.2751240270462,11.7184713306729));
#41971=CARTESIAN_POINT('Ctrl Pts',(-38.5,42.0900494371385,12.3179218587563));
#41972=CARTESIAN_POINT('Ctrl Pts',(-38.5068454246389,42.0900494371385,12.3179218587563));
#41973=CARTESIAN_POINT('Ctrl Pts',(-38.5137049378611,42.0901092205902,12.3177505069324));
#41974=CARTESIAN_POINT('Ctrl Pts',(-38.574487053383,42.0911734302424,12.3146992394163));
#41975=CARTESIAN_POINT('Ctrl Pts',(-38.6266179130002,42.0958133615388,12.3014448852174));
#41976=CARTESIAN_POINT('Ctrl Pts',(-38.7343668418878,42.1126444683801,12.2523913323773));
#41977=CARTESIAN_POINT('Ctrl Pts',(-38.7864380337499,42.1258891023781,12.2133094615048));
#41978=CARTESIAN_POINT('Ctrl Pts',(-38.885076407075,42.1601839674529,12.1084861762414));
#41979=CARTESIAN_POINT('Ctrl Pts',(-38.9288507671719,42.1829880422529,12.0365453528697));
#41980=CARTESIAN_POINT('Ctrl Pts',(-38.9855092027927,42.2295139139639,11.8814589266464));
#41981=CARTESIAN_POINT('Ctrl Pts',(-38.9995659056513,42.2523337408292,11.8018633471128));
#41982=CARTESIAN_POINT('Ctrl Pts',(-38.9999967004912,42.2744474855277,11.7209494981299));
#41983=CARTESIAN_POINT('Ctrl Pts',(-39.,42.2747858712613,11.719710445334));
#41984=CARTESIAN_POINT('Ctrl Pts',(-39.,42.2751240270462,11.7184713306729));
#41985=CARTESIAN_POINT('',(-39.,37.0086337430747,14.1674059193286));
#41986=CARTESIAN_POINT('Ctrl Pts',(-39.,37.0086337430746,14.1674059193286));
#41987=CARTESIAN_POINT('Ctrl Pts',(-39.,37.0677771080364,14.1458794949282));
#41988=CARTESIAN_POINT('Ctrl Pts',(-38.9854014653638,37.1374107416916,14.1205349249739));
#41989=CARTESIAN_POINT('Ctrl Pts',(-38.9377610024774,37.2465671473057,14.0808052424509));
#41990=CARTESIAN_POINT('Ctrl Pts',(-38.8963920732344,37.3055052224255,14.0593535374423));
#41991=CARTESIAN_POINT('Ctrl Pts',(-38.8087985454361,37.3887709311951,14.0290472979151));
#41992=CARTESIAN_POINT('Ctrl Pts',(-38.747240880002,37.428004125326,14.0147675830563));
#41993=CARTESIAN_POINT('Ctrl Pts',(-38.6335018474161,37.4728113710041,13.99845907935));
#41994=CARTESIAN_POINT('Ctrl Pts',(-38.5613457566216,37.4865145651702,13.9934715245592));
#41995=CARTESIAN_POINT('Ctrl Pts',(-38.5,37.4865145651702,13.9934715245592));
#41996=CARTESIAN_POINT('Origin',(-39.,39.9592920728172,13.6255430020507));
#41997=CARTESIAN_POINT('Origin',(-29.,38.5965482096145,9.88143500940095));
#41998=CARTESIAN_POINT('',(-29.,39.4462618578287,12.2160040708718));
#41999=CARTESIAN_POINT('Origin',(-30.,39.4462618578287,12.2160040708718));
#42000=CARTESIAN_POINT('',(-29.,40.4723222878057,15.0350819332295));
#42001=CARTESIAN_POINT('',(-29.,38.5965482096145,9.88143500940095));
#42002=CARTESIAN_POINT('Origin',(-30.,40.4723222878057,15.0350819332295));
#42003=CARTESIAN_POINT('',(-34.,38.5965482096145,9.88143500940095));
#42004=CARTESIAN_POINT('Origin',(-42.5,40.13030214448,14.0953893124436));
#42005=CARTESIAN_POINT('',(-38.5,42.4320695804642,13.2576144795422));
#42006=CARTESIAN_POINT('Origin',(-42.5,39.7882820011544,13.1556966916577));
#42007=CARTESIAN_POINT('',(-38.5,39.7882820011544,13.1556966916577));
#42008=CARTESIAN_POINT('Origin',(-42.5,40.13030214448,14.0953893124436));
#42009=CARTESIAN_POINT('',(-38.5,36.192066340255,15.5287899207029));
#42010=CARTESIAN_POINT('',(-38.5,35.4318390405505,15.805490029072));
#42011=CARTESIAN_POINT('',(-34.22360679775,38.2013139081217,14.7974836127277));
#42012=CARTESIAN_POINT('Origin',(-38.5,39.9592920728172,13.6255430020507));
#42013=CARTESIAN_POINT('',(-39.,38.3487778137292,16.1565988728829));
#42014=CARTESIAN_POINT('Origin',(-38.5,38.3487778137292,16.1565988728829));
#42015=CARTESIAN_POINT('',(-39.,37.6434601185882,15.5326146734285));
#42016=CARTESIAN_POINT('Origin',(-39.,39.9592920728172,13.6255430020507));
#42017=CARTESIAN_POINT('Ctrl Pts',(-38.5,37.8285347084959,14.9331641453451));
#42018=CARTESIAN_POINT('Ctrl Pts',(-38.5068454246389,37.8285347084959,14.9331641453451));
#42019=CARTESIAN_POINT('Ctrl Pts',(-38.5137049378611,37.8284749250441,14.933335497169));
#42020=CARTESIAN_POINT('Ctrl Pts',(-38.574487053383,37.827410715392,14.9363867646851));
#42021=CARTESIAN_POINT('Ctrl Pts',(-38.6266179130002,37.8227707840955,14.949641118884));
#42022=CARTESIAN_POINT('Ctrl Pts',(-38.7343668418877,37.8059396772543,14.9986946717241));
#42023=CARTESIAN_POINT('Ctrl Pts',(-38.7864380337499,37.7926950432563,15.0377765425966));
#42024=CARTESIAN_POINT('Ctrl Pts',(-38.885076407075,37.7584001781814,15.1425998278601));
#42025=CARTESIAN_POINT('Ctrl Pts',(-38.9288507671719,37.7355961033814,15.2145406512318));
#42026=CARTESIAN_POINT('Ctrl Pts',(-38.9855092027929,37.6890702316704,15.3696270774554));
#42027=CARTESIAN_POINT('Ctrl Pts',(-38.9995659056513,37.6662504048046,15.4492226569908));
#42028=CARTESIAN_POINT('Ctrl Pts',(-38.9999967004912,37.6441366601067,15.5301365059714));
#42029=CARTESIAN_POINT('Ctrl Pts',(-39.,37.643798274373,15.5313755587675));
#42030=CARTESIAN_POINT('Ctrl Pts',(-39.,37.6434601185882,15.5326146734285));
#42031=CARTESIAN_POINT('Origin',(-38.5,40.3013122161429,14.5652356228366));
#42032=CARTESIAN_POINT('',(-39.,36.3630764119178,15.9986362310959));
#42033=CARTESIAN_POINT('',(-39.,37.9995447801587,15.4030104557381));
#42034=CARTESIAN_POINT('Origin',(-38.5,36.3630764119178,15.9986362310959));
#42035=CARTESIAN_POINT('Ctrl Pts',(-38.499976268987,36.1920824132574,15.528784071));
#42036=CARTESIAN_POINT('Ctrl Pts',(-39.0000141579952,36.1920742957822,15.5287617695291));
#42037=CARTESIAN_POINT('Ctrl Pts',(-38.9999999997996,36.3631080422587,15.9986397839424));
#42038=CARTESIAN_POINT('Ctrl Pts',(-38.5097935987872,36.1644071656834,15.5388572571144));
#42039=CARTESIAN_POINT('Ctrl Pts',(-39.0000137450654,36.1679944730221,15.5478735083829));
#42040=CARTESIAN_POINT('Ctrl Pts',(-38.9999999998035,36.3169823289421,16.0154292157321));
#42041=CARTESIAN_POINT('Ctrl Pts',(-38.5196108634531,36.1362370290697,15.5475699381323));
#42042=CARTESIAN_POINT('Ctrl Pts',(-39.0000133419967,36.1419138371004,15.5656989246035));
#42043=CARTESIAN_POINT('Ctrl Pts',(-38.9999999998075,36.2698666781457,16.0294976363005));
#42044=CARTESIAN_POINT('Ctrl Pts',(-38.5390736407832,36.0793995346958,15.5621222878223));
#42045=CARTESIAN_POINT('Ctrl Pts',(-39.0000125682431,36.0869060952579,15.5975660971732));
#42046=CARTESIAN_POINT('Ctrl Pts',(-38.9999999998153,36.1744793668348,16.0519471037778));
#42047=CARTESIAN_POINT('Ctrl Pts',(-38.5487190733747,36.0507326010709,15.5679624197071));
#42048=CARTESIAN_POINT('Ctrl Pts',(-39.0000121966607,36.0580101419523,15.6116879967721));
#42049=CARTESIAN_POINT('Ctrl Pts',(-38.9999999998191,36.1262084792976,16.0603291053491));
#42050=CARTESIAN_POINT('Ctrl Pts',(-38.5676730659644,35.9933927191952,15.5766710046091));
#42051=CARTESIAN_POINT('Ctrl Pts',(-39.0000114876801,35.9982390714978,15.6356400264069));
#42052=CARTESIAN_POINT('Ctrl Pts',(-38.9999999998267,36.0293379704017,16.0712648402057));
#42053=CARTESIAN_POINT('Ctrl Pts',(-38.5769815381232,35.9647200359621,15.5795394154795));
#42054=CARTESIAN_POINT('Ctrl Pts',(-39.0000111493512,35.967367881521,15.6455528228801));
#42055=CARTESIAN_POINT('Ctrl Pts',(-38.9999999998304,35.9807387962325,16.0738185200393));
#42056=CARTESIAN_POINT('Ctrl Pts',(-38.5951004176242,35.9078651416925,15.5822548730069));
#42057=CARTESIAN_POINT('Ctrl Pts',(-39.0000105080838,35.9045586256948,15.6607504618682));
#42058=CARTESIAN_POINT('Ctrl Pts',(-38.9999999998377,35.8840532497444,16.0730533413708));
#42059=CARTESIAN_POINT('Ctrl Pts',(-38.6039107409546,35.8796831935688,15.5821019053127));
#42060=CARTESIAN_POINT('Ctrl Pts',(-39.0000102042262,35.8726008933071,15.6661139213138));
#42061=CARTESIAN_POINT('Ctrl Pts',(-38.9999999998412,35.8359673238182,16.0697344836139));
#42062=CARTESIAN_POINT('Ctrl Pts',(-38.6208807544625,35.8242977617097,15.5787772351315));
#42063=CARTESIAN_POINT('Ctrl Pts',(-39.0000096326357,35.8085383701626,15.672043607951));
#42064=CARTESIAN_POINT('Ctrl Pts',(-38.999999999848,35.7411409298723,16.0572816469404));
#42065=CARTESIAN_POINT('Ctrl Pts',(-38.6290403659709,35.7970945340313,15.5756055463191));
#42066=CARTESIAN_POINT('Ctrl Pts',(-39.0000093640297,35.7763944628456,15.6726787655436));
#42067=CARTESIAN_POINT('Ctrl Pts',(-38.9999999998513,35.6944008994066,16.0481477228676));
#42068=CARTESIAN_POINT('Ctrl Pts',(-38.6445676535155,35.7441375911989,15.5662983324471));
#42069=CARTESIAN_POINT('Ctrl Pts',(-39.0000088633528,35.7128591951203,15.6691379903098));
#42070=CARTESIAN_POINT('Ctrl Pts',(-38.9999999998575,35.6030756547977,16.0242228639181));
#42071=CARTESIAN_POINT('Ctrl Pts',(-38.6519352576302,35.7183841206501,15.5601628487775));
#42072=CARTESIAN_POINT('Ctrl Pts',(-39.0000086304804,35.6814143002466,15.6650171583177));
#42073=CARTESIAN_POINT('Ctrl Pts',(-38.9999999998605,35.5584908615417,16.0094320368528));
#42074=CARTESIAN_POINT('Ctrl Pts',(-38.6657509411343,35.6687726400952,15.5450342622458));
#42075=CARTESIAN_POINT('Ctrl Pts',(-39.0000082014641,35.6201335587595,15.6520932108391));
#42076=CARTESIAN_POINT('Ctrl Pts',(-38.999999999866,35.4722481374437,15.9744494378102));
#42077=CARTESIAN_POINT('Ctrl Pts',(-38.6721989566158,35.6449148589008,15.5360412276563));
#42078=CARTESIAN_POINT('Ctrl Pts',(-39.000008004609,35.5902352214897,15.6433287035253));
#42079=CARTESIAN_POINT('Ctrl Pts',(-38.9999999998686,35.4305906033754,15.9542578244946));
#42080=CARTESIAN_POINT('Ctrl Pts',(-38.6840637962516,35.5995078834839,15.5153532356979));
#42081=CARTESIAN_POINT('Ctrl Pts',(-39.0000076476799,35.5328419212708,15.6213754182932));
#42082=CARTESIAN_POINT('Ctrl Pts',(-38.9999999998734,35.3509237627701,15.9088232405161));
#42083=CARTESIAN_POINT('Ctrl Pts',(-38.6894805656146,35.5779588982795,15.5036583721644));
#42084=CARTESIAN_POINT('Ctrl Pts',(-39.0000074869986,35.5052810328468,15.6082074902829));
#42085=CARTESIAN_POINT('Ctrl Pts',(-38.9999999998755,35.3129148219788,15.8835804763394));
#42086=CARTESIAN_POINT('Ctrl Pts',(-38.6991891029095,35.5375426665068,15.4777692022388));
#42087=CARTESIAN_POINT('Ctrl Pts',(-39.0000072023815,35.453278780813,15.5778206579272));
#42088=CARTESIAN_POINT('Ctrl Pts',(-38.9999999998794,35.2412033609684,15.8284806465574));
#42089=CARTESIAN_POINT('Ctrl Pts',(-38.7034808260903,35.5186756055761,15.4635750134849));
#42090=CARTESIAN_POINT('Ctrl Pts',(-39.000007077952,35.4287733420543,15.5606048558306));
#42091=CARTESIAN_POINT('Ctrl Pts',(-38.9999999998812,35.2075011692091,15.7986238314282));
#42092=CARTESIAN_POINT('Ctrl Pts',(-38.7108649420266,35.4839499382353,15.4329329506642));
#42093=CARTESIAN_POINT('Ctrl Pts',(-39.0000068657516,35.3835065226858,15.5225965334714));
#42094=CARTESIAN_POINT('Ctrl Pts',(-38.9999999998841,35.1449868299947,15.734812856048));
#42095=CARTESIAN_POINT('Ctrl Pts',(-38.7139573008052,35.4680914909596,15.4164852158956));
#42096=CARTESIAN_POINT('Ctrl Pts',(-39.0000067776074,35.3626877297703,15.5017905115115));
#42097=CARTESIAN_POINT('Ctrl Pts',(-38.9999999998854,35.1161749682031,15.7008589857377));
#42098=CARTESIAN_POINT('Ctrl Pts',(-38.7188891272861,35.4396576740633,15.3816208410028));
#42099=CARTESIAN_POINT('Ctrl Pts',(-39.000006637863,35.3253159030815,15.4571622621386));
#42100=CARTESIAN_POINT('Ctrl Pts',(-38.9999999998873,35.0639402373661,15.629441805129));
#42101=CARTESIAN_POINT('Ctrl Pts',(-38.7207285723286,35.4270824344453,15.3632043593695));
#42102=CARTESIAN_POINT('Ctrl Pts',(-39.0000065860148,35.3087162707208,15.4333120500278));
#42103=CARTESIAN_POINT('Ctrl Pts',(-38.9999999998881,35.0405176064801,15.5919788191372));
#42104=CARTESIAN_POINT('Ctrl Pts',(-38.7231227065882,35.405432808278,15.3247213622512));
#42105=CARTESIAN_POINT('Ctrl Pts',(-39.0000065187358,35.2801924397798,15.3832270666568));
#42106=CARTESIAN_POINT('Ctrl Pts',(-38.999999999889,34.9994669708968,15.5141920809946));
#42107=CARTESIAN_POINT('Ctrl Pts',(-38.7236773848157,35.3963585204766,15.3046550217128));
#42108=CARTESIAN_POINT('Ctrl Pts',(-39.0000065031849,35.2682357947743,15.3569527614816));
#42109=CARTESIAN_POINT('Ctrl Pts',(-38.9999999998892,34.9818391529727,15.47386868195));
#42110=CARTESIAN_POINT('Ctrl Pts',(-38.7234923684179,35.3818679549979,15.2632197487042));
#42111=CARTESIAN_POINT('Ctrl Pts',(-39.0000065083713,35.2492882925041,15.302706822063));
#42112=CARTESIAN_POINT('Ctrl Pts',(-38.9999999998892,34.9526834379338,15.3910593278306));
#42113=CARTESIAN_POINT('Ctrl Pts',(-38.7227526746417,35.376451743197,15.2418510046719));
#42114=CARTESIAN_POINT('Ctrl Pts',(-39.0000065291178,35.2422815479729,15.2746876798518));
#42115=CARTESIAN_POINT('Ctrl Pts',(-38.9999999998889,34.9411556731551,15.3485737487106));
#42116=CARTESIAN_POINT('Ctrl Pts',(-38.7199917114554,35.3693711473898,15.1981809212197));
#42117=CARTESIAN_POINT('Ctrl Pts',(-39.0000066067696,35.2333994155145,15.2176788928919));
#42118=CARTESIAN_POINT('Ctrl Pts',(-38.9999999998878,34.9243997338898,15.2621756907445));
#42119=CARTESIAN_POINT('Ctrl Pts',(-38.71797045472,35.3677067952793,15.1758797805686));
#42120=CARTESIAN_POINT('Ctrl Pts',(-39.0000066638135,35.2315260836188,15.1886378039953));
#42121=CARTESIAN_POINT('Ctrl Pts',(-38.999999999887,34.9191716350856,15.2182636044247));
#42122=CARTESIAN_POINT('Ctrl Pts',(-38.7126813554341,35.3681587728171,15.1307310487624));
#42123=CARTESIAN_POINT('Ctrl Pts',(-39.0000068139304,35.2329478863815,15.1303351175404));
#42124=CARTESIAN_POINT('Ctrl Pts',(-38.9999999998848,34.9151056148188,15.1297728960607));
#42125=CARTESIAN_POINT('Ctrl Pts',(-38.7094135371893,35.3702750997888,15.1078836633738));
#42126=CARTESIAN_POINT('Ctrl Pts',(-39.0000069072694,35.236263315592,15.1010224532041));
#42127=CARTESIAN_POINT('Ctrl Pts',(-38.9999999998835,34.9162677110207,15.0851946765572));
#42128=CARTESIAN_POINT('Ctrl Pts',(-38.7016878913306,35.3782518262364,15.0620380494563));
#42129=CARTESIAN_POINT('Ctrl Pts',(-39.0000071298392,35.2479693887033,15.0429328957708));
#42130=CARTESIAN_POINT('Ctrl Pts',(-38.9999999998804,34.9249620169377,14.9961436072836));
#42131=CARTESIAN_POINT('Ctrl Pts',(-38.6972300992734,35.3841121884087,15.0390400302111));
#42132=CARTESIAN_POINT('Ctrl Pts',(-39.0000072594605,35.2563977307434,15.014109705271));
#42133=CARTESIAN_POINT('Ctrl Pts',(-38.9999999998786,34.9324941858258,14.9516711632801));
#42134=CARTESIAN_POINT('Ctrl Pts',(-38.6872016890651,35.3994755467077,14.9932913687407));
#42135=CARTESIAN_POINT('Ctrl Pts',(-39.000007554437,35.2781058833073,14.9577442969424));
#42136=CARTESIAN_POINT('Ctrl Pts',(-38.9999999998746,34.9537982699429,14.8636017258914));
#42137=CARTESIAN_POINT('Ctrl Pts',(-38.6816311171518,35.4089784714142,14.9705409357234));
#42138=CARTESIAN_POINT('Ctrl Pts',(-39.0000077203025,35.2914388153182,14.930164811733));
#42139=CARTESIAN_POINT('Ctrl Pts',(-38.9999999998724,34.9675700863202,14.8200051345488));
#42140=CARTESIAN_POINT('Ctrl Pts',(-38.6694736006842,35.4314624433087,14.9256813847395));
#42141=CARTESIAN_POINT('Ctrl Pts',(-39.0000080875677,35.322603574829,14.8770030217846));
#42142=CARTESIAN_POINT('Ctrl Pts',(-38.9999999998675,35.0011150523726,14.734442324397));
#42143=CARTESIAN_POINT('Ctrl Pts',(-38.6628867122873,35.4444433860599,14.9035724722508));
#42144=CARTESIAN_POINT('Ctrl Pts',(-39.0000082895903,35.3405008359967,14.8513963837194));
#42145=CARTESIAN_POINT('Ctrl Pts',(-38.9999999998649,35.0208880466275,14.6924764968968));
#42146=CARTESIAN_POINT('Ctrl Pts',(-38.6488106161275,35.4736586580552,14.8603787974157));
#42147=CARTESIAN_POINT('Ctrl Pts',(-39.0000087288964,35.3803164068158,14.802848917274));
#42148=CARTESIAN_POINT('Ctrl Pts',(-38.9999999998592,35.0660930378355,14.6109019054829));
#42149=CARTESIAN_POINT('Ctrl Pts',(-38.6413214734913,35.489892851549,14.8392942331689));
#42150=CARTESIAN_POINT('Ctrl Pts',(-39.0000089669049,35.402308270487,14.7798999933156));
#42151=CARTESIAN_POINT('Ctrl Pts',(-38.9999999998562,35.0915248252762,14.5712935152036));
#42152=CARTESIAN_POINT('Ctrl Pts',(-38.6255705468163,35.5253335556531,14.7985143583617));
#42153=CARTESIAN_POINT('Ctrl Pts',(-39.0000094777876,35.4497155470534,14.7372695705394));
#42154=CARTESIAN_POINT('Ctrl Pts',(-38.9999999998499,35.1476070823755,14.4951196753651));
#42155=CARTESIAN_POINT('Ctrl Pts',(-38.6173088357458,35.5445399014998,14.778819234957));
#42156=CARTESIAN_POINT('Ctrl Pts',(-39.0000097514748,35.4752074583967,14.7175986525734));
#42157=CARTESIAN_POINT('Ctrl Pts',(-38.9999999998466,35.1782572919257,14.4585545750434));
#42158=CARTESIAN_POINT('Ctrl Pts',(-38.6001558291468,35.5855923740298,14.7411592921823));
#42159=CARTESIAN_POINT('Ctrl Pts',(-39.0000103331288,35.5289057182098,14.6820383202293));
#42160=CARTESIAN_POINT('Ctrl Pts',(-38.9999999998397,35.2442457072874,14.3891005019824));
#42161=CARTESIAN_POINT('Ctrl Pts',(-38.591264613141,35.607438309806,14.7231946456245));
#42162=CARTESIAN_POINT('Ctrl Pts',(-39.0000106419771,35.5571855083951,14.6661794507694));
#42163=CARTESIAN_POINT('Ctrl Pts',(-38.9999999998362,35.2795836068755,14.3562118477394));
#42164=CARTESIAN_POINT('Ctrl Pts',(-38.5730065552073,35.653391716595,14.6893067484556));
#42165=CARTESIAN_POINT('Ctrl Pts',(-39.000011293078,35.6156498660526,14.6386478824867));
#42166=CARTESIAN_POINT('Ctrl Pts',(-38.9999999998289,35.354335539997,14.2946801994281));
#42167=CARTESIAN_POINT('Ctrl Pts',(-38.5636397979342,35.6774989739494,14.6733836531619));
#42168=CARTESIAN_POINT('Ctrl Pts',(-39.0000116362538,35.6458982364807,14.6270255264977));
#42169=CARTESIAN_POINT('Ctrl Pts',(-38.9999999998251,35.3937492265869,14.2660374873015));
#42170=CARTESIAN_POINT('Ctrl Pts',(-38.544592851426,35.7275576179694,14.6438546054077));
#42171=CARTESIAN_POINT('Ctrl Pts',(-39.0000123547097,35.7074046291006,14.608238812539));
#42172=CARTESIAN_POINT('Ctrl Pts',(-38.9999999998175,35.4759702897537,14.2134937397502));
#42173=CARTESIAN_POINT('Ctrl Pts',(-38.5349127504493,35.7535087720731,14.630248787943));
#42174=CARTESIAN_POINT('Ctrl Pts',(-39.0000127309186,35.7387100140626,14.6011426709817));
#42175=CARTESIAN_POINT('Ctrl Pts',(-38.9999999998136,35.5187772848732,14.1895929445726));
#42176=CARTESIAN_POINT('Ctrl Pts',(-38.5154067371474,35.8068058703489,14.6055899230286));
#42177=CARTESIAN_POINT('Ctrl Pts',(-39.0000135135293,35.8013704615112,14.5915224275482));
#42178=CARTESIAN_POINT('Ctrl Pts',(-38.9999999998058,35.607043756353,14.1469469425535));
#42179=CARTESIAN_POINT('Ctrl Pts',(-38.5055809150832,35.8341515672782,14.594536987818));
#42180=CARTESIAN_POINT('Ctrl Pts',(-39.0000139208182,35.8327499432145,14.5890804612011));
#42181=CARTESIAN_POINT('Ctrl Pts',(-38.9999999998018,35.6525028236316,14.1282019299212));
#42182=CARTESIAN_POINT('Ctrl Pts',(-38.4859536041471,35.8897642585238,14.5751753147767));
#42183=CARTESIAN_POINT('Ctrl Pts',(-39.0000147628207,35.8945620836492,14.5886989627516));
#42184=CARTESIAN_POINT('Ctrl Pts',(-38.999999999794,35.7452863002563,14.0961921325892));
#42185=CARTESIAN_POINT('Ctrl Pts',(-38.4761522059002,35.9180309954215,14.5668666644427));
#42186=CARTESIAN_POINT('Ctrl Pts',(-39.0000151983183,35.9249907258467,14.5908493270198));
#42187=CARTESIAN_POINT('Ctrl Pts',(-38.99999999979,35.792610280322,14.0829274926165));
#42188=CARTESIAN_POINT('Ctrl Pts',(-38.4567434646595,35.974996318516,14.5531374737745));
#42189=CARTESIAN_POINT('Ctrl Pts',(-39.0000160927976,35.9839070296273,14.5993741709333));
#42190=CARTESIAN_POINT('Ctrl Pts',(-38.9999999997822,35.8883041425332,14.0621081867874));
#42191=CARTESIAN_POINT('Ctrl Pts',(-38.4471362110153,36.0036946418055,14.5477169947031));
#42192=CARTESIAN_POINT('Ctrl Pts',(-39.0000165523838,36.0123586893398,14.6058379828008));
#42193=CARTESIAN_POINT('Ctrl Pts',(-38.9999999997784,35.9366735829977,14.0545536137068));
#42194=CARTESIAN_POINT('Ctrl Pts',(-38.4282821195088,36.0610262084247,14.5398580520424));
#42195=CARTESIAN_POINT('Ctrl Pts',(-39.0000174895439,36.0663818685961,14.6224820332273));
#42196=CARTESIAN_POINT('Ctrl Pts',(-38.9999999997708,36.033620814048,14.0452853161319));
#42197=CARTESIAN_POINT('Ctrl Pts',(-38.4190353681169,36.089659188121,14.5374196225146));
#42198=CARTESIAN_POINT('Ctrl Pts',(-39.0000179674514,36.0918849124185,14.6327409659728));
#42199=CARTESIAN_POINT('Ctrl Pts',(-38.9999999997671,36.0821981585482,14.0435716310186));
#42200=CARTESIAN_POINT('Ctrl Pts',(-38.4010623993245,36.146364260849,14.5355670505141));
#42201=CARTESIAN_POINT('Ctrl Pts',(-39.0000189337675,36.1391959072527,14.6562284569052));
#42202=CARTESIAN_POINT('Ctrl Pts',(-38.9999999997599,36.1787200361203,14.0460148457356));
#42203=CARTESIAN_POINT('Ctrl Pts',(-38.392336263983,36.1744360942504,14.5361529144741));
#42204=CARTESIAN_POINT('Ctrl Pts',(-39.0000194221385,36.1609066386604,14.6695142627742));
#42205=CARTESIAN_POINT('Ctrl Pts',(-38.9999999997564,36.2266641267153,14.050171731156));
#42206=CARTESIAN_POINT('Ctrl Pts',(-38.3755556305667,36.2295327745401,14.5403388340369));
#42207=CARTESIAN_POINT('Ctrl Pts',(-39.0000203994702,36.2000284416751,14.6980809799109));
#42208=CARTESIAN_POINT('Ctrl Pts',(-38.9999999997497,36.3210892901581,14.0642841698589));
#42209=CARTESIAN_POINT('Ctrl Pts',(-38.367501208712,36.2565573703884,14.5439388685547));
#42210=CARTESIAN_POINT('Ctrl Pts',(-39.0000208879253,36.2173223481235,14.713387954275));
#42211=CARTESIAN_POINT('Ctrl Pts',(-38.9999999997465,36.3675699319872,14.0742396555811));
#42212=CARTESIAN_POINT('Ctrl Pts',(-38.3522034742026,36.3090915989522,14.5540908400596));
#42213=CARTESIAN_POINT('Ctrl Pts',(-39.0000218527547,36.2473143300469,14.7448410689014));
#42214=CARTESIAN_POINT('Ctrl Pts',(-38.9999999997403,36.4582633219484,14.0997769689501));
#42215=CARTESIAN_POINT('Ctrl Pts',(-38.3449602306372,36.3346009935599,14.5606427290728));
#42216=CARTESIAN_POINT('Ctrl Pts',(-39.0000223280847,36.2598891039266,14.7609760213118));
#42217=CARTESIAN_POINT('Ctrl Pts',(-38.9999999997374,36.5024756580302,14.1153586775199));
#42218=CARTESIAN_POINT('Ctrl Pts',(-38.3314102784294,36.3836630691935,14.5765850031111));
#42219=CARTESIAN_POINT('Ctrl Pts',(-39.0000232511576,36.2805499895026,14.7928435792589));
#42220=CARTESIAN_POINT('Ctrl Pts',(-38.999999999732,36.5878668276054,14.1518786846698));
#42221=CARTESIAN_POINT('Ctrl Pts',(-38.3251036306141,36.4072155290489,14.5859753143807));
#42222=CARTESIAN_POINT('Ctrl Pts',(-39.0000236973072,36.2885237503305,14.8085282882104));
#42223=CARTESIAN_POINT('Ctrl Pts',(-38.9999999997295,36.6290452750275,14.1728168152053));
#42224=CARTESIAN_POINT('Ctrl Pts',(-38.3135360779263,36.4519558604292,14.607431870355));
#42225=CARTESIAN_POINT('Ctrl Pts',(-39.0000245440666,36.3005570344607,14.8383222788334));
#42226=CARTESIAN_POINT('Ctrl Pts',(-38.9999999997248,36.7076555825882,14.2196871579371));
#42227=CARTESIAN_POINT('Ctrl Pts',(-38.3082751784691,36.4731437264623,14.6194981478164));
#42228=CARTESIAN_POINT('Ctrl Pts',(-39.0000249426352,36.3045330498124,14.852363427476));
#42229=CARTESIAN_POINT('Ctrl Pts',(-38.9999999997227,36.745087131247,14.2456191901704));
#42230=CARTESIAN_POINT('Ctrl Pts',(-38.3035827917596,36.4929654448321,14.6327976801015));
#42231=CARTESIAN_POINT('Ctrl Pts',(-39.0000253059108,36.3070470821327,14.865052826966));
#42232=CARTESIAN_POINT('Ctrl Pts',(-38.9999999997209,36.7803212016997,14.2738237060164));
#42233=CARTESIAN_POINT('',(-38.9808995532817,35.0987932250002,14.8625310449412));
#42234=CARTESIAN_POINT('',(-39.,36.7598993715046,14.257937916702));
#42235=CARTESIAN_POINT('Ctrl Pts',(-38.9808995442742,35.0987933242929,14.8625310222129));
#42236=CARTESIAN_POINT('Ctrl Pts',(-38.9767647379296,35.116349019978,14.8561412678243));
#42237=CARTESIAN_POINT('Ctrl Pts',(-38.9719271471844,35.1341609379785,14.8496306127704));
#42238=CARTESIAN_POINT('Ctrl Pts',(-38.9663672797599,35.1521966963304,14.8430315129897));
#42239=CARTESIAN_POINT('Ctrl Pts',(-38.9589054668452,35.176402211376,14.8341749622469));
#42240=CARTESIAN_POINT('Ctrl Pts',(-38.9501421609617,35.2010095699642,14.8251608525414));
#42241=CARTESIAN_POINT('Ctrl Pts',(-38.9400483440121,35.2259561953471,14.8160432642181));
#42242=CARTESIAN_POINT('Ctrl Pts',(-38.9308756360675,35.2486263220181,14.8077576993751));
#42243=CARTESIAN_POINT('Ctrl Pts',(-38.9206045220855,35.2715762307629,14.7993865402743));
#42244=CARTESIAN_POINT('Ctrl Pts',(-38.9092251669917,35.2947851487066,14.7909462729069));
#42245=CARTESIAN_POINT('Ctrl Pts',(-38.8978601608867,35.3179648009758,14.7825166484363));
#42246=CARTESIAN_POINT('Ctrl Pts',(-38.8853895090675,35.3414022162457,14.7740185519616));
#42247=CARTESIAN_POINT('Ctrl Pts',(-38.8718153038447,35.3651025799904,14.7654350181464));
#42248=CARTESIAN_POINT('Ctrl Pts',(-38.8629383335795,35.380601640214,14.7598217411112));
#42249=CARTESIAN_POINT('Ctrl Pts',(-38.8535896256093,35.3962138014434,14.7541712904865));
#42250=CARTESIAN_POINT('Ctrl Pts',(-38.8437734577105,35.411950727854,14.7484733033058));
#42251=CARTESIAN_POINT('Ctrl Pts',(-38.8299407627953,35.4341268055438,14.7404438442426));
#42252=CARTESIAN_POINT('Ctrl Pts',(-38.8151786393598,35.4565484470982,14.7323203526436));
#42253=CARTESIAN_POINT('Ctrl Pts',(-38.7995152955661,35.4792736089631,14.7240525449706));
#42254=CARTESIAN_POINT('Ctrl Pts',(-38.7936375981427,35.4878012660903,14.7209500355386));
#42255=CARTESIAN_POINT('Ctrl Pts',(-38.7876332216565,35.4963721011908,14.7178271266627));
#42256=CARTESIAN_POINT('Ctrl Pts',(-38.7815045885274,35.5049909053511,14.7146810901815));
#42257=CARTESIAN_POINT('Ctrl Pts',(-38.7795162123981,35.5077871935437,14.7136603888752));
#42258=CARTESIAN_POINT('Ctrl Pts',(-38.7771942222782,35.5110389942361,14.7124711412873));
#42259=CARTESIAN_POINT('Ctrl Pts',(-38.7751079474046,35.5139398250466,14.711413790367));
#42260=CARTESIAN_POINT('Ctrl Pts',(-38.7736879354939,35.5159142601288,14.7106941100797));
#42261=CARTESIAN_POINT('Ctrl Pts',(-38.7723780994354,35.517726392354,14.7100348526341));
#42262=CARTESIAN_POINT('Ctrl Pts',(-38.7713664599503,35.5191246936257,14.7095250845846));
#42263=CARTESIAN_POINT('Ctrl Pts',(-38.7591460919159,35.5360158454794,14.7033672059448));
#42264=CARTESIAN_POINT('Ctrl Pts',(-38.7459652690169,35.5537552475421,14.6968911730339));
#42265=CARTESIAN_POINT('Ctrl Pts',(-38.7317687459757,35.5723139069922,14.6901294727658));
#42266=CARTESIAN_POINT('Ctrl Pts',(-38.7232003627024,35.5835150797543,14.6860484143751));
#42267=CARTESIAN_POINT('Ctrl Pts',(-38.7142624901345,35.5950148086917,14.6818626484207));
#42268=CARTESIAN_POINT('Ctrl Pts',(-38.7049499967065,35.6068100037668,14.6775738863478));
#42269=CARTESIAN_POINT('Ctrl Pts',(-38.6914598459875,35.6238966154841,14.6713611521097));
#42270=CARTESIAN_POINT('Ctrl Pts',(-38.6771815904704,35.6416017827983,14.6649326897865));
#42271=CARTESIAN_POINT('Ctrl Pts',(-38.6621289822079,35.6599303559949,14.6582736496514));
#42272=CARTESIAN_POINT('Ctrl Pts',(-38.6529092037587,35.6711566751295,14.6541949628445));
#42273=CARTESIAN_POINT('Ctrl Pts',(-38.6433996162985,35.6826172647426,14.6500294703126));
#42274=CARTESIAN_POINT('Ctrl Pts',(-38.6336114709703,35.6943188541858,14.6457727995193));
#42275=CARTESIAN_POINT('Ctrl Pts',(-38.6307797553414,35.6977041302108,14.6445413424038));
#42276=CARTESIAN_POINT('Ctrl Pts',(-38.6279247708707,35.7011096036338,14.6433022574605));
#42277=CARTESIAN_POINT('Ctrl Pts',(-38.6250469058212,35.7045355081267,14.642055390223));
#42278=CARTESIAN_POINT('Ctrl Pts',(-38.6231484010499,35.7067955501765,14.6412328417856));
#42279=CARTESIAN_POINT('Ctrl Pts',(-38.6219577178143,35.70821201593,14.6407173324049));
#42280=CARTESIAN_POINT('Ctrl Pts',(-38.6193199827135,35.7113415310103,14.639578540854));
#42281=CARTESIAN_POINT('Ctrl Pts',(-38.6093963463712,35.7231153325473,14.6352942011503));
#42282=CARTESIAN_POINT('Ctrl Pts',(-38.600451520594,35.733924467879,14.6312927832749));
#42283=CARTESIAN_POINT('Ctrl Pts',(-38.5925313692603,35.7438150067674,14.6275978327402));
#42284=CARTESIAN_POINT('Ctrl Pts',(-38.5839175250442,35.7545718165312,14.6235792569642));
#42285=CARTESIAN_POINT('Ctrl Pts',(-38.5765151121156,35.7642419688015,14.6199244835375));
#42286=CARTESIAN_POINT('Ctrl Pts',(-38.5703367971687,35.7728453441612,14.6166607138016));
#42287=CARTESIAN_POINT('Ctrl Pts',(-38.5689416731234,35.7747880706065,14.6159237226194));
#42288=CARTESIAN_POINT('Ctrl Pts',(-38.5676088151344,35.7766762616162,14.6152066150956));
#42289=CARTESIAN_POINT('Ctrl Pts',(-38.5663381283992,35.7785099169919,14.6145095958068));
#42290=CARTESIAN_POINT('Ctrl Pts',(-38.5600210194182,35.7876257757806,14.6110444248188));
#42291=CARTESIAN_POINT('Ctrl Pts',(-38.5552431665246,35.7953964841108,14.6080782285374));
#42292=CARTESIAN_POINT('Ctrl Pts',(-38.5519704510026,35.8017991138177,14.6056167712994));
#42293=CARTESIAN_POINT('Ctrl Pts',(-38.5508098883644,35.8040695992216,14.6047438951552));
#42294=CARTESIAN_POINT('Ctrl Pts',(-38.5498383139863,35.8061677486475,14.603934201354));
#42295=CARTESIAN_POINT('Ctrl Pts',(-38.5490533846631,35.808091706157,14.603187009408));
#42296=CARTESIAN_POINT('Ctrl Pts',(-38.5486074101368,35.8091848441171,14.6027624761865));
#42297=CARTESIAN_POINT('Ctrl Pts',(-38.5485269918336,35.8092779875322,14.602729607332));
#42298=CARTESIAN_POINT('Ctrl Pts',(-38.5479678306013,35.8109932342015,14.602055342206));
#42299=CARTESIAN_POINT('Ctrl Pts',(-38.5479228048346,35.8111313523181,14.6020010478406));
#42300=CARTESIAN_POINT('Ctrl Pts',(-38.5478746740126,35.8112799988974,14.6019426209443));
#42301=CARTESIAN_POINT('Ctrl Pts',(-38.5478229968322,35.8114405509189,14.6018795418018));
#42302=CARTESIAN_POINT('Ctrl Pts',(-38.5449835603478,35.8202621867631,14.5984136170561));
#42303=CARTESIAN_POINT('Ctrl Pts',(-38.5433058289746,35.8292618452946,14.5949231012738));
#42304=CARTESIAN_POINT('Ctrl Pts',(-38.5427752974539,35.8384513754963,14.5914640211649));
#42305=CARTESIAN_POINT('Ctrl Pts',(-38.5423420551633,35.8459557234158,14.5886392695128));
#42306=CARTESIAN_POINT('Ctrl Pts',(-38.5426741373589,35.8535859788554,14.5858347064009));
#42307=CARTESIAN_POINT('Ctrl Pts',(-38.5437703713166,35.8613377512468,14.5830585045683));
#42308=CARTESIAN_POINT('Ctrl Pts',(-38.5451107571661,35.8708159889432,14.579663990445));
#42309=CARTESIAN_POINT('Ctrl Pts',(-38.5475935941593,35.8804757210054,14.5763134226948));
#42310=CARTESIAN_POINT('Ctrl Pts',(-38.5512260819329,35.890297003835,14.5729770455601));
#42311=CARTESIAN_POINT('Ctrl Pts',(-38.5547558391688,35.8998405305566,14.569735024646));
#42312=CARTESIAN_POINT('Ctrl Pts',(-38.5593717925242,35.909535959512,14.5665064366129));
#42313=CARTESIAN_POINT('Ctrl Pts',(-38.5650829120781,35.9193616198279,14.5632169645182));
#42314=CARTESIAN_POINT('Ctrl Pts',(-38.5658016677034,35.9205981984981,14.5628029779872));
#42315=CARTESIAN_POINT('Ctrl Pts',(-38.5671656761932,35.922871397621,14.5620409226064));
#42316=CARTESIAN_POINT('Ctrl Pts',(-38.567290740915,35.9230774137073,14.5619718110317));
#42317=CARTESIAN_POINT('Ctrl Pts',(-38.5682304871265,35.924625434875,14.561452501193));
#42318=CARTESIAN_POINT('Ctrl Pts',(-38.570461396946,35.9276549380703,14.5603840529096));
#42319=CARTESIAN_POINT('Ctrl Pts',(-38.5739282260106,35.9321429471728,14.5587879606264));
#42320=CARTESIAN_POINT('Ctrl Pts',(-38.5766210025586,35.9356289008882,14.5575482341246));
#42321=CARTESIAN_POINT('Ctrl Pts',(-38.58006088657,35.9399948247985,14.5559900602808));
#42322=CARTESIAN_POINT('Ctrl Pts',(-38.5842425702584,35.9452337123745,14.5541188046349));
#42323=CARTESIAN_POINT('Ctrl Pts',(-38.5902071488439,35.9527062423353,14.5514497239044));
#42324=CARTESIAN_POINT('Ctrl Pts',(-38.5976806527857,35.9619529111913,14.5481458695105));
#42325=CARTESIAN_POINT('Ctrl Pts',(-38.6066862825953,35.9729747446293,14.5441966642552));
#42326=CARTESIAN_POINT('Ctrl Pts',(-38.6144225315189,35.9824430049148,14.5408041158659));
#42327=CARTESIAN_POINT('Ctrl Pts',(-38.6232918494035,35.9932206612145,14.5369352592365));
#42328=CARTESIAN_POINT('Ctrl Pts',(-38.6333101538699,36.0053367931859,14.5325548376229));
#42329=CARTESIAN_POINT('Ctrl Pts',(-38.634953979492,36.0073248349989,14.5318360883267));
#42330=CARTESIAN_POINT('Ctrl Pts',(-38.6366286984273,36.009348995464,14.5311034993255));
#42331=CARTESIAN_POINT('Ctrl Pts',(-38.6383343167614,36.0114095103981,14.5303568361756));
#42332=CARTESIAN_POINT('Ctrl Pts',(-38.6403446495301,36.0138381432345,14.5294767791504));
#42333=CARTESIAN_POINT('Ctrl Pts',(-38.6430226780081,36.0170741020974,14.5283029774242));
#42334=CARTESIAN_POINT('Ctrl Pts',(-38.6450720281982,36.0195454051338,14.5274039547414));
#42335=CARTESIAN_POINT('Ctrl Pts',(-38.6459862124317,36.0206478161728,14.5270029142719));
#42336=CARTESIAN_POINT('Ctrl Pts',(-38.6467744829065,36.0215977660742,14.5266569179816));
#42337=CARTESIAN_POINT('Ctrl Pts',(-38.6473190777943,36.022254636695,14.5264177462369));
#42338=CARTESIAN_POINT('Ctrl Pts',(-38.6495834782687,36.0249858744988,14.5254232811321));
#42339=CARTESIAN_POINT('Ctrl Pts',(-38.6518336507024,36.0277062660658,14.5244327799928));
#42340=CARTESIAN_POINT('Ctrl Pts',(-38.6540694260694,36.0304158360253,14.5234462803024));
#42341=CARTESIAN_POINT('Ctrl Pts',(-38.667469166842,36.0466551843962,14.5175338615874));
#42342=CARTESIAN_POINT('Ctrl Pts',(-38.6803477610403,36.0625071583347,14.5117657668271));
#42343=CARTESIAN_POINT('Ctrl Pts',(-38.6926983696478,36.0779736920762,14.5061390254219));
#42344=CARTESIAN_POINT('Ctrl Pts',(-38.6975666324403,36.0840701649816,14.5039211221026));
#42345=CARTESIAN_POINT('Ctrl Pts',(-38.7023533966268,36.0901065401151,14.5017250552718));
#42346=CARTESIAN_POINT('Ctrl Pts',(-38.7070601793549,36.0960821953089,14.4995499061324));
#42347=CARTESIAN_POINT('Ctrl Pts',(-38.7110458741123,36.1011423688826,14.4977079939341));
#42348=CARTESIAN_POINT('Ctrl Pts',(-38.7146256566631,36.1057104847595,14.4960433701251));
#42349=CARTESIAN_POINT('Ctrl Pts',(-38.7184672819383,36.1106486014496,14.4942458820026));
#42350=CARTESIAN_POINT('Ctrl Pts',(-38.7205521762747,36.1133285743211,14.4932703644708));
#42351=CARTESIAN_POINT('Ctrl Pts',(-38.7227146244336,36.1161180496071,14.4922552996327));
#42352=CARTESIAN_POINT('Ctrl Pts',(-38.7250639334399,36.1191596590394,14.4911476720038));
#42353=CARTESIAN_POINT('Ctrl Pts',(-38.725134081171,36.1192504780845,14.4911145994855));
#42354=CARTESIAN_POINT('Ctrl Pts',(-38.7252043956138,36.1193415222387,14.4910814442195));
#42355=CARTESIAN_POINT('Ctrl Pts',(-38.7252748796988,36.1194327953631,14.4910482047526));
#42356=CARTESIAN_POINT('Ctrl Pts',(-38.7391992330306,36.1374640890149,14.4844816431961));
#42357=CARTESIAN_POINT('Ctrl Pts',(-38.7525852683106,36.1552020757998,14.4780033780421));
#42358=CARTESIAN_POINT('Ctrl Pts',(-38.7653792735979,36.1726723554198,14.4716284835979));
#42359=CARTESIAN_POINT('Ctrl Pts',(-38.7756440047546,36.1866888982854,14.4665138556019));
#42360=CARTESIAN_POINT('Ctrl Pts',(-38.785528790763,36.2005323432467,14.4614663378914));
#42361=CARTESIAN_POINT('Ctrl Pts',(-38.7950264447249,36.214203378581,14.45649124442));
#42362=CARTESIAN_POINT('Ctrl Pts',(-38.8079002855734,36.2327341372116,14.4497476252259));
#42363=CARTESIAN_POINT('Ctrl Pts',(-38.8200619297502,36.2509486437685,14.4431385491419));
#42364=CARTESIAN_POINT('Ctrl Pts',(-38.8315338136742,36.268839344416,14.4366484694331));
#42365=CARTESIAN_POINT('Ctrl Pts',(-38.8395762860386,36.2813817887514,14.4320985378747));
#42366=CARTESIAN_POINT('Ctrl Pts',(-38.8472807935542,36.2937644106038,14.4276064034222));
#42367=CARTESIAN_POINT('Ctrl Pts',(-38.8546637596816,36.3059802738794,14.4231551143583));
#42368=CARTESIAN_POINT('Ctrl Pts',(-38.8563276050559,36.3087332741307,14.4221519597196));
#42369=CARTESIAN_POINT('Ctrl Pts',(-38.857677559501,36.3109841441762,14.4213330235564));
#42370=CARTESIAN_POINT('Ctrl Pts',(-38.8593427195925,36.3137774238209,14.4203146899841));
#42371=CARTESIAN_POINT('Ctrl Pts',(-38.8600372362967,36.3149424645772,14.4198899562424));
#42372=CARTESIAN_POINT('Ctrl Pts',(-38.8607863197798,36.3162022978644,14.4194305167246));
#42373=CARTESIAN_POINT('Ctrl Pts',(-38.8616341123971,36.3176350562414,14.4189085099844));
#42374=CARTESIAN_POINT('Ctrl Pts',(-38.8620353308256,36.3183131101108,14.4186614699421));
#42375=CARTESIAN_POINT('Ctrl Pts',(-38.8624357283147,36.318990958965,14.4184144479097));
#42376=CARTESIAN_POINT('Ctrl Pts',(-38.8628353023743,36.3196686044897,14.4181674451164));
#42377=CARTESIAN_POINT('Ctrl Pts',(-38.8747207051118,36.339825293296,14.4108203023155));
#42378=CARTESIAN_POINT('Ctrl Pts',(-38.8858742499577,36.3598051766581,14.4034902073188));
#42379=CARTESIAN_POINT('Ctrl Pts',(-38.8962515739831,36.3796455861763,14.3962075160251));
#42380=CARTESIAN_POINT('Ctrl Pts',(-38.9073388406698,36.4008433353228,14.3884265948192));
#42381=CARTESIAN_POINT('Ctrl Pts',(-38.9175408702454,36.4218807760399,14.3807005684331));
#42382=CARTESIAN_POINT('Ctrl Pts',(-38.9268423622115,36.4427703158319,14.3730516163559));
#42383=CARTESIAN_POINT('Ctrl Pts',(-38.9383225424702,36.4685528121461,14.3636110503739));
#42384=CARTESIAN_POINT('Ctrl Pts',(-38.9484320971274,36.494109926635,14.354288799014));
#42385=CARTESIAN_POINT('Ctrl Pts',(-38.9571837010109,36.5194437401331,14.345086390156));
#42386=CARTESIAN_POINT('Ctrl Pts',(-38.9661019465223,36.5452599415428,14.3357087557723));
#42387=CARTESIAN_POINT('Ctrl Pts',(-38.9736123558276,36.5708426756316,14.3264533231054));
#42388=CARTESIAN_POINT('Ctrl Pts',(-38.9797348916918,36.5961815584403,14.3172922402715));
#42389=CARTESIAN_POINT('Ctrl Pts',(-38.9864757782507,36.6240795631782,14.3072059261181));
#42390=CARTESIAN_POINT('Ctrl Pts',(-38.9915356867791,36.6516828688677,14.2972307775915));
#42391=CARTESIAN_POINT('Ctrl Pts',(-38.9949170488217,36.6789767320434,14.287338916061));
#42392=CARTESIAN_POINT('Ctrl Pts',(-38.9978813548361,36.7029041795484,14.27866711332));
#42393=CARTESIAN_POINT('Ctrl Pts',(-38.9995545419852,36.7265941813416,14.2700581931021));
#42394=CARTESIAN_POINT('Ctrl Pts',(-38.9999223536161,36.7500252217522,14.261531615527));
#42395=CARTESIAN_POINT('Ctrl Pts',(-38.9999741020041,36.7533217966002,14.2603319888489));
#42396=CARTESIAN_POINT('Ctrl Pts',(-38.9999999996542,36.7566132194275,14.2591340723458));
#42397=CARTESIAN_POINT('Ctrl Pts',(-39.,36.7598994028097,14.2579380027121));
#42398=CARTESIAN_POINT('',(-38.7236068457623,35.3906903574536,15.2883751610654));
#42399=CARTESIAN_POINT('Ctrl Pts',(-38.7236068979077,35.3906894271638,15.2883726211906));
#42400=CARTESIAN_POINT('Ctrl Pts',(-38.7246641593601,35.3897885482407,15.2874430895349));
#42401=CARTESIAN_POINT('Ctrl Pts',(-38.7250262636518,35.389481991673,15.2871302835944));
#42402=CARTESIAN_POINT('Ctrl Pts',(-38.7514788663481,35.3668699550198,15.2636753415614));
#42403=CARTESIAN_POINT('Ctrl Pts',(-38.8224426853319,35.3062619186145,15.2008982931996));
#42404=CARTESIAN_POINT('Ctrl Pts',(-38.9289695382785,35.1867017408949,15.0281412453392));
#42405=CARTESIAN_POINT('Ctrl Pts',(-38.9617634006977,35.140307300847,14.9486149885387));
#42406=CARTESIAN_POINT('Ctrl Pts',(-38.9808995805048,35.0987931708383,14.8625310771125));
#42407=CARTESIAN_POINT('Origin',(-38.5,36.0210562685922,15.0589436103097));
#42408=CARTESIAN_POINT('Origin',(-38.9999999999999,36.0210586628155,15.058945287974));
#42409=CARTESIAN_POINT('Origin',(-40.02360679775,35.3051952361797,15.3194957179792));
#42410=CARTESIAN_POINT('',(-39.,35.2608289688876,15.335643718679));
#42411=CARTESIAN_POINT('Origin',(-38.5,40.3013122161429,14.5652356228366));
#42412=CARTESIAN_POINT('',(-39.,44.2395480203679,13.1318350145773));
#42413=CARTESIAN_POINT('Origin',(-38.5,44.2395480203679,13.1318350145773));
#42414=CARTESIAN_POINT('',(-39.,44.9997753200724,12.8551349062082));
#42415=CARTESIAN_POINT('Ctrl Pts',(-38.4957681230772,43.7146667366125,11.7267038890717));
#42416=CARTESIAN_POINT('Ctrl Pts',(-39.,43.716193831966,11.7306891746095));
#42417=CARTESIAN_POINT('Ctrl Pts',(-39.,43.5357661657807,11.2598241647595));
#42418=CARTESIAN_POINT('Ctrl Pts',(-38.5104887561845,43.755952609823,11.7110172571947));
#42419=CARTESIAN_POINT('Ctrl Pts',(-39.0000000000001,43.7513673016004,11.7015437407619));
#42420=CARTESIAN_POINT('Ctrl Pts',(-39.,43.6045049054216,11.2334846192326));
#42421=CARTESIAN_POINT('Ctrl Pts',(-38.5252362294721,43.7984294432773,11.6983678551985));
#42422=CARTESIAN_POINT('Ctrl Pts',(-39.,43.7911361284587,11.675132616616));
#42423=CARTESIAN_POINT('Ctrl Pts',(-39.,43.675600497817,11.2132286937603));
#42424=CARTESIAN_POINT('Ctrl Pts',(-38.5542137101166,43.8841199255624,11.6796331382235));
#42425=CARTESIAN_POINT('Ctrl Pts',(-39.,43.8764894776903,11.6313912291823));
#42426=CARTESIAN_POINT('Ctrl Pts',(-39.,43.819752056524,11.1856680867503));
#42427=CARTESIAN_POINT('Ctrl Pts',(-38.5684428387846,43.9273310021072,11.6735484618443));
#42428=CARTESIAN_POINT('Ctrl Pts',(-39.,43.9219957425488,11.6137920684096));
#42429=CARTESIAN_POINT('Ctrl Pts',(-39.,43.8928036600594,11.1783643871917));
#42430=CARTESIAN_POINT('Ctrl Pts',(-38.5958298929736,44.0128086259304,11.668180454929));
#42431=CARTESIAN_POINT('Ctrl Pts',(-39.,44.0157276825881,11.5890560462835));
#42432=CARTESIAN_POINT('Ctrl Pts',(-39.,44.0380247156817,11.1769935191695));
#42433=CARTESIAN_POINT('Ctrl Pts',(-38.6089871338095,44.0550730387334,11.6688972641344));
#42434=CARTESIAN_POINT('Ctrl Pts',(-39.,44.0640020110278,11.5816534952057));
#42435=CARTESIAN_POINT('Ctrl Pts',(-39.,44.1101905494472,11.1829263849608));
#42436=CARTESIAN_POINT('Ctrl Pts',(-38.6337186415401,44.1370136007802,11.6771046639679));
#42437=CARTESIAN_POINT('Ctrl Pts',(-39.,44.1601223386003,11.5778169161264));
#42438=CARTESIAN_POINT('Ctrl Pts',(-39.,44.2508333864788,11.2077985694355));
#42439=CARTESIAN_POINT('Ctrl Pts',(-38.6452922898437,44.1766877029697,11.6845950548096));
#42440=CARTESIAN_POINT('Ctrl Pts',(-39.,44.2081128144266,11.5811665269809));
#42441=CARTESIAN_POINT('Ctrl Pts',(-39.,44.3193068873798,11.2267372688822));
#42442=CARTESIAN_POINT('Ctrl Pts',(-38.6664064032844,44.251904572198,11.7060586330073));
#42443=CARTESIAN_POINT('Ctrl Pts',(-39.,44.3006750969489,11.598562111161));
#42444=CARTESIAN_POINT('Ctrl Pts',(-39.,44.4499018395266,11.2768852145754));
#42445=CARTESIAN_POINT('Ctrl Pts',(-38.6759463402347,44.2874454600443,11.7200312889306));
#42446=CARTESIAN_POINT('Ctrl Pts',(-39.,44.3454481642641,11.6124687294269));
#42447=CARTESIAN_POINT('Ctrl Pts',(-39.,44.5120200408709,11.3080932130564));
#42448=CARTESIAN_POINT('Ctrl Pts',(-38.6926218940153,44.3530134983602,11.753916307973));
#42449=CARTESIAN_POINT('Ctrl Pts',(-39.,44.428901013663,11.6500339784918));
#42450=CARTESIAN_POINT('Ctrl Pts',(-39.,44.6274882090049,11.3815666424003));
#42451=CARTESIAN_POINT('Ctrl Pts',(-38.6997570937363,44.3830390111172,11.7738278290408));
#42452=CARTESIAN_POINT('Ctrl Pts',(-39.,44.4677973706649,11.6736416532639));
#42453=CARTESIAN_POINT('Ctrl Pts',(-39.,44.6808353045031,11.4238302464452));
#42454=CARTESIAN_POINT('Ctrl Pts',(-38.7113455437151,44.4364083250159,11.8188165042088));
#42455=CARTESIAN_POINT('Ctrl Pts',(-39.,44.5372576216464,11.7291039591263));
#42456=CARTESIAN_POINT('Ctrl Pts',(-39.,44.7766860774448,11.5177717429142));
#42457=CARTESIAN_POINT('Ctrl Pts',(-38.7157985041745,44.4597507937971,11.8438925388205));
#42458=CARTESIAN_POINT('Ctrl Pts',(-39.,44.5680147948136,11.760993098812));
#42459=CARTESIAN_POINT('Ctrl Pts',(-39.,44.8191873730925,11.5694473011972));
#42460=CARTESIAN_POINT('Ctrl Pts',(-38.7218491523116,44.4988458933973,11.8982352839493));
#42461=CARTESIAN_POINT('Ctrl Pts',(-39.,44.619483259022,11.8310677445932));
#42462=CARTESIAN_POINT('Ctrl Pts',(-39.,44.8916930695162,11.6802034356976));
#42463=CARTESIAN_POINT('Ctrl Pts',(-38.7234466887105,44.514597548933,11.9275006414011));
#42464=CARTESIAN_POINT('Ctrl Pts',(-39.,44.6403325524953,11.869358484827));
#42465=CARTESIAN_POINT('Ctrl Pts',(-39.,44.9216956695369,11.7392812613325));
#42466=CARTESIAN_POINT('Ctrl Pts',(-38.7237242128408,44.5378980584001,11.9890841057603));
#42467=CARTESIAN_POINT('Ctrl Pts',(-39.,44.6708633890369,11.9499591289122));
#42468=CARTESIAN_POINT('Ctrl Pts',(-39.,44.9680365091014,11.8625446758251));
#42469=CARTESIAN_POINT('Ctrl Pts',(-38.7224041936341,44.5454463318916,12.0214006787586));
#42470=CARTESIAN_POINT('Ctrl Pts',(-39.,44.6806049880233,11.9924212363057));
#42471=CARTESIAN_POINT('Ctrl Pts',(-39.,44.9843735979966,11.9267272040495));
#42472=CARTESIAN_POINT('Ctrl Pts',(-38.7168978002672,44.5520461127452,12.0878299294229));
#42473=CARTESIAN_POINT('Ctrl Pts',(-39.,44.6884337596283,12.0788836807004));
#42474=CARTESIAN_POINT('Ctrl Pts',(-39.,45.0027473637736,12.0577041266596));
#42475=CARTESIAN_POINT('Ctrl Pts',(-38.7127115637761,44.5510974570559,12.1219409519436));
#42476=CARTESIAN_POINT('Ctrl Pts',(-39.,44.6864915499809,12.1230533895049));
#42477=CARTESIAN_POINT('Ctrl Pts',(-39.,45.0047835844392,12.1244952683306));
#42478=CARTESIAN_POINT('Ctrl Pts',(-38.7016354079073,44.5407398453553,12.1906326060098));
#42479=CARTESIAN_POINT('Ctrl Pts',(-39.,44.6711238494387,12.210373277459));
#42480=CARTESIAN_POINT('Ctrl Pts',(-39.,44.9944757119117,12.2580919452284));
#42481=CARTESIAN_POINT('Ctrl Pts',(-38.6947457655101,44.5313311502024,12.2252115255115));
#42482=CARTESIAN_POINT('Ctrl Pts',(-39.,44.6575804147925,12.2536773253778));
#42483=CARTESIAN_POINT('Ctrl Pts',(-39.,44.982131874978,12.3248941610696));
#42484=CARTESIAN_POINT('Ctrl Pts',(-38.6785306211109,44.5044189374293,12.2934942107537));
#42485=CARTESIAN_POINT('Ctrl Pts',(-39.,44.6198413622739,12.3367624214714));
#42486=CARTESIAN_POINT('Ctrl Pts',(-39.,44.9435432418528,12.4559149547927));
#42487=CARTESIAN_POINT('Ctrl Pts',(-38.6692055246944,44.486916094711,12.3271962742984));
#42488=CARTESIAN_POINT('Ctrl Pts',(-39.,44.5954530285034,12.3766497399001));
#42489=CARTESIAN_POINT('Ctrl Pts',(-39.,44.9172994052938,12.5201302750391));
#42490=CARTESIAN_POINT('Ctrl Pts',(-38.6484820298786,44.4444958642473,12.3924145118707));
#42491=CARTESIAN_POINT('Ctrl Pts',(-39.,44.537496750665,12.4505883516032));
#42492=CARTESIAN_POINT('Ctrl Pts',(-39.,44.851930741321,12.6434797252075));
#42493=CARTESIAN_POINT('Ctrl Pts',(-38.6370841498941,44.4195795393625,12.4239290601754));
#42494=CARTESIAN_POINT('Ctrl Pts',(-39.,44.5036878365839,12.4846706149496));
#42495=CARTESIAN_POINT('Ctrl Pts',(-39.,44.8128075406341,12.7026107858961));
#42496=CARTESIAN_POINT('Ctrl Pts',(-38.612658278484,44.36330096768,12.4835465298239));
#42497=CARTESIAN_POINT('Ctrl Pts',(-39.,44.4289638773543,12.5450197756454));
#42498=CARTESIAN_POINT('Ctrl Pts',(-39.,44.7232010636579,12.8134917740948));
#42499=CARTESIAN_POINT('Ctrl Pts',(-38.5996308980214,44.3319401302231,12.511647965753));
#42500=CARTESIAN_POINT('Ctrl Pts',(-39.,44.3877977020642,12.5712233390459));
#42501=CARTESIAN_POINT('Ctrl Pts',(-39.,44.6727200187587,12.8652389406661));
#42502=CARTESIAN_POINT('Ctrl Pts',(-38.5724526116315,44.2639918355033,12.5633461379396));
#42503=CARTESIAN_POINT('Ctrl Pts',(-39.,44.3009663522788,12.6143232592351));
#42504=CARTESIAN_POINT('Ctrl Pts',(-39.,44.5623605667487,12.9593392527306));
#42505=CARTESIAN_POINT('Ctrl Pts',(-38.5583023852123,44.2274060787236,12.5869415874867));
#42506=CARTESIAN_POINT('Ctrl Pts',(-39.,44.2550869417833,12.6310565225753));
#42507=CARTESIAN_POINT('Ctrl Pts',(-39.,44.5024849092967,13.0016900538045));
#42508=CARTESIAN_POINT('Ctrl Pts',(-38.5294286852375,44.1504305117409,12.6287098869748));
#42509=CARTESIAN_POINT('Ctrl Pts',(-39.,44.1618651290856,12.6543799114258));
#42510=CARTESIAN_POINT('Ctrl Pts',(-39.,44.3756644133745,13.0753500839617));
#42511=CARTESIAN_POINT('Ctrl Pts',(-38.5147061045232,44.1100431097314,12.6468815233693));
#42512=CARTESIAN_POINT('Ctrl Pts',(-39.,44.1143989355615,12.660720422544));
#42513=CARTESIAN_POINT('Ctrl Pts',(-39.,44.3087235418349,13.1066571838109));
#42514=CARTESIAN_POINT('Ctrl Pts',(-38.4999828339055,44.0685379488058,12.6619887044612));
#42515=CARTESIAN_POINT('Ctrl Pts',(-39.,44.0685320774541,12.661972573055));
#42516=CARTESIAN_POINT('Ctrl Pts',(-39.,44.2395480203679,13.1318350145773));
#42517=CARTESIAN_POINT('',(-39.,43.5555078199205,11.2524499908864));
#42518=CARTESIAN_POINT('Ctrl Pts',(-38.5439382020836,43.7465865791704,11.7129332004299));
#42519=CARTESIAN_POINT('Ctrl Pts',(-38.5627108024178,43.7454905093906,11.7115697786477));
#42520=CARTESIAN_POINT('Ctrl Pts',(-38.5818394836764,43.7440439920326,11.7091586579251));
#42521=CARTESIAN_POINT('Ctrl Pts',(-38.6011103776041,43.7422011778166,11.7055948274057));
#42522=CARTESIAN_POINT('Ctrl Pts',(-38.6202864790502,43.7403674283036,11.7020485271752));
#42523=CARTESIAN_POINT('Ctrl Pts',(-38.639602741903,43.7381411164017,11.6973604045454));
#42524=CARTESIAN_POINT('Ctrl Pts',(-38.6588261733529,43.7354930847464,11.6914710015509));
#42525=CARTESIAN_POINT('Ctrl Pts',(-38.6780496048027,43.7328450530911,11.6855815985564));
#42526=CARTESIAN_POINT('Ctrl Pts',(-38.6971794210865,43.729775197568,11.6784906291453));
#42527=CARTESIAN_POINT('Ctrl Pts',(-38.7159711064253,43.7262723900725,11.6701881703371));
#42528=CARTESIAN_POINT('Ctrl Pts',(-38.7336425594366,43.7229783961093,11.6623806475916));
#42529=CARTESIAN_POINT('Ctrl Pts',(-38.7510179611022,43.7192998641312,11.6535001143584));
#42530=CARTESIAN_POINT('Ctrl Pts',(-38.7678799008077,43.7152435234236,11.6435908256301));
#42531=CARTESIAN_POINT('Ctrl Pts',(-38.7846868277303,43.7112004166971,11.6337138663705));
#42532=CARTESIAN_POINT('Ctrl Pts',(-38.8009828486583,43.7067820402673,11.6228150671742));
#42533=CARTESIAN_POINT('Ctrl Pts',(-38.8165686297444,43.702011877337,11.6109844626736));
#42534=CARTESIAN_POINT('Ctrl Pts',(-38.8321255085374,43.6972505602032,11.5991757968617));
#42535=CARTESIAN_POINT('Ctrl Pts',(-38.8469740663892,43.6921389056185,11.5864391783255));
#42536=CARTESIAN_POINT('Ctrl Pts',(-38.860943297614,43.6867153771627,11.5729056582632));
#42537=CARTESIAN_POINT('Ctrl Pts',(-38.8638049456601,43.6856043475463,11.5701332672403));
#42538=CARTESIAN_POINT('Ctrl Pts',(-38.8666298041761,43.6844802762301,11.5673275608693));
#42539=CARTESIAN_POINT('Ctrl Pts',(-38.8694165842623,43.6833435624567,11.5644898541878));
#42540=CARTESIAN_POINT('Ctrl Pts',(-38.8830703511397,43.6777742586767,11.5505865735923));
#42541=CARTESIAN_POINT('Ctrl Pts',(-38.8958018953305,43.6719012781054,11.5359181594009));
#42542=CARTESIAN_POINT('Ctrl Pts',(-38.907487219436,43.6657813607992,11.5206573183788));
#42543=CARTESIAN_POINT('Ctrl Pts',(-38.919187229744,43.6596537519353,11.5053772974177));
#42544=CARTESIAN_POINT('Ctrl Pts',(-38.9298380208449,43.6532788417078,11.4895040641895));
#42545=CARTESIAN_POINT('Ctrl Pts',(-38.9393615495029,43.646721800628,11.4732335514217));
#42546=CARTESIAN_POINT('Ctrl Pts',(-38.9489282990728,43.6401350015348,11.4568891977047));
#42547=CARTESIAN_POINT('Ctrl Pts',(-38.957357351642,43.6333646919751,11.440144712106));
#42548=CARTESIAN_POINT('Ctrl Pts',(-38.964620598952,43.6264811843718,11.4232103854808));
#42549=CARTESIAN_POINT('Ctrl Pts',(-38.9660145216253,43.6251601392647,11.4199604421934));
#42550=CARTESIAN_POINT('Ctrl Pts',(-38.967365659868,43.6238349302522,11.4167035214325));
#42551=CARTESIAN_POINT('Ctrl Pts',(-38.9686740335233,43.6225060587887,11.413441121867));
#42552=CARTESIAN_POINT('Ctrl Pts',(-38.9760247879083,43.6150401428423,11.3951121851654));
#42553=CARTESIAN_POINT('Ctrl Pts',(-38.9820201538307,43.6074604423925,11.3766151341195));
#42554=CARTESIAN_POINT('Ctrl Pts',(-38.9867094178029,43.5998495614506,11.3581761811704));
#42555=CARTESIAN_POINT('Ctrl Pts',(-38.9914661093554,43.5921292425905,11.3394720919461));
#42556=CARTESIAN_POINT('Ctrl Pts',(-38.9948792009387,43.5843770901683,11.3208284707058));
#42557=CARTESIAN_POINT('Ctrl Pts',(-38.9970499532579,43.5766720279274,11.3024613860455));
#42558=CARTESIAN_POINT('Ctrl Pts',(-38.9990538941774,43.5695590609736,11.2855057194795));
#42559=CARTESIAN_POINT('Ctrl Pts',(-38.9999999917031,43.5624862507436,11.2687857923547));
#42560=CARTESIAN_POINT('Ctrl Pts',(-39.,43.5555078257317,11.2524499884039));
#42561=CARTESIAN_POINT('Origin',(-39.,43.8975113829057,12.1921486462674));
#42562=CARTESIAN_POINT('Origin',(-38.5,39.6172719294915,12.6858503812648));
#42563=CARTESIAN_POINT('',(-39.,39.6172719294915,12.6858503812648));
#42564=CARTESIAN_POINT('Ctrl Pts',(-38.5,42.3431727827618,14.3786118971418));
#42565=CARTESIAN_POINT('Ctrl Pts',(-39.,42.3431727827618,14.3786118971418));
#42566=CARTESIAN_POINT('Ctrl Pts',(-39.,42.8199489247508,14.5292256761601));
#42567=CARTESIAN_POINT('Ctrl Pts',(-38.5000000151735,42.3235389145373,14.4407639791455));
#42568=CARTESIAN_POINT('Ctrl Pts',(-38.9808235694178,42.3295231330866,14.4218206445454));
#42569=CARTESIAN_POINT('Ctrl Pts',(-39.,42.7834708241676,14.5798104778281));
#42570=CARTESIAN_POINT('Ctrl Pts',(-38.5044132464344,42.3017127589935,14.5014168958436));
#42571=CARTESIAN_POINT('Ctrl Pts',(-38.9652824568155,42.3135424787352,14.4689442264536));
#42572=CARTESIAN_POINT('Ctrl Pts',(-39.0022066208479,42.7452111602329,14.6295830574807));
#42573=CARTESIAN_POINT('Ctrl Pts',(-38.5201182104299,42.2538679845483,14.6200333912239));
#42574=CARTESIAN_POINT('Ctrl Pts',(-38.9423369615246,42.2764879943097,14.5669878025861));
#42575=CARTESIAN_POINT('Ctrl Pts',(-39.0100591075842,42.6651957614355,14.7276861607036));
#42576=CARTESIAN_POINT('Ctrl Pts',(-38.5314246665614,42.227847908903,14.6779967191923));
#42577=CARTESIAN_POINT('Ctrl Pts',(-38.9346328775752,42.2555724552384,14.6178337748267));
#42578=CARTESIAN_POINT('Ctrl Pts',(-39.0157123318515,42.6234394464224,14.7760157468895));
#42579=CARTESIAN_POINT('Ctrl Pts',(-38.552651089205,42.1857348662789,14.7630638104245));
#42580=CARTESIAN_POINT('Ctrl Pts',(-38.9285245106868,42.2199024964374,14.6960761304899));
#42581=CARTESIAN_POINT('Ctrl Pts',(-39.0263255453171,42.5581752806135,14.8475077052381));
#42582=CARTESIAN_POINT('Ctrl Pts',(-38.5604419961988,42.1711826366542,14.7911056783425));
#42583=CARTESIAN_POINT('Ctrl Pts',(-38.9273730528816,42.2074674656466,14.7221761912045));
#42584=CARTESIAN_POINT('Ctrl Pts',(-39.0302209975595,42.5359817233398,14.8711708137875));
#42585=CARTESIAN_POINT('Ctrl Pts',(-38.5731186427038,42.1485842461019,14.832708622288));
#42586=CARTESIAN_POINT('Ctrl Pts',(-38.926916498768,42.1877378091319,14.7616810012592));
#42587=CARTESIAN_POINT('Ctrl Pts',(-39.0365593216219,42.5020273470754,14.9064206387115));
#42588=CARTESIAN_POINT('Ctrl Pts',(-38.5775094223885,42.1409230674214,14.846499586987));
#42589=CARTESIAN_POINT('Ctrl Pts',(-38.9269719591409,42.1810223729242,14.7748341780693));
#42590=CARTESIAN_POINT('Ctrl Pts',(-39.0387547109623,42.4905985146427,14.9181297528723));
#42591=CARTESIAN_POINT('Ctrl Pts',(-38.5866095911227,42.1253437576203,14.8739295117817));
#42592=CARTESIAN_POINT('Ctrl Pts',(-38.9274916449468,42.1672574095469,14.8011897647693));
#42593=CARTESIAN_POINT('Ctrl Pts',(-39.0433047957933,42.4675180576399,14.9414671669666));
#42594=CARTESIAN_POINT('Ctrl Pts',(-38.5913209172013,42.1174228143287,14.8875723296809));
#42595=CARTESIAN_POINT('Ctrl Pts',(-38.9279536908748,42.1602065716068,14.8143979542777));
#42596=CARTESIAN_POINT('Ctrl Pts',(-39.0456604581885,42.4558625514204,14.9530988371724));
#42597=CARTESIAN_POINT('Ctrl Pts',(-38.6155177819721,42.0773849632758,14.9550630836894));
#42598=CARTESIAN_POINT('Ctrl Pts',(-38.9311989887487,42.1246877033306,14.8794706017327));
#42599=CARTESIAN_POINT('Ctrl Pts',(-39.0577588926346,42.3973293691335,15.0107605238563));
#42600=CARTESIAN_POINT('Ctrl Pts',(-38.6370023785226,42.0438120311917,15.0070352766296));
#42601=CARTESIAN_POINT('Ctrl Pts',(-38.9368284508843,42.0937684062961,14.9316236792503));
#42602=CARTESIAN_POINT('Ctrl Pts',(-39.0685011882335,42.3494478230898,15.0555491513583));
#42603=CARTESIAN_POINT('Ctrl Pts',(-38.6834063423229,41.9737282317394,15.1073632756364));
#42604=CARTESIAN_POINT('Ctrl Pts',(-38.9532556851885,42.0277155354844,15.0338788517455));
#42605=CARTESIAN_POINT('Ctrl Pts',(-39.0917031721878,42.2515616380507,15.1427428606496));
#42606=CARTESIAN_POINT('Ctrl Pts',(-38.7083300695819,41.9372167755023,15.1557169775274));
#42607=CARTESIAN_POINT('Ctrl Pts',(-38.963949218556,41.9925965667856,15.0841722205039));
#42608=CARTESIAN_POINT('Ctrl Pts',(-39.1041650341826,42.2015570290535,15.1851464699237));
#42609=CARTESIAN_POINT('Ctrl Pts',(-38.7610633626364,41.8613333331087,15.2490754374726));
#42610=CARTESIAN_POINT('Ctrl Pts',(-38.9895991647772,41.9183569021626,15.1822592900656));
#42611=CARTESIAN_POINT('Ctrl Pts',(-39.1305316819265,42.0993810792371,15.2677629211416));
#42612=CARTESIAN_POINT('Ctrl Pts',(-38.7888752933149,41.8219610687487,15.2940790871008));
#42613=CARTESIAN_POINT('Ctrl Pts',(-39.0044992158228,41.8792245556372,15.2302347536082));
#42614=CARTESIAN_POINT('Ctrl Pts',(-39.1444376463372,42.0472098181495,15.3079749806063));
#42615=CARTESIAN_POINT('Ctrl Pts',(-38.8324659250877,41.7607737749083,15.3591954444135));
#42616=CARTESIAN_POINT('Ctrl Pts',(-39.0296343641317,41.8173594933725,15.3004082221224));
#42617=CARTESIAN_POINT('Ctrl Pts',(-39.166232962704,41.967271130407,15.3667436422317));
#42618=CARTESIAN_POINT('Ctrl Pts',(-38.8473093173328,41.7400227844779,15.3805019886511));
#42619=CARTESIAN_POINT('Ctrl Pts',(-39.0384151694295,41.7963453190696,15.3233737884774));
#42620=CARTESIAN_POINT('Ctrl Pts',(-39.1736546585605,41.940344345471,15.3860744919038));
#42621=CARTESIAN_POINT('Ctrl Pts',(-38.870015379526,41.7083619831663,15.4118730882152));
#42622=CARTESIAN_POINT('Ctrl Pts',(-39.0522271030963,41.7640415062336,15.357359413503));
#42623=CARTESIAN_POINT('Ctrl Pts',(-39.1850076898159,41.8995237784172,15.4146908074332));
#42624=CARTESIAN_POINT('Ctrl Pts',(-38.8776576124367,41.6977193058703,15.4222319640262));
#42625=CARTESIAN_POINT('Ctrl Pts',(-39.0569232021872,41.7531759506236,15.3685790901832));
#42626=CARTESIAN_POINT('Ctrl Pts',(-39.1888288061772,41.8858451739218,15.4241662290078));
#42627=CARTESIAN_POINT('Ctrl Pts',(-38.8930849110735,41.6762552578125,15.4427545725828));
#42628=CARTESIAN_POINT('Ctrl Pts',(-39.066511133906,41.7312068662022,15.3908393217828));
#42629=CARTESIAN_POINT('Ctrl Pts',(-39.1965424555779,41.8583426536247,15.4429914483156));
#42630=CARTESIAN_POINT('Ctrl Pts',(-38.9008746912715,41.66542735373,15.4529240043621));
#42631=CARTESIAN_POINT('Ctrl Pts',(-39.0714060895731,41.7200956440113,15.4018887144115));
#42632=CARTESIAN_POINT('Ctrl Pts',(-39.2004373455104,41.8445104908778,15.4523465539704));
#42633=CARTESIAN_POINT('Ctrl Pts',(-38.9400159979964,41.611054246107,15.5030904749622));
#42634=CARTESIAN_POINT('Ctrl Pts',(-39.0961105529348,41.664486384419,15.4561555034708));
#42635=CARTESIAN_POINT('Ctrl Pts',(-39.2200079994996,41.7752545712226,15.4986298218549));
#42636=CARTESIAN_POINT('Ctrl Pts',(-38.9720506860609,41.566657227979,15.5411994956368));
#42637=CARTESIAN_POINT('Ctrl Pts',(-39.1172505217694,41.6183487327083,15.4979423053299));
#42638=CARTESIAN_POINT('Ctrl Pts',(-39.2360252362306,41.7193499540182,15.5342207819066));
#42639=CARTESIAN_POINT('Ctrl Pts',(-39.004664367461,41.5213832040514,15.5774321632787));
#42640=CARTESIAN_POINT('Ctrl Pts',(-39.139478538059,41.5707159497276,15.537951312608));
#42641=CARTESIAN_POINT('Ctrl Pts',(-39.2523321837305,41.6629039474018,15.5684921983703));
#42642=CARTESIAN_POINT('',(-39.0936699647309,42.2443432359162,15.1482528495184));
#42643=CARTESIAN_POINT('Ctrl Pts',(-39.,41.5278577779161,15.5722329179818));
#42644=CARTESIAN_POINT('Ctrl Pts',(-39.,41.555365582337,15.5500682176439));
#42645=CARTESIAN_POINT('Ctrl Pts',(-39.0025061283031,41.6103743139319,15.5062349506866));
#42646=CARTESIAN_POINT('Ctrl Pts',(-39.011910467653,41.6938875962409,15.4431191586721));
#42647=CARTESIAN_POINT('Ctrl Pts',(-39.0251886793738,41.7791789788017,15.383441099477));
#42648=CARTESIAN_POINT('Ctrl Pts',(-39.0355006548008,41.8375977236174,15.3462767602701));
#42649=CARTESIAN_POINT('Ctrl Pts',(-39.0460180996933,41.8969209424409,15.3105044475851));
#42650=CARTESIAN_POINT('Ctrl Pts',(-39.0513795683656,41.9270342259527,15.2933134663306));
#42651=CARTESIAN_POINT('Ctrl Pts',(-39.0592129369566,41.9729415209881,15.2685857940176));
#42652=CARTESIAN_POINT('Ctrl Pts',(-39.0617895723962,41.9883665401829,15.2605193084358));
#42653=CARTESIAN_POINT('Ctrl Pts',(-39.0668167987977,42.0194688332009,15.2447375200145));
#42654=CARTESIAN_POINT('Ctrl Pts',(-39.0692638673594,42.0351249489564,15.2370331001163));
#42655=CARTESIAN_POINT('Ctrl Pts',(-39.0763170763895,42.0823578826811,15.2144966152885));
#42656=CARTESIAN_POINT('Ctrl Pts',(-39.0806383134429,42.1142224339666,15.2002291333683));
#42657=CARTESIAN_POINT('Ctrl Pts',(-39.086250870079,42.1626004871079,15.1799187978017));
#42658=CARTESIAN_POINT('Ctrl Pts',(-39.0888401552868,42.1869348076306,15.1700364166254));
#42659=CARTESIAN_POINT('Ctrl Pts',(-39.0914175141258,42.2155837611224,15.1589770191016));
#42660=CARTESIAN_POINT('Ctrl Pts',(-39.0924201592736,42.227917997062,15.15433750161));
#42661=CARTESIAN_POINT('Ctrl Pts',(-39.0929039086555,42.2340945254209,15.1520344157921));
#42662=CARTESIAN_POINT('Ctrl Pts',(-39.0930625659985,42.236159807516,15.1512676840144));
#42663=CARTESIAN_POINT('Ctrl Pts',(-39.0933714042916,42.2402499173753,15.1497569469128));
#42664=CARTESIAN_POINT('Ctrl Pts',(-39.0935224084833,42.2422960384328,15.1490037844944));
#42665=CARTESIAN_POINT('Ctrl Pts',(-39.0936699647319,42.2443432359167,15.1482528495195));
#42666=CARTESIAN_POINT('Ctrl Pts',(-39.0936699647319,42.2443432359167,15.1482528495195));
#42667=CARTESIAN_POINT('Ctrl Pts',(-39.0805958020047,42.2975092731202,15.1026169640987));
#42668=CARTESIAN_POINT('Ctrl Pts',(-39.0684075521881,42.3495683432789,15.0555700511839));
#42669=CARTESIAN_POINT('Ctrl Pts',(-39.0545825391346,42.413189511403,14.994849343675));
#42670=CARTESIAN_POINT('Ctrl Pts',(-39.0518885060209,42.4258409923919,14.9826093594223));
#42671=CARTESIAN_POINT('Ctrl Pts',(-39.0466519979229,42.4509962153533,14.9579329492598));
#42672=CARTESIAN_POINT('Ctrl Pts',(-39.0441085920868,42.4635046891825,14.945491722837));
#42673=CARTESIAN_POINT('Ctrl Pts',(-39.0367291513417,42.5007669083855,14.9079038797878));
#42674=CARTESIAN_POINT('Ctrl Pts',(-39.0321447527579,42.5252490627375,14.8825025364275));
#42675=CARTESIAN_POINT('Ctrl Pts',(-39.0195339780508,42.5975848409282,14.805227756089));
#42676=CARTESIAN_POINT('Ctrl Pts',(-39.0126341194485,42.6443310367265,14.752288032587));
#42677=CARTESIAN_POINT('Ctrl Pts',(-39.0053154013728,42.7120528329345,14.6705075551378));
#42678=CARTESIAN_POINT('Ctrl Pts',(-39.0033844025761,42.7342264354137,14.6428512503343));
#42679=CARTESIAN_POINT('Ctrl Pts',(-39.0007271289037,42.7777317502299,14.586691290421));
#42680=CARTESIAN_POINT('Ctrl Pts',(-38.9999999999987,42.799063541628,14.5581877930259));
#42681=CARTESIAN_POINT('Ctrl Pts',(-39.,42.8199489247508,14.5292256761601));
#42682=CARTESIAN_POINT('Origin',(-29.,20.7255401693197,-2.54750793782168));
#42683=CARTESIAN_POINT('Origin',(-29.,39.9592920728172,13.6255430020507));
#42684=CARTESIAN_POINT('Origin',(-29.,39.9592920728172,13.6255430020507));
#42685=CARTESIAN_POINT('Ctrl Pts',(-39.,38.3487778137292,16.1565988728829));
#42686=CARTESIAN_POINT('Ctrl Pts',(-39.,38.6171968569105,15.7347562277442));
#42687=CARTESIAN_POINT('Ctrl Pts',(-38.5,38.6171968569105,15.7347562277442));
#42688=CARTESIAN_POINT('Ctrl Pts',(-39.,38.4092369437272,16.1719014080264));
#42689=CARTESIAN_POINT('Ctrl Pts',(-38.980823569418,38.6554271426563,15.7590822228985));
#42690=CARTESIAN_POINT('Ctrl Pts',(-38.5000000151735,38.6721878607891,15.7697470775665));
#42691=CARTESIAN_POINT('Ctrl Pts',(-39.0022066208479,38.4705387441827,16.1854365781618));
#42692=CARTESIAN_POINT('Ctrl Pts',(-38.9652824568155,38.6979594886938,15.7849088143478));
#42693=CARTESIAN_POINT('Ctrl Pts',(-38.5044132464344,38.7278946093028,15.8021803250113));
#42694=CARTESIAN_POINT('Ctrl Pts',(-39.0100591075842,38.5948935550188,16.2091550083072));
#42695=CARTESIAN_POINT('Ctrl Pts',(-38.9423369615246,38.7893660665278,15.8361963875558));
#42696=CARTESIAN_POINT('Ctrl Pts',(-38.5201182104299,38.8407910464338,15.862291803958));
#42697=CARTESIAN_POINT('Ctrl Pts',(-39.0157123318516,38.6579464072813,16.2193371773267));
#42698=CARTESIAN_POINT('Ctrl Pts',(-38.9346328775752,38.8380714599669,15.8617024126807));
#42699=CARTESIAN_POINT('Ctrl Pts',(-38.5314246665614,38.8979816898257,15.889968907025));
#42700=CARTESIAN_POINT('Ctrl Pts',(-39.0263255453171,38.7538958038527,16.2321521976088));
#42701=CARTESIAN_POINT('Ctrl Pts',(-38.9285245106867,38.9156894504658,15.8987113268976));
#42702=CARTESIAN_POINT('Ctrl Pts',(-38.552651089205,38.9849222243469,15.9280643375507));
#42703=CARTESIAN_POINT('Ctrl Pts',(-39.0302209975595,38.7861074080575,16.2360134467896));
#42704=CARTESIAN_POINT('Ctrl Pts',(-38.9273730528816,38.9419920323425,15.9107120496548));
#42705=CARTESIAN_POINT('Ctrl Pts',(-38.5604419961988,39.014094844236,15.9401916617479));
#42706=CARTESIAN_POINT('Ctrl Pts',(-39.0365593216218,38.8347761200192,16.2411909269361));
#42707=CARTESIAN_POINT('Ctrl Pts',(-38.926916498768,38.9824990285064,15.9282925111225));
#42708=CARTESIAN_POINT('Ctrl Pts',(-38.5731186427039,39.0581480726366,15.9575354003289));
#42709=CARTESIAN_POINT('Ctrl Pts',(-39.0387547109622,38.8510575870985,16.2428143168919));
#42710=CARTESIAN_POINT('Ctrl Pts',(-38.9269719591409,38.996098050178,15.9340518299393));
#42711=CARTESIAN_POINT('Ctrl Pts',(-38.5775094223885,39.0728815372267,15.9631753814703));
#42712=CARTESIAN_POINT('Ctrl Pts',(-39.0433047957933,38.8837392435521,16.2458559814884));
#42713=CARTESIAN_POINT('Ctrl Pts',(-38.9274916449469,39.0235836684596,15.9453934327693));
#42714=CARTESIAN_POINT('Ctrl Pts',(-38.5866095911227,39.1024475967202,15.974173735627));
#42715=CARTESIAN_POINT('Ctrl Pts',(-39.0456604581885,38.9001445728115,16.2472743428312));
#42716=CARTESIAN_POINT('Ctrl Pts',(-38.9279536908748,39.0374749842454,15.9509793016801));
#42717=CARTESIAN_POINT('Ctrl Pts',(-38.5913209172013,39.1172848256198,15.9795332562622));
#42718=CARTESIAN_POINT('Ctrl Pts',(-39.0577588926345,38.9820478095945,16.2538213531667));
#42719=CARTESIAN_POINT('Ctrl Pts',(-38.9311989887487,39.1065119074279,15.9779967532242));
#42720=CARTESIAN_POINT('Ctrl Pts',(-38.6155177819721,39.1913378193784,16.0054983387571));
#42721=CARTESIAN_POINT('Ctrl Pts',(-39.0685011882335,39.0475167766825,16.2573537678501));
#42722=CARTESIAN_POINT('Ctrl Pts',(-38.9368284508843,39.1637208151416,15.9980737874138));
#42723=CARTESIAN_POINT('Ctrl Pts',(-38.6370023785226,39.2504632591108,16.023731083591));
#42724=CARTESIAN_POINT('Ctrl Pts',(-39.0917031721878,39.1785489807647,16.2612279974249));
#42725=CARTESIAN_POINT('Ctrl Pts',(-38.9532556851884,39.2800486076852,16.0339478271421));
#42726=CARTESIAN_POINT('Ctrl Pts',(-38.6834063423228,39.3686401589,16.0555377917917));
#42727=CARTESIAN_POINT('Ctrl Pts',(-39.1041650341826,39.2441112482649,16.2615687035868));
#42728=CARTESIAN_POINT('Ctrl Pts',(-38.9639492185558,39.3392792527924,16.0499007448607));
#42729=CARTESIAN_POINT('Ctrl Pts',(-38.7083300695817,39.4276907175188,16.0691097647488));
#42730=CARTESIAN_POINT('Ctrl Pts',(-39.1305316819266,39.3754873980411,16.2591791424027));
#42731=CARTESIAN_POINT('Ctrl Pts',(-38.9895991647774,39.4591992883204,16.077319462873));
#42732=CARTESIAN_POINT('Ctrl Pts',(-38.7610633626365,39.5458304682011,16.091849557657));
#42733=CARTESIAN_POINT('Ctrl Pts',(-39.1444376463372,39.4413007162717,16.2564483268932));
#42734=CARTESIAN_POINT('Ctrl Pts',(-39.0044992158227,39.5200144384565,16.0889170126415));
#42735=CARTESIAN_POINT('Ctrl Pts',(-38.788875293315,39.6049191608988,16.1010163496788));
#42736=CARTESIAN_POINT('Ctrl Pts',(-39.1662329627039,39.5403130713378,16.2500841355454));
#42737=CARTESIAN_POINT('Ctrl Pts',(-39.0296343641317,39.6125124617173,16.1029069127551));
#42738=CARTESIAN_POINT('Ctrl Pts',(-38.8324659250876,39.6936473350033,16.1115679390035));
#42739=CARTESIAN_POINT('Ctrl Pts',(-39.1736546585605,39.573365815963,16.2475842217919));
#42740=CARTESIAN_POINT('Ctrl Pts',(-39.0384151694294,39.6433722346712,16.1069919063746));
#42741=CARTESIAN_POINT('Ctrl Pts',(-38.8473093173327,39.7232390985529,16.1145512192814));
#42742=CARTESIAN_POINT('Ctrl Pts',(-39.1850076898159,39.6230303975766,16.2432666365631));
#42743=CARTESIAN_POINT('Ctrl Pts',(-39.0522271030963,39.6899639296596,16.1122619149349));
#42744=CARTESIAN_POINT('Ctrl Pts',(-38.870015379526,39.7676576335643,16.1182317049812));
#42745=CARTESIAN_POINT('Ctrl Pts',(-39.1888288061771,39.6395995001247,16.2417327931191));
#42746=CARTESIAN_POINT('Ctrl Pts',(-39.0569232021872,39.7054992973109,16.1138724413908));
#42747=CARTESIAN_POINT('Ctrl Pts',(-38.8776576124367,39.7824689543885,16.1193260831334));
#42748=CARTESIAN_POINT('Ctrl Pts',(-39.1965424555779,39.6727682706908,16.2384754684783));
#42749=CARTESIAN_POINT('Ctrl Pts',(-39.0665111339059,39.7366371934134,16.1168033128481));
#42750=CARTESIAN_POINT('Ctrl Pts',(-38.8930849110734,39.8121030476287,16.1212504892313));
#42751=CARTESIAN_POINT('Ctrl Pts',(-39.2004373455104,39.6893776681015,16.236750752351));
#42752=CARTESIAN_POINT('Ctrl Pts',(-39.0714060895731,39.7522512961052,16.1181254827183));
#42753=CARTESIAN_POINT('Ctrl Pts',(-38.9008746912715,39.8269344881269,16.1220806833524));
#42754=CARTESIAN_POINT('Ctrl Pts',(-39.2200079994996,39.7721810916385,16.2276889454715));
#42755=CARTESIAN_POINT('Ctrl Pts',(-39.0961105529348,39.8297324800265,16.1239513118732));
#42756=CARTESIAN_POINT('Ctrl Pts',(-38.9400159979962,39.9008330908001,16.1255600695062));
#42757=CARTESIAN_POINT('Ctrl Pts',(-39.2360252362298,39.8378839411281,16.2190184073814));
#42758=CARTESIAN_POINT('Ctrl Pts',(-39.1172505217682,39.8919360102205,16.1263051483739));
#42759=CARTESIAN_POINT('Ctrl Pts',(-38.9720506860607,39.9593391861364,16.126215419867));
#42760=CARTESIAN_POINT('Ctrl Pts',(-39.2523321837305,39.9031533327047,16.2089890418516));
#42761=CARTESIAN_POINT('Ctrl Pts',(-39.1394785380589,39.9541421330884,16.1263360633587));
#42762=CARTESIAN_POINT('Ctrl Pts',(-39.0046643674609,40.0173110104085,16.1248696719522));
#42763=CARTESIAN_POINT('',(-39.0936699647309,39.1876203501825,16.2608089943257));
#42764=CARTESIAN_POINT('Ctrl Pts',(-39.0936699647318,39.187620350183,16.2608089943268));
#42765=CARTESIAN_POINT('Ctrl Pts',(-39.0935222711613,39.1896732804381,16.2600676057615));
#42766=CARTESIAN_POINT('Ctrl Pts',(-39.0933711189158,39.1917268197941,16.2593286228811));
#42767=CARTESIAN_POINT('Ctrl Pts',(-39.0932165432533,39.1937809620199,16.2585920211916));
#42768=CARTESIAN_POINT('Ctrl Pts',(-39.0930619675907,39.1958351042458,16.2578554195021));
#42769=CARTESIAN_POINT('Ctrl Pts',(-39.092903426222,39.1979084188697,16.2571158289587));
#42770=CARTESIAN_POINT('Ctrl Pts',(-39.0927422452511,39.1999780775388,16.2563808711829));
#42771=CARTESIAN_POINT('Ctrl Pts',(-39.0924198833093,39.2041173948769,16.2549109556315));
#42772=CARTESIAN_POINT('Ctrl Pts',(-39.0920858400397,39.2082587537971,16.2534536804623));
#42773=CARTESIAN_POINT('Ctrl Pts',(-39.0917405120476,39.2124021988525,16.2520090278225));
#42774=CARTESIAN_POINT('Ctrl Pts',(-39.0913590487798,39.2169792158534,16.2504132060838));
#42775=CARTESIAN_POINT('Ctrl Pts',(-39.0909638345645,39.2215588916347,16.2488327920271));
#42776=CARTESIAN_POINT('Ctrl Pts',(-39.0905552639041,39.2261405355601,16.2472677592867));
#42777=CARTESIAN_POINT('Ctrl Pts',(-39.0902240994565,39.2298541589952,16.24599923158));
#42778=CARTESIAN_POINT('Ctrl Pts',(-39.0898844110932,39.2335707729552,16.2447408596389));
#42779=CARTESIAN_POINT('Ctrl Pts',(-39.0895361673382,39.2372882900436,16.2434925788529));
#42780=CARTESIAN_POINT('Ctrl Pts',(-39.0886541452664,39.2467039136605,16.240330968087));
#42781=CARTESIAN_POINT('Ctrl Pts',(-39.0877185869797,39.2561331757771,16.2372343338719));
#42782=CARTESIAN_POINT('Ctrl Pts',(-39.086733089636,39.2655732066824,16.2342025468132));
#42783=CARTESIAN_POINT('Ctrl Pts',(-39.0859802984598,39.2727841565797,16.2318866577235));
#42784=CARTESIAN_POINT('Ctrl Pts',(-39.0851976546674,39.2799960143386,16.2296084227804));
#42785=CARTESIAN_POINT('Ctrl Pts',(-39.0843887635932,39.2872199202528,16.227368365464));
#42786=CARTESIAN_POINT('Ctrl Pts',(-39.0821852989432,39.3068982450882,16.2212663237091));
#42787=CARTESIAN_POINT('Ctrl Pts',(-39.0797811657753,39.3266296736303,16.2154445797335));
#42788=CARTESIAN_POINT('Ctrl Pts',(-39.0772180387328,39.3464197777051,16.2099084657454));
#42789=CARTESIAN_POINT('Ctrl Pts',(-39.0754357491048,39.3601809751188,16.2060588873295));
#42790=CARTESIAN_POINT('Ctrl Pts',(-39.0735764432121,39.3739705906881,16.2023472616272));
#42791=CARTESIAN_POINT('Ctrl Pts',(-39.0716534468229,39.3877906531785,16.1987731088965));
#42792=CARTESIAN_POINT('Ctrl Pts',(-39.0697077670658,39.4017737349879,16.1951567960131));
#42793=CARTESIAN_POINT('Ctrl Pts',(-39.0676967956697,39.4157878636927,16.1916811593399));
#42794=CARTESIAN_POINT('Ctrl Pts',(-39.0656363274421,39.4298353024344,16.1883485708264));
#42795=CARTESIAN_POINT('Ctrl Pts',(-39.0627317165124,39.4496377645914,16.1836506711497));
#42796=CARTESIAN_POINT('Ctrl Pts',(-39.0597289039457,39.4695066940188,16.1792373046652));
#42797=CARTESIAN_POINT('Ctrl Pts',(-39.0566705585344,39.4894474076504,16.1751065688499));
#42798=CARTESIAN_POINT('Ctrl Pts',(-39.0553071680152,39.4983368482646,16.1732651136541));
#42799=CARTESIAN_POINT('Ctrl Pts',(-39.0539328325859,39.5072405288181,16.1714799449962));
#42800=CARTESIAN_POINT('Ctrl Pts',(-39.0525528681501,39.5161521790931,16.1697524675246));
#42801=CARTESIAN_POINT('Ctrl Pts',(-39.0512871217776,39.5243262223628,16.1681679713691));
#42802=CARTESIAN_POINT('Ctrl Pts',(-39.0500165629401,39.5325070881124,16.1666320070914));
#42803=CARTESIAN_POINT('Ctrl Pts',(-39.0487453928414,39.540689545901,16.165145081683));
#42804=CARTESIAN_POINT('Ctrl Pts',(-39.0460883451561,39.5577928277904,16.1620370541116));
#42805=CARTESIAN_POINT('Ctrl Pts',(-39.0434267036561,39.574915257398,16.1591411118856));
#42806=CARTESIAN_POINT('Ctrl Pts',(-39.0407917137069,39.5920596775563,16.1564516597163));
#42807=CARTESIAN_POINT('Ctrl Pts',(-39.0365649129289,39.6195611291217,16.1521374958141));
#42808=CARTESIAN_POINT('Ctrl Pts',(-39.0324051221603,39.6471188125438,16.1483543509625));
#42809=CARTESIAN_POINT('Ctrl Pts',(-39.0284495518797,39.6747449792293,16.1450705587353));
#42810=CARTESIAN_POINT('Ctrl Pts',(-39.0274733127469,39.6815631478105,16.1442601151711));
#42811=CARTESIAN_POINT('Ctrl Pts',(-39.0265094328012,39.6883854420688,16.143479855215));
#42812=CARTESIAN_POINT('Ctrl Pts',(-39.0255598220946,39.6952119531012,16.1427288579772));
#42813=CARTESIAN_POINT('Ctrl Pts',(-39.0253702851041,39.6965744865557,16.1425789631253));
#42814=CARTESIAN_POINT('Ctrl Pts',(-39.025181313738,39.6979371831495,16.1424302302673));
#42815=CARTESIAN_POINT('Ctrl Pts',(-39.024992926915,39.6993000467681,16.1422826560201));
#42816=CARTESIAN_POINT('Ctrl Pts',(-39.0214262186056,39.7251030032366,16.1394886480019));
#42817=CARTESIAN_POINT('Ctrl Pts',(-39.0180708061177,39.7509672726913,16.1371132295503));
#42818=CARTESIAN_POINT('Ctrl Pts',(-39.0150463870856,39.7769022070589,16.135109441488));
#42819=CARTESIAN_POINT('Ctrl Pts',(-39.0141873375696,39.7842687103705,16.1345402898107));
#42820=CARTESIAN_POINT('Ctrl Pts',(-39.0133548629673,39.7916408279094,16.1340008353982));
#42821=CARTESIAN_POINT('Ctrl Pts',(-39.0125513944238,39.7990185563883,16.1334893473139));
#42822=CARTESIAN_POINT('Ctrl Pts',(-39.0099373559885,39.8230215692805,16.1318252504152));
#42823=CARTESIAN_POINT('Ctrl Pts',(-39.0076304951035,39.8470819631763,16.1304589284462));
#42824=CARTESIAN_POINT('Ctrl Pts',(-39.005733443495,39.871213035224,16.1293377024353));
#42825=CARTESIAN_POINT('Ctrl Pts',(-39.004959266345,39.8810608034669,16.1288801357809));
#42826=CARTESIAN_POINT('Ctrl Pts',(-39.0042530766643,39.8909201437646,16.128462873272));
#42827=CARTESIAN_POINT('Ctrl Pts',(-39.0036206852641,39.9007910684579,16.1280803373666));
#42828=CARTESIAN_POINT('Ctrl Pts',(-39.0035609301979,39.9017237784193,16.1280441913052));
#42829=CARTESIAN_POINT('Ctrl Pts',(-39.0035018335811,39.9026565289322,16.1280083528885));
#42830=CARTESIAN_POINT('Ctrl Pts',(-39.0034433999712,39.9035893197067,16.1279728172578));
#42831=CARTESIAN_POINT('Ctrl Pts',(-39.0023473053679,39.9210865603477,16.1273062417523));
#42832=CARTESIAN_POINT('Ctrl Pts',(-39.0014873834615,39.9386193782255,16.1267495520393));
#42833=CARTESIAN_POINT('Ctrl Pts',(-39.0009007469202,39.9561889486819,16.1262726075685));
#42834=CARTESIAN_POINT('Ctrl Pts',(-39.0006074286495,39.9649737339102,16.1260341353331));
#42835=CARTESIAN_POINT('Ctrl Pts',(-39.0003824779079,39.9737677102205,16.1258155565433));
#42836=CARTESIAN_POINT('Ctrl Pts',(-39.0002308110869,39.9825710305249,16.1256127882412));
#42837=CARTESIAN_POINT('Ctrl Pts',(-39.0001549776764,39.9869726906771,16.1255114040901));
#42838=CARTESIAN_POINT('Ctrl Pts',(-39.0000974681329,39.9913766867925,16.1254139687993));
#42839=CARTESIAN_POINT('Ctrl Pts',(-39.0000589140448,39.995783037166,16.1253199473816));
#42840=CARTESIAN_POINT('Ctrl Pts',(-39.0000396370008,39.9979862123527,16.1252729366727));
#42841=CARTESIAN_POINT('Ctrl Pts',(-39.0000250989958,40.0001899760904,16.1252267791589));
#42842=CARTESIAN_POINT('Ctrl Pts',(-39.000015380015,40.0023943305614,16.1251814062609));
#42843=CARTESIAN_POINT('Ctrl Pts',(-39.0000105205245,40.0034965077969,16.1251587198119));
#42844=CARTESIAN_POINT('Ctrl Pts',(-39.0000068658008,40.0045988327145,16.1251362294985));
#42845=CARTESIAN_POINT('Ctrl Pts',(-39.0000044259056,40.0057013055785,16.1251139266363));
#42846=CARTESIAN_POINT('Ctrl Pts',(-39.0000019860103,40.0068037784424,16.125091623774));
#42847=CARTESIAN_POINT('Ctrl Pts',(-39.0000007609435,40.0079063992528,16.125069508363));
#42848=CARTESIAN_POINT('Ctrl Pts',(-39.0000007608086,40.0090091682675,16.125047571642));
#42849=CARTESIAN_POINT('Ctrl Pts',(-39.,38.3487778137292,16.1565988728829));
#42850=CARTESIAN_POINT('Ctrl Pts',(-39.,38.3833934352842,16.1653602760744));
#42851=CARTESIAN_POINT('Ctrl Pts',(-39.0007271289037,38.418056230505,16.1734834106599));
#42852=CARTESIAN_POINT('Ctrl Pts',(-39.0033844025761,38.4874821615589,16.1885397585578));
#42853=CARTESIAN_POINT('Ctrl Pts',(-39.0053154013728,38.5222452565794,16.1954728002341));
#42854=CARTESIAN_POINT('Ctrl Pts',(-39.0126341194485,38.6266906398611,16.2145895490314));
#42855=CARTESIAN_POINT('Ctrl Pts',(-39.0195339780508,38.6965293017166,16.2250958545813));
#42856=CARTESIAN_POINT('Ctrl Pts',(-39.0321447527579,38.8016129939812,16.2377952286948));
#42857=CARTESIAN_POINT('Ctrl Pts',(-39.0367291513417,38.8366950810595,16.2415169611478));
#42858=CARTESIAN_POINT('Ctrl Pts',(-39.0441085920868,38.8894005968051,16.2463592266313));
#42859=CARTESIAN_POINT('Ctrl Pts',(-39.0466519979229,38.9069797098678,16.2478494670046));
#42860=CARTESIAN_POINT('Ctrl Pts',(-39.0518885060209,38.9421114193367,16.2505832282473));
#42861=CARTESIAN_POINT('Ctrl Pts',(-39.065360489734,39.029907703484,16.2568029716959));
#42862=CARTESIAN_POINT('Ctrl Pts',(-39.0805958020047,39.1175586211149,16.260024347864));
#42863=CARTESIAN_POINT('Ctrl Pts',(-39.0936699647319,39.1876203501829,16.2608089943269));
#42864=CARTESIAN_POINT('Origin',(-39.5,34.999999994595,6.54998265276524E-10));
#42865=CARTESIAN_POINT('Origin',(-39.,34.999999994595,6.54998265276524E-10));
#42866=CARTESIAN_POINT('Origin',(-39.5,42.1186371575735,14.8853956938121));
#42867=CARTESIAN_POINT('Origin',(-39.5,34.999999994595,6.54998265276524E-10));
#42868=CARTESIAN_POINT('',(-39.,18.5084035288379,-0.52654155575758));
#42869=CARTESIAN_POINT('Ctrl Pts',(-39.5,18.2644264063412,-2.98673344445558));
#42870=CARTESIAN_POINT('Ctrl Pts',(-39.4982565645427,18.2632940298282,-2.98038839532042));
#42871=CARTESIAN_POINT('Ctrl Pts',(-39.4965117602025,18.2621733491251,-2.97403614595641));
#42872=CARTESIAN_POINT('Ctrl Pts',(-39.4947636361374,18.2610631637812,-2.96766936765203));
#42873=CARTESIAN_POINT('Ctrl Pts',(-39.4930155120723,18.2599529784372,-2.96130258934765));
#42874=CARTESIAN_POINT('Ctrl Pts',(-39.4912678321557,18.2588557079406,-2.95493499688772));
#42875=CARTESIAN_POINT('Ctrl Pts',(-39.4895206393129,18.2577713218828,-2.94856658238146));
#42876=CARTESIAN_POINT('Ctrl Pts',(-39.4860262536273,18.2556025497672,-2.93582975336894));
#42877=CARTESIAN_POINT('Ctrl Pts',(-39.4825338167734,18.2534853302707,-2.92308963332142));
#42878=CARTESIAN_POINT('Ctrl Pts',(-39.4790436750457,18.2514195389397,-2.91034613927784));
#42879=CARTESIAN_POINT('Ctrl Pts',(-39.4720633915901,18.2472879562777,-2.88485915119069));
#42880=CARTESIAN_POINT('Ctrl Pts',(-39.4650922877873,18.2433620564643,-2.85935867096065));
#42881=CARTESIAN_POINT('Ctrl Pts',(-39.4581331343936,18.2396411072223,-2.83384400738141));
#42882=CARTESIAN_POINT('Ctrl Pts',(-39.4442148276061,18.2321992087383,-2.78281468022295));
#42883=CARTESIAN_POINT('Ctrl Pts',(-39.4303442716327,18.2255766539551,-2.73172870279065));
#42884=CARTESIAN_POINT('Ctrl Pts',(-39.4165440806474,18.2197717559618,-2.68058028152748));
#42885=CARTESIAN_POINT('Ctrl Pts',(-39.3889436986768,18.2081619599752,-2.57828343900114));
#42886=CARTESIAN_POINT('Ctrl Pts',(-39.3616221749354,18.1998153193335,-2.47573793659964));
#42887=CARTESIAN_POINT('Ctrl Pts',(-39.3347784476018,18.1947856738467,-2.37288927501648));
#42888=CARTESIAN_POINT('Ctrl Pts',(-39.3335875496944,18.1945625381319,-2.368326486312));
#42889=CARTESIAN_POINT('Ctrl Pts',(-39.3323975904841,18.1943459235456,-2.36376309599717));
#42890=CARTESIAN_POINT('Ctrl Pts',(-39.331208587611,18.1941358327567,-2.35919910078715));
#42891=CARTESIAN_POINT('Ctrl Pts',(-39.3055965786381,18.1896103204193,-2.26088723887917));
#42892=CARTESIAN_POINT('Ctrl Pts',(-39.2804265332853,18.1881140973325,-2.16229734459659));
#42893=CARTESIAN_POINT('Ctrl Pts',(-39.2559179426822,18.1897840045728,-2.06336481042167));
#42894=CARTESIAN_POINT('Ctrl Pts',(-39.2543480339218,18.1898909712298,-2.05702764258509));
#42895=CARTESIAN_POINT('Ctrl Pts',(-39.2527808346664,18.1900109130978,-2.05068906626546));
#42896=CARTESIAN_POINT('Ctrl Pts',(-39.2512164033361,18.1901438593256,-2.04434907378134));
#42897=CARTESIAN_POINT('Ctrl Pts',(-39.2400023905221,18.1910968322516,-1.99890332261146));
#42898=CARTESIAN_POINT('Ctrl Pts',(-39.2289314687727,18.1927201844435,-1.95338409824031));
#42899=CARTESIAN_POINT('Ctrl Pts',(-39.2180308629908,18.1950353121287,-1.9077834153972));
#42900=CARTESIAN_POINT('Ctrl Pts',(-39.2162879759569,18.1954054755953,-1.90049236749997));
#42901=CARTESIAN_POINT('Ctrl Pts',(-39.2145494600503,18.1957933142013,-1.89319931660478));
#42902=CARTESIAN_POINT('Ctrl Pts',(-39.2128154190889,18.1961989089874,-1.8859042096267));
#42903=CARTESIAN_POINT('Ctrl Pts',(-39.2096666341135,18.1969354145239,-1.8726572773113));
#42904=CARTESIAN_POINT('Ctrl Pts',(-39.2065326463223,18.1977305429674,-1.85940352639851));
#42905=CARTESIAN_POINT('Ctrl Pts',(-39.2034141624684,18.1985849209553,-1.84614255750622));
#42906=CARTESIAN_POINT('Ctrl Pts',(-39.2021303279584,18.1989366559641,-1.84068320921452));
#42907=CARTESIAN_POINT('Ctrl Pts',(-39.2008487219748,18.1992985676539,-1.83522091067537));
#42908=CARTESIAN_POINT('Ctrl Pts',(-39.1995701568081,18.1996704526564,-1.82975891490213));
#42909=CARTESIAN_POINT('Ctrl Pts',(-39.1977421510071,18.2002021486229,-1.82194972361643));
#42910=CARTESIAN_POINT('Ctrl Pts',(-39.1959192655843,18.2007545485336,-1.81413647416283));
#42911=CARTESIAN_POINT('Ctrl Pts',(-39.1941037111139,18.2013271931799,-1.80632787186134));
#42912=CARTESIAN_POINT('Ctrl Pts',(-39.1898662232147,18.2026637406637,-1.78810266391492));
#42913=CARTESIAN_POINT('Ctrl Pts',(-39.1856666064574,18.2041108748653,-1.76989434449253));
#42914=CARTESIAN_POINT('Ctrl Pts',(-39.1815045041788,18.2056702971502,-1.75169250579292));
#42915=CARTESIAN_POINT('Ctrl Pts',(-39.1796210579155,18.2063759713213,-1.74345575840182));
#42916=CARTESIAN_POINT('Ctrl Pts',(-39.1777454922288,18.2071045751166,-1.7352212012678));
#42917=CARTESIAN_POINT('Ctrl Pts',(-39.1758779937713,18.2078561914943,-1.72698881253716));
#42918=CARTESIAN_POINT('Ctrl Pts',(-39.1541654270963,18.2165948978911,-1.63127452238991));
#42919=CARTESIAN_POINT('Ctrl Pts',(-39.133529694962,18.2284326450439,-1.53585516105736));
#42920=CARTESIAN_POINT('Ctrl Pts',(-39.1143518851541,18.2435811130114,-1.44068967460049));
#42921=CARTESIAN_POINT('Ctrl Pts',(-39.1125541406822,18.2450011434956,-1.43176877962281));
#42922=CARTESIAN_POINT('Ctrl Pts',(-39.1107692087929,18.2464502566782,-1.42285010476126));
#42923=CARTESIAN_POINT('Ctrl Pts',(-39.1089974104922,18.2479286136716,-1.41393362056419));
#42924=CARTESIAN_POINT('Ctrl Pts',(-39.1005058581712,18.2550138139192,-1.37120031844464));
#42925=CARTESIAN_POINT('Ctrl Pts',(-39.0923179063329,18.2627729609616,-1.32851751678849));
#42926=CARTESIAN_POINT('Ctrl Pts',(-39.0844832261953,18.271236307921,-1.28588020640277));
#42927=CARTESIAN_POINT('Ctrl Pts',(-39.0828756161155,18.2729729151138,-1.27713139103993));
#42928=CARTESIAN_POINT('Ctrl Pts',(-39.0812828770768,18.2747391740245,-1.26838447431847));
#42929=CARTESIAN_POINT('Ctrl Pts',(-39.0797054438143,18.276535337416,-1.25963942990192));
#42930=CARTESIAN_POINT('Ctrl Pts',(-39.0719912104367,18.2853192422034,-1.2168729210884));
#42931=CARTESIAN_POINT('Ctrl Pts',(-39.064642510105,18.2948181395909,-1.17415144094987));
#42932=CARTESIAN_POINT('Ctrl Pts',(-39.0577257707355,18.3050731128552,-1.1314683987587));
#42933=CARTESIAN_POINT('Ctrl Pts',(-39.0563799319872,18.30706849531,-1.1231632582857));
#42934=CARTESIAN_POINT('Ctrl Pts',(-39.0550503898463,18.3090925886837,-1.11485922024422));
#42935=CARTESIAN_POINT('Ctrl Pts',(-39.053737708826,18.3111455823682,-1.10655668676609));
#42936=CARTESIAN_POINT('Ctrl Pts',(-39.0517286769875,18.3142876478149,-1.09384982665325));
#42937=CARTESIAN_POINT('Ctrl Pts',(-39.0497593032948,18.3174975330194,-1.08114645633668));
#42938=CARTESIAN_POINT('Ctrl Pts',(-39.0478319313426,18.3207761133243,-1.06844792063594));
#42939=CARTESIAN_POINT('Ctrl Pts',(-39.0471208500752,18.3219857070594,-1.0637629448841));
#42940=CARTESIAN_POINT('Ctrl Pts',(-39.0464152375459,18.323205119103,-1.05907690212186));
#42941=CARTESIAN_POINT('Ctrl Pts',(-39.0457155529325,18.3244337666235,-1.05439218017061));
#42942=CARTESIAN_POINT('Ctrl Pts',(-39.044520955394,18.3265314821878,-1.04639378031453));
#42943=CARTESIAN_POINT('Ctrl Pts',(-39.0433430534469,18.3286571222814,-1.03839536818302));
#42944=CARTESIAN_POINT('Ctrl Pts',(-39.0421834943012,18.330809197905,-1.03040397925429));
#42945=CARTESIAN_POINT('Ctrl Pts',(-39.0414816456199,18.3321117890182,-1.02556701530778));
#42946=CARTESIAN_POINT('Ctrl Pts',(-39.040786633438,18.333423792319,-1.0207335461338));
#42947=CARTESIAN_POINT('Ctrl Pts',(-39.0400984395507,18.3347455178494,-1.01590260391144));
#42948=CARTESIAN_POINT('Ctrl Pts',(-39.0382732462829,18.3382509319266,-1.00309022155061));
#42949=CARTESIAN_POINT('Ctrl Pts',(-39.0364962908506,18.3418242089596,-0.990297549473336));
#42950=CARTESIAN_POINT('Ctrl Pts',(-39.0347699154051,18.3454662563153,-0.977524706607762));
#42951=CARTESIAN_POINT('Ctrl Pts',(-39.0337567600377,18.3476036591823,-0.970028727480062));
#42952=CARTESIAN_POINT('Ctrl Pts',(-39.0327610270135,18.3497647464099,-0.962539592535702));
#42953=CARTESIAN_POINT('Ctrl Pts',(-39.0317831970767,18.3519497059365,-0.955057313744942));
#42954=CARTESIAN_POINT('Ctrl Pts',(-39.0260962976061,18.3646570742702,-0.911541600336059));
#42955=CARTESIAN_POINT('Ctrl Pts',(-39.0210121201334,18.3781709589092,-0.868257443629536));
#42956=CARTESIAN_POINT('Ctrl Pts',(-39.0166488781946,18.3925369729867,-0.825211111031793));
#42957=CARTESIAN_POINT('Ctrl Pts',(-39.0160595867312,18.3944772205315,-0.819397352206009));
#42958=CARTESIAN_POINT('Ctrl Pts',(-39.0154834597696,18.3964330177636,-0.813587937240513));
#42959=CARTESIAN_POINT('Ctrl Pts',(-39.0149208018372,18.3984044833367,-0.807782873087525));
#42960=CARTESIAN_POINT('Ctrl Pts',(-39.010601091197,18.4135400751802,-0.763215479751383));
#42961=CARTESIAN_POINT('Ctrl Pts',(-39.0070725985321,18.4295985556218,-0.718904554302151));
#42962=CARTESIAN_POINT('Ctrl Pts',(-39.004522940544,18.446649756052,-0.674858878290108));
#42963=CARTESIAN_POINT('Ctrl Pts',(-39.0043320691178,18.4479262358618,-0.671561549379601));
#42964=CARTESIAN_POINT('Ctrl Pts',(-39.0041466913404,18.4492082820768,-0.668265708929566));
#42965=CARTESIAN_POINT('Ctrl Pts',(-39.0039668898115,18.4504959258862,-0.66497135916845));
#42966=CARTESIAN_POINT('Ctrl Pts',(-39.001432063524,18.4686490161198,-0.618527903270653));
#42967=CARTESIAN_POINT('Ctrl Pts',(-39.,18.4879134182867,-0.572380484667404));
#42968=CARTESIAN_POINT('Ctrl Pts',(-39.,18.5084035288379,-0.52654155575758));
#42969=CARTESIAN_POINT('Origin',(-39.,34.999999994595,6.54998265276524E-10));
#42970=CARTESIAN_POINT('Origin',(-39.5,39.1149554701578,15.978646421242));
#42971=CARTESIAN_POINT('Origin',(-38.5,20.7255401693197,-2.54750793782168));
#42972=CARTESIAN_POINT('',(-39.,19.7255401693197,0.28091918692451));
#42973=CARTESIAN_POINT('Ctrl Pts',(-38.5,20.2255401693197,-0.0980181950385015));
#42974=CARTESIAN_POINT('Ctrl Pts',(-38.5068454246389,20.2255401693197,-0.0980181950385014));
#42975=CARTESIAN_POINT('Ctrl Pts',(-38.5137049378611,20.2253995984199,-0.0979034111946665));
#42976=CARTESIAN_POINT('Ctrl Pts',(-38.574487053383,20.2228963259888,-0.0958597862843734));
#42977=CARTESIAN_POINT('Ctrl Pts',(-38.6266179130002,20.2120282571218,-0.0869664209613772));
#42978=CARTESIAN_POINT('Ctrl Pts',(-38.7343668418878,20.1716895730688,-0.0543730508899982));
#42979=CARTESIAN_POINT('Ctrl Pts',(-38.7864380337499,20.1394945590217,-0.0285603789798399));
#42980=CARTESIAN_POINT('Ctrl Pts',(-38.8850764070749,20.0527224260415,0.0395179277114487));
#42981=CARTESIAN_POINT('Ctrl Pts',(-38.9288507671718,19.9929196181174,0.0855519592453916));
#42982=CARTESIAN_POINT('Ctrl Pts',(-38.9855092027928,19.863098833122,0.182314659292735));
#42983=CARTESIAN_POINT('Ctrl Pts',(-38.9995659056513,19.7961082948418,0.230981573726129));
#42984=CARTESIAN_POINT('Ctrl Pts',(-38.9999967004912,19.7276374941665,0.279435862662001));
#42985=CARTESIAN_POINT('Ctrl Pts',(-39.,19.7265889001319,0.280177622255819));
#42986=CARTESIAN_POINT('Ctrl Pts',(-39.,19.7255401693201,0.28091918692451));
#42987=CARTESIAN_POINT('Origin',(-39.,20.7255401693197,-2.54750793782168));
#42988=CARTESIAN_POINT('Origin',(-38.5,18.5084035288379,-0.52654155575758));
#42989=CARTESIAN_POINT('Ctrl Pts',(-38.5,18.8779263022516,-0.863369286101596));
#42990=CARTESIAN_POINT('Ctrl Pts',(-39.,18.8779263022516,-0.863369286101596));
#42991=CARTESIAN_POINT('Ctrl Pts',(-39.,18.5084035288379,-0.526541555757579));
#42992=CARTESIAN_POINT('Ctrl Pts',(-38.5000000121044,18.8428991572258,-0.901796430331833));
#42993=CARTESIAN_POINT('Ctrl Pts',(-38.9846448633454,18.8534834999705,-0.890184678462895));
#42994=CARTESIAN_POINT('Ctrl Pts',(-39.,18.4881009996417,-0.571960841817054));
#42995=CARTESIAN_POINT('Ctrl Pts',(-38.5028175697433,18.8093997703974,-0.940951127436968));
#42996=CARTESIAN_POINT('Ctrl Pts',(-38.9716161398923,18.8276179047806,-0.919547640497487));
#42997=CARTESIAN_POINT('Ctrl Pts',(-39.001408782789,18.4688157281884,-0.61810138075627));
#42998=CARTESIAN_POINT('Ctrl Pts',(-38.5130500106387,18.7452608184442,-1.02070981564836));
#42999=CARTESIAN_POINT('Ctrl Pts',(-38.9507774942834,18.7751212471768,-0.982362104350359));
#43000=CARTESIAN_POINT('Ctrl Pts',(-39.006525007402,18.4321760372884,-0.711841267055085));
#43001=CARTESIAN_POINT('Ctrl Pts',(-38.5204704459176,18.7146215389275,-1.06131431190728));
#43002=CARTESIAN_POINT('Ctrl Pts',(-38.9428107063041,18.7484926791068,-1.01571890599804));
#43003=CARTESIAN_POINT('Ctrl Pts',(-39.0102352215507,18.4148220173941,-0.759440668067828));
#43004=CARTESIAN_POINT('Ctrl Pts',(-38.5392127937583,18.6560779514862,-1.14397975473208));
#43005=CARTESIAN_POINT('Ctrl Pts',(-38.9317121494331,18.6955196203185,-1.08611448020077));
#43006=CARTESIAN_POINT('Ctrl Pts',(-39.0196063982873,18.3819868820653,-0.8561250274524));
#43007=CARTESIAN_POINT('Ctrl Pts',(-38.5505376800415,18.6281740998822,-1.18604062346602));
#43008=CARTESIAN_POINT('Ctrl Pts',(-38.9284460459492,18.6691391641143,-1.12309259491601));
#43009=CARTESIAN_POINT('Ctrl Pts',(-39.0252688391042,18.3665060238294,-0.905209872964393));
#43010=CARTESIAN_POINT('Ctrl Pts',(-38.5700807581267,18.5883170213382,-1.25023709676593));
#43011=CARTESIAN_POINT('Ctrl Pts',(-38.9268518414429,18.6301154171898,-1.18142532324));
#43012=CARTESIAN_POINT('Ctrl Pts',(-39.0350403795217,18.3446715373495,-0.979981027272348));
#43013=CARTESIAN_POINT('Ctrl Pts',(-38.5770224165533,18.5753648269077,-1.27182020968494));
#43014=CARTESIAN_POINT('Ctrl Pts',(-38.9268547426899,18.6173082485063,-1.20115921207614));
#43015=CARTESIAN_POINT('Ctrl Pts',(-39.0385112079161,18.3376247517694,-1.00509550606235));
#43016=CARTESIAN_POINT('Ctrl Pts',(-38.5880392751736,18.556433320345,-1.30447383795162));
#43017=CARTESIAN_POINT('Ctrl Pts',(-38.9276416963271,18.5982881776557,-1.23144666676493));
#43018=CARTESIAN_POINT('Ctrl Pts',(-39.0440196377671,18.3274014203209,-1.0430582153955));
#43019=CARTESIAN_POINT('Ctrl Pts',(-38.5918107280427,18.5502090235416,-1.31539948656175));
#43020=CARTESIAN_POINT('Ctrl Pts',(-38.9280311463852,18.5920097611487,-1.24160683011756));
#43021=CARTESIAN_POINT('Ctrl Pts',(-39.0459053636913,18.3240533247711,-1.05575467508082));
#43022=CARTESIAN_POINT('Ctrl Pts',(-38.5995170068257,18.537974590515,-1.33725438261636));
#43023=CARTESIAN_POINT('Ctrl Pts',(-38.9290567915728,18.5795930841744,-1.26203671753181));
#43024=CARTESIAN_POINT('Ctrl Pts',(-39.0497585037429,18.3174988913271,-1.08114115888948));
#43025=CARTESIAN_POINT('Ctrl Pts',(-38.6034554755142,18.5319580960745,-1.34819451677163));
#43026=CARTESIAN_POINT('Ctrl Pts',(-38.9296918352213,18.5734470765348,-1.2723168318538));
#43027=CARTESIAN_POINT('Ctrl Pts',(-39.0517277374561,18.3142891141038,-1.09384384268011));
#43028=CARTESIAN_POINT('Ctrl Pts',(-38.6235552691089,18.5023687406762,-1.4029605589706));
#43029=CARTESIAN_POINT('Ctrl Pts',(-38.9334287389161,18.5433014861436,-1.32359797225254));
#43030=CARTESIAN_POINT('Ctrl Pts',(-39.0617776357584,18.2985713692847,-1.15740800389106));
#43031=CARTESIAN_POINT('Ctrl Pts',(-38.6409338208112,18.4802721042523,-1.44698296900576));
#43032=CARTESIAN_POINT('Ctrl Pts',(-38.9382939320124,18.5199892666906,-1.36598545379934));
#43033=CARTESIAN_POINT('Ctrl Pts',(-39.0704669095817,18.2870548910152,-1.20842227191335));
#43034=CARTESIAN_POINT('Ctrl Pts',(-38.6778880423194,18.4390140339829,-1.53548910231471));
#43035=CARTESIAN_POINT('Ctrl Pts',(-38.9513053448041,18.4758073593947,-1.45244063995325));
#43036=CARTESIAN_POINT('Ctrl Pts',(-39.0889440219837,18.2660157117594,-1.31085653901257));
#43037=CARTESIAN_POINT('Ctrl Pts',(-38.6974651244877,18.4198532838473,-1.57997264774622));
#43038=CARTESIAN_POINT('Ctrl Pts',(-38.9593984641188,18.4548505882054,-1.4965504346942));
#43039=CARTESIAN_POINT('Ctrl Pts',(-39.0987325617014,18.2564934169457,-1.3622762904579));
#43040=CARTESIAN_POINT('Ctrl Pts',(-38.7590544808404,18.3665552095797,-1.71416757203857));
#43041=CARTESIAN_POINT('Ctrl Pts',(-38.9876508556077,18.3963878957642,-1.62990979111957));
#43042=CARTESIAN_POINT('Ctrl Pts',(-39.1295272415051,18.2307988288308,-1.51724815893203));
#43043=CARTESIAN_POINT('Ctrl Pts',(-38.8039018553468,18.3365825126792,-1.80462281697605));
#43044=CARTESIAN_POINT('Ctrl Pts',(-39.012095726413,18.3618241711421,-1.72283960130348));
#43045=CARTESIAN_POINT('Ctrl Pts',(-39.1519509272974,18.2174861530546,-1.62151228107335));
#43046=CARTESIAN_POINT('Ctrl Pts',(-38.863719532733,18.3056934244436,-1.91909402720029));
#43047=CARTESIAN_POINT('Ctrl Pts',(-39.0483420183347,18.3254434461637,-1.84301300206946));
#43048=CARTESIAN_POINT('Ctrl Pts',(-39.1818597664605,18.2054486954808,-1.7533579412421));
#43049=CARTESIAN_POINT('Ctrl Pts',(-38.8758729301451,18.2998460440467,-1.94205839310398));
#43050=CARTESIAN_POINT('Ctrl Pts',(-39.0557807395094,18.3185797826281,-1.86696003063784));
#43051=CARTESIAN_POINT('Ctrl Pts',(-39.187936465009,18.2032724058732,-1.779802873125));
#43052=CARTESIAN_POINT('Ctrl Pts',(-38.8943746691618,18.2915681837471,-1.97661332531131));
#43053=CARTESIAN_POINT('Ctrl Pts',(-39.0673289982722,18.3087953136981,-1.90315643956538));
#43054=CARTESIAN_POINT('Ctrl Pts',(-39.1971873346127,18.2003545864548,-1.81959037093966));
#43055=CARTESIAN_POINT('Ctrl Pts',(-38.9005893670775,18.2888903886097,-1.98815358276858));
#43056=CARTESIAN_POINT('Ctrl Pts',(-39.0712357141135,18.305624513315,-1.91524480475088));
#43057=CARTESIAN_POINT('Ctrl Pts',(-39.2002946834377,18.1994395715941,-1.83287735674673));
#43058=CARTESIAN_POINT('Ctrl Pts',(-38.9130672827963,18.2837149816403,-2.01119720590798));
#43059=CARTESIAN_POINT('Ctrl Pts',(-39.0791435396456,18.2994780043902,-1.93941653842486));
#43060=CARTESIAN_POINT('Ctrl Pts',(-39.2065336414992,18.1977302703166,-1.85940775826571));
#43061=CARTESIAN_POINT('Ctrl Pts',(-38.9193352153427,18.281215176572,-2.02270942842269));
#43062=CARTESIAN_POINT('Ctrl Pts',(-39.0831476831193,18.2964988066967,-1.95151041911247));
#43063=CARTESIAN_POINT('Ctrl Pts',(-39.2096676075802,18.1969351868286,-1.87266137268417));
#43064=CARTESIAN_POINT('Ctrl Pts',(-38.9508133295184,18.2691491038573,-2.08022508586583));
#43065=CARTESIAN_POINT('Ctrl Pts',(-39.1033178931505,18.2821373957891,-2.01174614075846));
#43066=CARTESIAN_POINT('Ctrl Pts',(-39.2254066651236,18.1932537976226,-1.9388755573968));
#43067=CARTESIAN_POINT('Ctrl Pts',(-38.9764375556006,18.2608798321247,-2.12609264637355));
#43068=CARTESIAN_POINT('Ctrl Pts',(-39.1202929972975,18.2720741420306,-2.06029596271023));
#43069=CARTESIAN_POINT('Ctrl Pts',(-39.2382187775668,18.1912484049181,-1.99167508271378));
#43070=CARTESIAN_POINT('Ctrl Pts',(-39.0544233622651,18.240018901072,-2.26334297249591));
#43071=CARTESIAN_POINT('Ctrl Pts',(-39.1728036049692,18.2464825605143,-2.20533681448651));
#43072=CARTESIAN_POINT('Ctrl Pts',(-39.2772116815981,18.1879347508401,-2.14969704063337));
#43073=CARTESIAN_POINT('Ctrl Pts',(-39.1078893586506,18.2313577128234,-2.35437654643091));
#43074=CARTESIAN_POINT('Ctrl Pts',(-39.2105403633043,18.2350636347238,-2.30311269780209));
#43075=CARTESIAN_POINT('Ctrl Pts',(-39.3039446791879,18.1893184331436,-2.25454639009119));
#43076=CARTESIAN_POINT('Ctrl Pts',(-39.2169451138417,18.2239187624629,-2.53583757407667));
#43077=CARTESIAN_POINT('Ctrl Pts',(-39.2890733295988,18.2238760787528,-2.49823411040255));
#43078=CARTESIAN_POINT('Ctrl Pts',(-39.3584725570583,18.1989532058266,-2.46385177983269));
#43079=CARTESIAN_POINT('Ctrl Pts',(-39.2725402949566,18.225144403491,-2.62626286641505));
#43080=CARTESIAN_POINT('Ctrl Pts',(-39.3300826313235,18.2239232442552,-2.59620144360494));
#43081=CARTESIAN_POINT('Ctrl Pts',(-39.3862701474838,18.2072061381291,-2.56830453161861));
#43082=CARTESIAN_POINT('Ctrl Pts',(-39.357082512524,18.234316031401,-2.76162852484942));
#43083=CARTESIAN_POINT('Ctrl Pts',(-39.392982196192,18.2326394199283,-2.74287394441288));
#43084=CARTESIAN_POINT('Ctrl Pts',(-39.4285412562593,18.2247429067445,-2.72507720804866));
#43085=CARTESIAN_POINT('Ctrl Pts',(-39.3854560789677,18.2385989626561,-2.806704608599));
#43086=CARTESIAN_POINT('Ctrl Pts',(-39.4141769794873,18.2369681932566,-2.79171803684677));
#43087=CARTESIAN_POINT('Ctrl Pts',(-39.4427280394942,18.2314503925561,-2.77735004009521));
#43088=CARTESIAN_POINT('Ctrl Pts',(-39.4282569904425,18.2468831045004,-2.87427088692559));
#43089=CARTESIAN_POINT('Ctrl Pts',(-39.4462140714394,18.2456335650916,-2.86492145390258));
#43090=CARTESIAN_POINT('Ctrl Pts',(-39.4641284952161,18.2428263134802,-2.85583107289212));
#43091=CARTESIAN_POINT('Ctrl Pts',(-39.4425640907085,18.2499546634831,-2.89678499625148));
#43092=CARTESIAN_POINT('Ctrl Pts',(-39.4569337160795,18.2488829564956,-2.88931200575023));
#43093=CARTESIAN_POINT('Ctrl Pts',(-39.471282045358,18.2468375527533,-2.88200339188145));
#43094=CARTESIAN_POINT('Ctrl Pts',(-39.4640790716987,18.2550319670924,-2.9305467580359));
#43095=CARTESIAN_POINT('Ctrl Pts',(-39.4730619699745,18.2543045238099,-2.92588285247038));
#43096=CARTESIAN_POINT('Ctrl Pts',(-39.4820395358475,18.2531874490028,-2.92128612729157));
#43097=CARTESIAN_POINT('Ctrl Pts',(-39.471259788484,18.2568027437311,-2.9417991113903));
#43098=CARTESIAN_POINT('Ctrl Pts',(-39.4784461726879,18.2562028894815,-2.9380706271792));
#43099=CARTESIAN_POINT('Ctrl Pts',(-39.4856298942431,18.2553595973052,-2.93438441656583));
#43100=CARTESIAN_POINT('Ctrl Pts',(-39.48204372096,18.2595771436823,-2.95867561371929));
#43101=CARTESIAN_POINT('Ctrl Pts',(-39.4865331229068,18.2591880585981,-2.9563486344656));
#43102=CARTESIAN_POINT('Ctrl Pts',(-39.4910218604795,18.2587017046828,-2.95403872240394));
#43103=CARTESIAN_POINT('Ctrl Pts',(-39.4856405081953,18.2605216504332,-2.96430077645969));
#43104=CARTESIAN_POINT('Ctrl Pts',(-39.4892305469675,18.2602060471952,-2.96244069404455));
#43105=CARTESIAN_POINT('Ctrl Pts',(-39.4928202540979,18.2598297219177,-2.96059130293824));
#43106=CARTESIAN_POINT('Ctrl Pts',(-39.4928382474395,18.2624502093871,-2.97555048018476));
#43107=CARTESIAN_POINT('Ctrl Pts',(-39.4946286518323,18.2622880271486,-2.97462353554838));
#43108=CARTESIAN_POINT('Ctrl Pts',(-39.4964191237195,18.2621138291545,-2.97369889104282));
#43109=CARTESIAN_POINT('Ctrl Pts',(-39.4964375477875,18.2634339488499,-2.98117240404692));
#43110=CARTESIAN_POINT('Ctrl Pts',(-39.4973281609331,18.2633517166985,-2.98071163235519));
#43111=CARTESIAN_POINT('Ctrl Pts',(-39.4982187739313,18.263269484497,-2.9802508603831));
#43112=CARTESIAN_POINT('Ctrl Pts',(-39.5,18.2644264063412,-2.98673344445558));
#43113=CARTESIAN_POINT('Ctrl Pts',(-39.5,18.2644264063412,-2.98673344445558));
#43114=CARTESIAN_POINT('Ctrl Pts',(-39.5,18.2644264063412,-2.98673344445558));
#43115=CARTESIAN_POINT('Origin',(-38.5,21.7255401693197,6.54991633351602E-10));
#43116=CARTESIAN_POINT('',(-39.,21.7255401693197,4.24538528099178));
#43117=CARTESIAN_POINT('',(-39.,21.7255401693197,-0.0980181950384951));
#43118=CARTESIAN_POINT('Origin',(-38.4999999999995,21.7255401693202,3.24538528099092));
#43119=CARTESIAN_POINT('Origin',(-44.,34.999999994595,6.55E-10));
#43120=CARTESIAN_POINT('',(-45.,20.5124191061237,-0.599999999345));
#43121=CARTESIAN_POINT('Origin',(-45.,34.999999994595,6.55E-10));
#43122=CARTESIAN_POINT('',(-44.,21.5133399188016,-0.599999999345));
#43123=CARTESIAN_POINT('Ctrl Pts',(-45.,20.5124191061237,-0.599999999344999));
#43124=CARTESIAN_POINT('Ctrl Pts',(-45.,20.6359758165694,-0.599999999344999));
#43125=CARTESIAN_POINT('Ctrl Pts',(-44.9710914795861,20.7813983486954,-0.599999999344999));
#43126=CARTESIAN_POINT('Ctrl Pts',(-44.8765874788021,21.009674170601,-0.599999999344999));
#43127=CARTESIAN_POINT('Ctrl Pts',(-44.7942865874973,21.1329323008594,-0.599999999345));
#43128=CARTESIAN_POINT('Ctrl Pts',(-44.6197204613676,21.3076006884133,-0.599999999345));
#43129=CARTESIAN_POINT('Ctrl Pts',(-44.4965862673463,21.3899370868742,-0.599999999345));
#43130=CARTESIAN_POINT('Ctrl Pts',(-44.2685787628921,21.4844357492405,-0.599999999345));
#43131=CARTESIAN_POINT('Ctrl Pts',(-44.123376209915,21.5133399188016,-0.599999999345));
#43132=CARTESIAN_POINT('Ctrl Pts',(-44.,21.5133399188016,-0.599999999345));
#43133=CARTESIAN_POINT('Origin',(-44.,34.999999994595,6.55E-10));
#43134=CARTESIAN_POINT('Origin',(-35.3179607461319,34.999999994595,6.55E-10));
#43135=CARTESIAN_POINT('',(-39.,26.0690696232311,-5.52163768230196));
#43136=CARTESIAN_POINT('',(-35.3179607461319,26.0690696232311,-5.52163768230196));
#43137=CARTESIAN_POINT('',(-41.5,40.1133069970551,-9.17082828792356));
#43138=CARTESIAN_POINT('Origin',(-41.5,34.999999994595,6.55E-10));
#43139=CARTESIAN_POINT('',(-39.,40.1133069970551,-9.17082828792356));
#43140=CARTESIAN_POINT('',(-35.3179607461319,40.1133069970551,-9.17082828792356));
#43141=CARTESIAN_POINT('Origin',(-39.,34.999999994595,6.55E-10));
#43142=CARTESIAN_POINT('Origin',(-35.3179607461319,45.925692710035,-9.04424050588343));
#43143=CARTESIAN_POINT('',(-39.,40.600288616337,-9.04424050588343));
#43144=CARTESIAN_POINT('',(-41.5,40.600288616337,-9.04424050588343));
#43145=CARTESIAN_POINT('',(-42.,40.600288616337,-9.04424050588343));
#43146=CARTESIAN_POINT('',(-41.5000000000004,45.7278783986988,-9.04424052035057));
#43147=CARTESIAN_POINT('',(-41.5,45.925692710035,-9.04424050588343));
#43148=CARTESIAN_POINT('Ctrl Pts',(-41.4999999863947,45.7278783849965,-9.04424050588343));
#43149=CARTESIAN_POINT('Ctrl Pts',(-41.4989575245769,45.7289134916217,-9.04424050588343));
#43150=CARTESIAN_POINT('Ctrl Pts',(-41.4979150491538,45.7299486117559,-9.04424050588343));
#43151=CARTESIAN_POINT('Ctrl Pts',(-41.496611954875,45.7312425119236,-9.04424050588343));
#43152=CARTESIAN_POINT('Ctrl Pts',(-41.4963410586823,45.731507728408,-9.04424050588343));
#43153=CARTESIAN_POINT('Ctrl Pts',(-41.4958079020604,45.7320316239049,-9.04424050588343));
#43154=CARTESIAN_POINT('Ctrl Pts',(-41.4950075021982,45.732816720824,-9.04424050588343));
#43155=CARTESIAN_POINT('Ctrl Pts',(-41.4920653807838,45.7356871913015,-9.04424050588343));
#43156=CARTESIAN_POINT('Ctrl Pts',(-41.485053521909,45.7424071161188,-9.04424050588343));
#43157=CARTESIAN_POINT('Ctrl Pts',(-41.4740518184729,45.7525050091841,-9.04424050588343));
#43158=CARTESIAN_POINT('Ctrl Pts',(-41.4650206065347,45.7603253376589,-9.04424050588343));
#43159=CARTESIAN_POINT('Ctrl Pts',(-41.455874133144,45.7680162950512,-9.04424050588343));
#43160=CARTESIAN_POINT('Ctrl Pts',(-41.4512386468437,45.7718007126244,-9.04424050588343));
#43161=CARTESIAN_POINT('Ctrl Pts',(-41.4278314383774,45.7903528744546,-9.04424050588343));
#43162=CARTESIAN_POINT('Ctrl Pts',(-41.408427535806,45.803971097651,-9.04424050588343));
#43163=CARTESIAN_POINT('Ctrl Pts',(-41.3683622144799,45.8289387080156,-9.04424050588343));
#43164=CARTESIAN_POINT('Ctrl Pts',(-41.3270405528109,45.8516396038261,-9.04424050588343));
#43165=CARTESIAN_POINT('Ctrl Pts',(-41.2833493406892,45.8700653089784,-9.04424050588343));
#43166=CARTESIAN_POINT('Ctrl Pts',(-41.2553247044489,45.8802866146071,-9.04424050588343));
#43167=CARTESIAN_POINT('Ctrl Pts',(-41.2496913297918,45.8822630341662,-9.04424050588343));
#43168=CARTESIAN_POINT('Ctrl Pts',(-41.2384136513533,45.8860676194529,-9.04424050588343));
#43169=CARTESIAN_POINT('Ctrl Pts',(-41.2214609174604,45.8915593252978,-9.04424050588343));
#43170=CARTESIAN_POINT('Ctrl Pts',(-41.2044024102307,45.8964225983601,-9.04424050588343));
#43171=CARTESIAN_POINT('Ctrl Pts',(-41.1701505715342,45.9053481111329,-9.04424050588343));
#43172=CARTESIAN_POINT('Ctrl Pts',(-41.1241226655105,45.9151171234807,-9.04424050588343));
#43173=CARTESIAN_POINT('Ctrl Pts',(-41.0540721293783,45.9237777729692,-9.04424050588343));
#43174=CARTESIAN_POINT('Ctrl Pts',(-41.0067222812585,45.9256927100353,-9.04424050588343));
#43175=CARTESIAN_POINT('Ctrl Pts',(-40.9828862029043,45.925692710035,-9.04424050588343));
#43176=CARTESIAN_POINT('',(-39.,34.999999994595,-9.04424050588343));
#43177=CARTESIAN_POINT('Origin',(-41.5,34.999999994595,6.55E-10));
#43178=CARTESIAN_POINT('',(-42.,39.8698161874141,-8.73412217894363));
#43179=CARTESIAN_POINT('Origin',(-42.,34.999999994595,6.55E-10));
#43180=CARTESIAN_POINT('Origin',(-41.5,39.8698161874141,-8.73412217894363));
#43181=CARTESIAN_POINT('Origin',(-35.3179607461319,40.600288616337,-10.0442405058834));
#43182=CARTESIAN_POINT('Origin',(-41.5,40.600288616337,-10.0442405058834));
#43183=CARTESIAN_POINT('Origin',(-39.,40.600288616337,-10.0442405058834));
#43184=CARTESIAN_POINT('Origin',(-39.,52.6127679742695,-3.71354333343353));
#43185=CARTESIAN_POINT('',(-45.5,51.7756531463269,-4.26057054010477));
#43186=CARTESIAN_POINT('',(-45.,51.7756531463269,-4.26057054010477));
#43187=CARTESIAN_POINT('',(-39.,51.7756531463269,-4.26057054010477));
#43188=CARTESIAN_POINT('Origin',(-45.5,52.6127679742695,-3.71354333343353));
#43189=CARTESIAN_POINT('Origin',(-45.,52.6127679742695,-3.71354333343353));
#43190=CARTESIAN_POINT('Origin',(-35.3179607461319,25.2185048259584,-6.04750793782168));
#43191=CARTESIAN_POINT('',(-39.,25.2185048259584,-5.04750793782168));
#43192=CARTESIAN_POINT('',(-39.,25.2185048259584,-5.04750793782168));
#43193=CARTESIAN_POINT('Origin',(-39.,25.2185048259584,-6.04750793782168));
#43194=CARTESIAN_POINT('Origin',(-45.,50.5871414377259,-8.30646623141651));
#43195=CARTESIAN_POINT('',(-45.,50.8553569437039,-8.43044283154557));
#43196=CARTESIAN_POINT('',(-45.,50.5871414377259,-8.30646623141651));
#43197=CARTESIAN_POINT('',(-45.,50.5871414377259,-8.30646623141651));
#43198=CARTESIAN_POINT('Origin',(-45.,48.5946168001447,-6.3392739254555));
#43199=CARTESIAN_POINT('',(-45.,47.8027400910494,-6.80733765974042));
#43200=CARTESIAN_POINT('Origin',(-29.,57.5946168001448,-3.5392739254555));
#43201=CARTESIAN_POINT('',(-39.,57.5946168001448,-3.5392739254555));
#43202=CARTESIAN_POINT('',(-39.,57.5946168001448,0.460726074544505));
#43203=CARTESIAN_POINT('',(-39.,57.5946168001448,0.960726074544506));
#43204=CARTESIAN_POINT('',(-29.,57.5946168001448,0.460726074544506));
#43205=CARTESIAN_POINT('',(-33.5,57.5946168001448,-3.5392739254555));
#43206=CARTESIAN_POINT('',(-33.5,57.5946168001448,-3.5392739254555));
#43207=CARTESIAN_POINT('',(-29.,57.5946168001448,-3.5392739254555));
#43208=CARTESIAN_POINT('Origin',(-46.,24.5171568688013,-0.599999999345));
#43209=CARTESIAN_POINT('',(-45.5,29.0300753719553,-0.599999999345));
#43210=CARTESIAN_POINT('',(-42.5,29.0300753719553,-0.599999999345));
#43211=CARTESIAN_POINT('',(-42.,29.0300753719553,-0.599999999345));
#43212=CARTESIAN_POINT('',(-42.4999999999993,21.3792341097314,-0.599999999345));
#43213=CARTESIAN_POINT('',(-42.5,20.5124191061237,-0.599999999345));
#43214=CARTESIAN_POINT('',(-43.,21.5133399188016,-0.599999999345));
#43215=CARTESIAN_POINT('Ctrl Pts',(-43.,21.5133399188016,-0.599999999345));
#43216=CARTESIAN_POINT('Ctrl Pts',(-42.876623790085,21.5133399188016,-0.599999999345));
#43217=CARTESIAN_POINT('Ctrl Pts',(-42.7314212371079,21.4844357492405,-0.599999999345));
#43218=CARTESIAN_POINT('Ctrl Pts',(-42.5789143576127,21.4212286361744,-0.599999999345));
#43219=CARTESIAN_POINT('Ctrl Pts',(-42.5390282352261,21.4017889231421,-0.599999999345));
#43220=CARTESIAN_POINT('Ctrl Pts',(-42.4999999999992,21.3792341097314,-0.599999999345));
#43221=CARTESIAN_POINT('',(-35.8316689588642,21.5133399188016,-0.599999999345));
#43222=CARTESIAN_POINT('',(-45.,19.0050007760892,-0.599999999345));
#43223=CARTESIAN_POINT('',(-45.,20.1123922190465,-0.599999999345));
#43224=CARTESIAN_POINT('',(-45.5,19.0050007760892,-0.599999999345));
#43225=CARTESIAN_POINT('',(-46.,19.0050007760892,-0.599999999345));
#43226=CARTESIAN_POINT('',(-45.5,24.5171568688013,-0.599999999345));
#43227=CARTESIAN_POINT('Origin',(-38.5,19.7255401693197,6.5499063415088E-10));
#43228=CARTESIAN_POINT('',(-38.9999999569785,19.7255368100699,4.2453886351283));
#43229=CARTESIAN_POINT('Origin',(-38.4999787117434,19.7255206107479,3.24531886108545));
#43230=CARTESIAN_POINT('',(-39.,19.7255401693197,4.45249206217833));
#43231=CARTESIAN_POINT('Ctrl Pts',(-39.1464465764959,21.7257963191156,4.59893863867423));
#43232=CARTESIAN_POINT('Ctrl Pts',(-38.9999593663855,21.7257212747019,4.45245142856379));
#43233=CARTESIAN_POINT('Ctrl Pts',(-38.9999999931593,21.7256682191115,4.24528722681498));
#43234=CARTESIAN_POINT('Ctrl Pts',(-39.1464634170654,21.6602603482896,4.59895547924376));
#43235=CARTESIAN_POINT('Ctrl Pts',(-38.9999748341363,21.6793856140906,4.45246689631453));
#43236=CARTESIAN_POINT('Ctrl Pts',(-39.0000084101164,21.692906657039,4.24530406763262));
#43237=CARTESIAN_POINT('Ctrl Pts',(-39.1400171767355,21.5947258251822,4.59250923891378));
#43238=CARTESIAN_POINT('Ctrl Pts',(-38.994046097433,21.6329311996428,4.44653815961128));
#43239=CARTESIAN_POINT('Ctrl Pts',(-38.9967865689158,21.6601458581973,4.23885771343968));
#43240=CARTESIAN_POINT('Ctrl Pts',(-39.1144632601427,21.4662576111171,4.56695532232101));
#43241=CARTESIAN_POINT('Ctrl Pts',(-38.9707199974353,21.5430173938286,4.42321205961358));
#43242=CARTESIAN_POINT('Ctrl Pts',(-38.9840145639613,21.5959237595463,4.21330327190672));
#43243=CARTESIAN_POINT('Ctrl Pts',(-39.0953727103553,21.4033245021669,4.54786477253367));
#43244=CARTESIAN_POINT('Ctrl Pts',(-38.9532169021879,21.4993407965975,4.40570896436624));
#43245=CARTESIAN_POINT('Ctrl Pts',(-38.9744729908239,21.5644628247322,4.19421237408121));
#43246=CARTESIAN_POINT('Ctrl Pts',(-39.0452795734807,21.2823889717424,4.49777163565901));
#43247=CARTESIAN_POINT('Ctrl Pts',(-38.9077050083922,21.4174682540841,4.36019707057048));
#43248=CARTESIAN_POINT('Ctrl Pts',(-38.9494357984369,21.5040046541739,4.14411817045999));
#43249=CARTESIAN_POINT('Ctrl Pts',(-39.0142782037993,21.224389488238,4.46677026597765));
#43250=CARTESIAN_POINT('Ctrl Pts',(-38.879467578496,21.379123603316,4.33195964067435));
#43251=CARTESIAN_POINT('Ctrl Pts',(-38.9339408455836,21.4750089453472,4.1131162004694));
#43252=CARTESIAN_POINT('Ctrl Pts',(-38.9415542396192,21.1155503843622,4.39404630179754));
#43253=CARTESIAN_POINT('Ctrl Pts',(-38.8139510374573,21.310227924253,4.26644309963554));
#43254=CARTESIAN_POINT('Ctrl Pts',(-38.8975916626433,21.420595242064,4.04039059104397));
#43255=CARTESIAN_POINT('Ctrl Pts',(-38.8998334160569,21.0647134135968,4.3523254782352));
#43256=CARTESIAN_POINT('Ctrl Pts',(-38.7763600409834,21.279632197814,4.22885210316172));
#43257=CARTESIAN_POINT('Ctrl Pts',(-38.8767383967121,21.3951786071568,3.9986688841259));
#43258=CARTESIAN_POINT('Ctrl Pts',(-38.8072733651297,20.9721533626695,4.259765427308));
#43259=CARTESIAN_POINT('Ctrl Pts',(-38.6940769277129,21.2282175204938,4.14656898989117));
#43260=CARTESIAN_POINT('Ctrl Pts',(-38.8304731995627,21.3488997190596,3.90610655238314));
#43261=CARTESIAN_POINT('Ctrl Pts',(-38.7564363959324,20.930432540155,4.2089284581107));
#43262=CARTESIAN_POINT('Ctrl Pts',(-38.6490267800469,21.207490281533,4.10151884222526));
#43263=CARTESIAN_POINT('Ctrl Pts',(-38.8050624884519,21.3280386002814,3.85526837283333));
#43264=CARTESIAN_POINT('Ctrl Pts',(-38.6475972889203,20.8577085738793,4.10008935109861));
#43265=CARTESIAN_POINT('Ctrl Pts',(-38.5541985142433,21.1773746221138,4.00669057642161));
#43266=CARTESIAN_POINT('Ctrl Pts',(-38.7506581296402,21.2916725623259,3.74642626850048));
#43267=CARTESIAN_POINT('Ctrl Pts',(-38.5895978103376,20.8267072066348,4.04208987251594));
#43268=CARTESIAN_POINT('Ctrl Pts',(-38.504065524732,21.168236619467,3.95655758691019));
#43269=CARTESIAN_POINT('Ctrl Pts',(-38.7216659045744,21.2761685048643,3.68842519451931));
#43270=CARTESIAN_POINT('Ctrl Pts',(-38.468662273206,20.776614066982,3.92115433538435));
#43271=CARTESIAN_POINT('Ctrl Pts',(-38.4018336399262,21.1623409039058,3.85432570210466));
#43272=CARTESIAN_POINT('Ctrl Pts',(-38.6612119130009,21.2511127665618,3.5674858349066));
#43273=CARTESIAN_POINT('Ctrl Pts',(-38.4057291724627,20.7575235195491,3.85822123464104));
#43274=CARTESIAN_POINT('Ctrl Pts',(-38.3494444973764,21.165999727792,3.80193655955489));
#43275=CARTESIAN_POINT('Ctrl Pts',(-38.6297517092871,21.2415616400292,3.50455068049618));
#43276=CARTESIAN_POINT('Ctrl Pts',(-38.2772609486846,20.7319696010243,3.72975301086293));
#43277=CARTESIAN_POINT('Ctrl Pts',(-38.245742257131,21.1861053328133,3.6982343193092));
#43278=CARTESIAN_POINT('Ctrl Pts',(-38.5655282212259,21.22877106589,3.37607766713466));
#43279=CARTESIAN_POINT('Ctrl Pts',(-38.2117264341041,20.7255233616529,3.66421849628246));
#43280=CARTESIAN_POINT('Ctrl Pts',(-38.1942890677528,21.2031338859603,3.64678112993118));
#43281=CARTESIAN_POINT('Ctrl Pts',(-38.5327652990079,21.2255400971374,3.31054054493344));
#43282=CARTESIAN_POINT('Ctrl Pts',(-38.1461904595966,20.7255402022306,3.59868252177487));
#43283=CARTESIAN_POINT('Ctrl Pts',(-38.1462544999649,21.2258119718161,3.59874656214325));
#43284=CARTESIAN_POINT('Ctrl Pts',(-38.5000000005279,21.2255401201565,3.24500105575491));
#43285=CARTESIAN_POINT('',(-39.,21.2045380277352,4.45249206217834));
#43286=CARTESIAN_POINT('Ctrl Pts',(-39.,21.2045380277352,4.45249206217832));
#43287=CARTESIAN_POINT('Ctrl Pts',(-39.,21.3008251669304,4.45249206221659));
#43288=CARTESIAN_POINT('Ctrl Pts',(-39.0000000000062,21.3965734173472,4.43569854959937));
#43289=CARTESIAN_POINT('Ctrl Pts',(-39.0000000000062,21.5319333238365,4.38317740438376));
#43290=CARTESIAN_POINT('Ctrl Pts',(-39.,21.5756326282393,4.36086176771965));
#43291=CARTESIAN_POINT('Ctrl Pts',(-39.,21.6554324370807,4.30861274069145));
#43292=CARTESIAN_POINT('Ctrl Pts',(-39.,21.6909489715919,4.27981443779032));
#43293=CARTESIAN_POINT('Ctrl Pts',(-39.,21.7244769111452,4.24644851929847));
#43294=CARTESIAN_POINT('Ctrl Pts',(-39.,21.7250089648679,4.24591732890776));
#43295=CARTESIAN_POINT('Ctrl Pts',(-39.,21.7255401693197,4.24538528099177));
#43296=CARTESIAN_POINT('Origin',(-38.1470114564408,21.7245991495921,3.59950351982835));
#43297=CARTESIAN_POINT('Ctrl Pts',(-38.1462572731518,20.7255401513379,3.59874933533011));
#43298=CARTESIAN_POINT('Ctrl Pts',(-38.1463046022227,20.2253392826154,3.59879666440107));
#43299=CARTESIAN_POINT('Ctrl Pts',(-38.4999999999868,20.2255401961801,3.24510127662862));
#43300=CARTESIAN_POINT('Ctrl Pts',(-38.2121636970542,20.72555267005,3.66465575923247));
#43301=CARTESIAN_POINT('Ctrl Pts',(-38.1946078611317,20.2481352042117,3.64709992330954));
#43302=CARTESIAN_POINT('Ctrl Pts',(-38.532951213131,20.2255402139663,3.31101031535884));
#43303=CARTESIAN_POINT('Ctrl Pts',(-38.2780681553458,20.7190286310453,3.73056021752408));
#43304=CARTESIAN_POINT('Ctrl Pts',(-38.2463675111531,20.2652184255456,3.69885957333151));
#43305=CARTESIAN_POINT('Ctrl Pts',(-38.565900212778,20.2222723628149,3.37691671021798));
#43306=CARTESIAN_POINT('Ctrl Pts',(-38.407254472938,20.6931736218478,3.85974653511633));
#43307=CARTESIAN_POINT('Ctrl Pts',(-38.3506869574157,20.2852760717712,3.80317901959393));
#43308=CARTESIAN_POINT('Ctrl Pts',(-38.630485454596,20.2093347539537,3.50610658453323));
#43309=CARTESIAN_POINT('Ctrl Pts',(-38.4705347796647,20.6738555693773,3.92302684184305));
#43310=CARTESIAN_POINT('Ctrl Pts',(-38.4033912928499,20.2888369536623,3.85588335502822));
#43311=CARTESIAN_POINT('Ctrl Pts',(-38.6621208762061,20.1996713903363,3.5693884143297));
#43312=CARTESIAN_POINT('Ctrl Pts',(-38.5920768550543,20.6231753537079,4.04456891723265));
#43313=CARTESIAN_POINT('Ctrl Pts',(-38.5061830164427,20.2825955441402,3.95867507862105));
#43314=CARTESIAN_POINT('Ctrl Pts',(-38.7228816482343,20.1743245090983,3.69093332436145));
#43315=CARTESIAN_POINT('Ctrl Pts',(-38.6503355783925,20.5918144601458,4.10282764057083));
#43316=CARTESIAN_POINT('Ctrl Pts',(-38.5565669475031,20.2732153223087,4.00905900968133));
#43317=CARTESIAN_POINT('Ctrl Pts',(-38.7520054127713,20.1586415827856,3.74919322854446));
#43318=CARTESIAN_POINT('Ctrl Pts',(-38.7595684668405,20.518267630651,4.2120605290188));
#43319=CARTESIAN_POINT('Ctrl Pts',(-38.6517811607899,20.2425001122587,4.10427322296828));
#43320=CARTESIAN_POINT('Ctrl Pts',(-38.8066105511857,20.1218652238858,3.85842833570072));
#43321=CARTESIAN_POINT('Ctrl Pts',(-38.8105398978067,20.476083535291,4.26303195998505));
#43322=CARTESIAN_POINT('Ctrl Pts',(-38.696973157022,20.221417076274,4.14946521920037));
#43323=CARTESIAN_POINT('Ctrl Pts',(-38.8320904879864,20.1007726920394,3.90940066031844));
#43324=CARTESIAN_POINT('Ctrl Pts',(-38.9032154807064,20.3825303635642,4.35570754288468));
#43325=CARTESIAN_POINT('Ctrl Pts',(-38.779391773723,20.1692200507405,4.23188383590132));
#43326=CARTESIAN_POINT('Ctrl Pts',(-38.8784172753292,20.0539970424009,4.00207792736665));
#43327=CARTESIAN_POINT('Ctrl Pts',(-38.9449173162986,20.3311636249377,4.39740937847691));
#43328=CARTESIAN_POINT('Ctrl Pts',(-38.8169821824962,20.1381958541655,4.26947424467455));
#43329=CARTESIAN_POINT('Ctrl Pts',(-38.8992628993741,20.028315098226,4.04378041297156));
#43330=CARTESIAN_POINT('Ctrl Pts',(-39.0174313967732,20.221242438767,4.46992345895153));
#43331=CARTESIAN_POINT('Ctrl Pts',(-38.8823308068068,20.0684230182907,4.33482286898507));
#43332=CARTESIAN_POINT('Ctrl Pts',(-38.9355104847273,19.9733589503371,4.1162957034858));
#43333=CARTESIAN_POINT('Ctrl Pts',(-39.0482418325485,20.162690732765,4.50073389472685));
#43334=CARTESIAN_POINT('Ctrl Pts',(-38.9104043915022,20.0296252734399,4.36289645368056));
#43335=CARTESIAN_POINT('Ctrl Pts',(-38.9509114826831,19.9440861441119,4.14710657852245));
#43336=CARTESIAN_POINT('Ctrl Pts',(-39.0977743044738,20.040676419536,4.55026636665211));
#43337=CARTESIAN_POINT('Ctrl Pts',(-38.9554174663834,19.9468798542435,4.40790952856176));
#43338=CARTESIAN_POINT('Ctrl Pts',(-38.9756708542083,19.8830862055383,4.19663982883342));
#43339=CARTESIAN_POINT('Ctrl Pts',(-39.1164951072866,19.9772168492738,4.5689871694649));
#43340=CARTESIAN_POINT('Ctrl Pts',(-38.9725860550694,19.9027778034052,4.42507811724778));
#43341=CARTESIAN_POINT('Ctrl Pts',(-38.9850285683817,19.8513606357535,4.2153608830672));
#43342=CARTESIAN_POINT('Ctrl Pts',(-39.1411196304398,19.8478546030577,4.5936116926181));
#43343=CARTESIAN_POINT('Ctrl Pts',(-38.9950667773803,19.8121580843539,4.44755883955856));
#43344=CARTESIAN_POINT('Ctrl Pts',(-38.9973372985047,19.7866884869349,4.23998577975064));
#43345=CARTESIAN_POINT('Ctrl Pts',(-39.1470227465266,19.7819559842235,4.59951480870491));
#43346=CARTESIAN_POINT('Ctrl Pts',(-39.0004966222791,19.7654220878734,4.45298868445749));
#43347=CARTESIAN_POINT('Ctrl Pts',(-39.0002879913939,19.7537441030219,4.24588897487879));
#43348=CARTESIAN_POINT('Ctrl Pts',(-39.1464021965157,19.7161155308866,4.598894258694));
#43349=CARTESIAN_POINT('Ctrl Pts',(-38.9999293853924,19.7188765600821,4.45242144757075));
#43350=CARTESIAN_POINT('Ctrl Pts',(-38.9999778052401,19.720828532882,4.24526841347127));
#43351=CARTESIAN_POINT('',(-39.,20.2465429544735,4.45249206217834));
#43352=CARTESIAN_POINT('Ctrl Pts',(-38.99999993555,19.7255334503096,4.24539198975394));
#43353=CARTESIAN_POINT('Ctrl Pts',(-38.9999999358904,19.7263281247927,4.24618788058609));
#43354=CARTESIAN_POINT('Ctrl Pts',(-39.,19.7265795127331,4.24646470977148));
#43355=CARTESIAN_POINT('Ctrl Pts',(-39.,19.7599229652764,4.27922044541505));
#43356=CARTESIAN_POINT('Ctrl Pts',(-39.,19.7958071744378,4.30870610834091));
#43357=CARTESIAN_POINT('Ctrl Pts',(-39.,19.8753833962655,4.3608287869574));
#43358=CARTESIAN_POINT('Ctrl Pts',(-39.0000000000057,19.9190457575193,4.38312303219407));
#43359=CARTESIAN_POINT('Ctrl Pts',(-39.0000000000057,20.0543749715938,4.43567530216436));
#43360=CARTESIAN_POINT('Ctrl Pts',(-39.,20.1501887651632,4.45249206221052));
#43361=CARTESIAN_POINT('Ctrl Pts',(-39.,20.2465429544735,4.45249206217833));
#43362=CARTESIAN_POINT('Origin',(-38.1470191121941,19.7264777750522,3.59951117560489));
#43363=CARTESIAN_POINT('Origin',(-42.5,44.0301171154896,-5.44126213566782));
#43364=CARTESIAN_POINT('',(-42.,44.3597593181683,-5.5936318482172));
#43365=CARTESIAN_POINT('Ctrl Pts',(-42.5,44.9368005344368,-5.30952630282034));
#43366=CARTESIAN_POINT('Ctrl Pts',(-42.4693214931018,44.9368005344368,-5.30952630282034));
#43367=CARTESIAN_POINT('Ctrl Pts',(-42.438735398437,44.9334293437634,-5.31107746144859));
#43368=CARTESIAN_POINT('Ctrl Pts',(-42.3572140089482,44.9153607852898,-5.31942199117872));
#43369=CARTESIAN_POINT('Ctrl Pts',(-42.3091583591543,44.8948062033049,-5.32893045402432));
#43370=CARTESIAN_POINT('Ctrl Pts',(-42.2122788312625,44.8339566456983,-5.35744022010934));
#43371=CARTESIAN_POINT('Ctrl Pts',(-42.1666692197098,44.7909059160422,-5.37781140783887));
#43372=CARTESIAN_POINT('Ctrl Pts',(-42.0872212431615,44.6885725964396,-5.42717314417569));
#43373=CARTESIAN_POINT('Ctrl Pts',(-42.0554640174147,44.6277094584301,-5.45704131989472));
#43374=CARTESIAN_POINT('Ctrl Pts',(-42.0117784211058,44.4993327569534,-5.52143090175417));
#43375=CARTESIAN_POINT('Ctrl Pts',(-42.0003916727879,44.431048067398,-5.55638285908588));
#43376=CARTESIAN_POINT('Ctrl Pts',(-42.00000331059,44.3621090125528,-5.5924035000473));
#43377=CARTESIAN_POINT('Ctrl Pts',(-42.,44.3609341213816,-5.59301759162487));
#43378=CARTESIAN_POINT('Ctrl Pts',(-42.,44.3597593181683,-5.59363184821719));
#43379=CARTESIAN_POINT('',(-42.,40.3243975531895,-3.72837640711721));
#43380=CARTESIAN_POINT('',(-42.,44.7270136458737,-5.76338692171892));
#43381=CARTESIAN_POINT('Ctrl Pts',(-42.,40.3243975531895,-3.72837640711721));
#43382=CARTESIAN_POINT('Ctrl Pts',(-42.,40.3240403816243,-3.72705225349016));
#43383=CARTESIAN_POINT('Ctrl Pts',(-42.0000033207593,40.3236830750716,-3.72572813403057));
#43384=CARTESIAN_POINT('Ctrl Pts',(-42.0004541950922,40.2994116461814,-3.63581851390176));
#43385=CARTESIAN_POINT('Ctrl Pts',(-42.0157573105942,40.2747122081378,-3.54683042359109));
#43386=CARTESIAN_POINT('Ctrl Pts',(-42.0728019198682,40.2300648181134,-3.39000514927648));
#43387=CARTESIAN_POINT('Ctrl Pts',(-42.1117195110958,40.2096120486903,-3.31992019235924));
#43388=CARTESIAN_POINT('Ctrl Pts',(-42.2018967293794,40.1784437356806,-3.21492170975514));
#43389=CARTESIAN_POINT('Ctrl Pts',(-42.2479008339596,40.1665637525278,-3.17555129913948));
#43390=CARTESIAN_POINT('Ctrl Pts',(-42.3442168820676,40.1502391476712,-3.12183541479049));
#43391=CARTESIAN_POINT('Ctrl Pts',(-42.3916288820851,40.1450378828802,-3.10489199315609));
#43392=CARTESIAN_POINT('Ctrl Pts',(-42.4610040616797,40.141819202885,-3.09440760124827));
#43393=CARTESIAN_POINT('Ctrl Pts',(-42.4805205119926,40.1413699032525,-3.09294608072936));
#43394=CARTESIAN_POINT('Ctrl Pts',(-42.5,40.1413699032525,-3.09294608072936));
#43395=CARTESIAN_POINT('Origin',(-41.5,40.600288616337,-10.0442405058834));
#43396=CARTESIAN_POINT('',(-42.,40.600288616337,-8.54424050588343));
#43397=CARTESIAN_POINT('Origin',(-42.,40.600288616337,-10.0442405058834));
#43398=CARTESIAN_POINT('Origin',(-41.5,40.600288616337,-8.54424050588343));
#43399=CARTESIAN_POINT('Origin',(-42.5,48.5946168001447,-6.3392739254555));
#43400=CARTESIAN_POINT('',(-42.,44.902988110908,-8.54424050588343));
#43401=CARTESIAN_POINT('Origin',(-42.5,44.902988110908,-8.54424050588343));
#43402=CARTESIAN_POINT('Origin',(-42.,48.5946168001447,-6.3392739254555));
#43403=CARTESIAN_POINT('Origin',(-41.5,34.999999994595,-8.54424050588343));
#43404=CARTESIAN_POINT('Ctrl Pts',(-42.,44.902988110908,-8.54424050588343));
#43405=CARTESIAN_POINT('Ctrl Pts',(-42.,44.9217152275532,-8.55991728673912));
#43406=CARTESIAN_POINT('Ctrl Pts',(-41.99926699101,44.9405761487081,-8.5752530958335));
#43407=CARTESIAN_POINT('Ctrl Pts',(-41.9978770235583,44.9595626840342,-8.59027607382555));
#43408=CARTESIAN_POINT('Ctrl Pts',(-41.9973455416108,44.9668225668177,-8.59602041092588));
#43409=CARTESIAN_POINT('Ctrl Pts',(-41.9967179453166,44.9741007887899,-8.60171894364661));
#43410=CARTESIAN_POINT('Ctrl Pts',(-41.9959982552416,44.9813969174924,-8.60737315034953));
#43411=CARTESIAN_POINT('Ctrl Pts',(-41.9948357632704,44.9931821168892,-8.61650620654169));
#43412=CARTESIAN_POINT('Ctrl Pts',(-41.9934327691023,45.0050141049486,-8.62552362355322));
#43413=CARTESIAN_POINT('Ctrl Pts',(-41.9917995123892,45.0168907527111,-8.63443039129122));
#43414=CARTESIAN_POINT('Ctrl Pts',(-41.9897181963016,45.0320255798673,-8.64578059657901));
#43415=CARTESIAN_POINT('Ctrl Pts',(-41.9872630045812,45.0472328338408,-8.65695106915648));
#43416=CARTESIAN_POINT('Ctrl Pts',(-41.984453841326,45.0625086902382,-8.6679517649698));
#43417=CARTESIAN_POINT('Ctrl Pts',(-41.9801247004088,45.0860499831313,-8.68490470007424));
#43418=CARTESIAN_POINT('Ctrl Pts',(-41.9749549181365,45.1097541946394,-8.70145443366791));
#43419=CARTESIAN_POINT('Ctrl Pts',(-41.9689740864101,45.1336046186899,-8.7176289419902));
#43420=CARTESIAN_POINT('Ctrl Pts',(-41.9679244873749,45.13779022083,-8.72046746832024));
#43421=CARTESIAN_POINT('Ctrl Pts',(-41.966849894493,45.1419803414508,-8.72329444248294));
#43422=CARTESIAN_POINT('Ctrl Pts',(-41.9657504515975,45.1461749072067,-8.72611001084982));
#43423=CARTESIAN_POINT('Ctrl Pts',(-41.9642673716375,45.1518331150488,-8.72990803713926));
#43424=CARTESIAN_POINT('Ctrl Pts',(-41.9627388825222,45.1574993790093,-8.73368527854127));
#43425=CARTESIAN_POINT('Ctrl Pts',(-41.9611650123427,45.1631734698631,-8.73744204070059));
#43426=CARTESIAN_POINT('Ctrl Pts',(-41.9607679814752,45.1646048390084,-8.73838973674212));
#43427=CARTESIAN_POINT('Ctrl Pts',(-41.9603681175447,45.1660365084498,-8.73933599886251));
#43428=CARTESIAN_POINT('Ctrl Pts',(-41.9599653926612,45.1674685814126,-8.74028090364377));
#43429=CARTESIAN_POINT('Ctrl Pts',(-41.9579598774666,45.1746001101675,-8.74498640105417));
#43430=CARTESIAN_POINT('Ctrl Pts',(-41.955880829506,45.1817504452265,-8.74966397918282));
#43431=CARTESIAN_POINT('Ctrl Pts',(-41.9537330860392,45.1889019974108,-8.75430308378186));
#43432=CARTESIAN_POINT('Ctrl Pts',(-41.953335044313,45.1902273960073,-8.75516284996496));
#43433=CARTESIAN_POINT('Ctrl Pts',(-41.9529347426312,45.1915525258364,-8.75602109581612));
#43434=CARTESIAN_POINT('Ctrl Pts',(-41.9525321577263,45.1928774682436,-8.75687788307363));
#43435=CARTESIAN_POINT('Ctrl Pts',(-41.948591555106,45.2058463388042,-8.7652643329151));
#43436=CARTESIAN_POINT('Ctrl Pts',(-41.9444306648395,45.2188024265432,-8.7735143558228));
#43437=CARTESIAN_POINT('Ctrl Pts',(-41.9400504090668,45.231742825263,-8.78163392930062));
#43438=CARTESIAN_POINT('Ctrl Pts',(-41.9377366778172,45.238578180652,-8.78592283658468));
#43439=CARTESIAN_POINT('Ctrl Pts',(-41.9353619641797,45.2454093037384,-8.79017544543466));
#43440=CARTESIAN_POINT('Ctrl Pts',(-41.9329257017781,45.2522353739754,-8.79439229947627));
#43441=CARTESIAN_POINT('Ctrl Pts',(-41.9258772129349,45.2719842646844,-8.80659231891841));
#43442=CARTESIAN_POINT('Ctrl Pts',(-41.9183136346165,45.2916915246547,-8.81849347201985));
#43443=CARTESIAN_POINT('Ctrl Pts',(-41.910217493462,45.3113410897915,-8.83011052782056));
#43444=CARTESIAN_POINT('Ctrl Pts',(-41.9094845927378,45.3131198607202,-8.83116215827605));
#43445=CARTESIAN_POINT('Ctrl Pts',(-41.9087473256333,45.3148981526486,-8.83221145929809));
#43446=CARTESIAN_POINT('Ctrl Pts',(-41.9080056754341,45.3166759591509,-8.83325844445048));
#43447=CARTESIAN_POINT('Ctrl Pts',(-41.9005545315738,45.3345370640473,-8.84377719978644));
#43448=CARTESIAN_POINT('Ctrl Pts',(-41.8926617593855,45.3523499135917,-8.85406244540301));
#43449=CARTESIAN_POINT('Ctrl Pts',(-41.8842899617511,45.3700942133327,-8.86411913234023));
#43450=CARTESIAN_POINT('Ctrl Pts',(-41.8795553606888,45.380129355613,-8.86980660864286));
#43451=CARTESIAN_POINT('Ctrl Pts',(-41.8746675657325,45.3901422940905,-8.87542085810376));
#43452=CARTESIAN_POINT('Ctrl Pts',(-41.8696184988485,45.4001301957612,-8.8809631889771));
#43453=CARTESIAN_POINT('Ctrl Pts',(-41.8648510912,45.4095609281936,-8.88619634417246));
#43454=CARTESIAN_POINT('Ctrl Pts',(-41.8599393529639,45.4189689378561,-8.89136515656763));
#43455=CARTESIAN_POINT('Ctrl Pts',(-41.8548730788033,45.4283492718046,-8.89646937487582));
#43456=CARTESIAN_POINT('Ctrl Pts',(-41.8525827714795,45.4325898333813,-8.89877683558625));
#43457=CARTESIAN_POINT('Ctrl Pts',(-41.8502613638914,45.4368238606404,-8.90107060968825));
#43458=CARTESIAN_POINT('Ctrl Pts',(-41.8479069515496,45.4410525278538,-8.90335156539488));
#43459=CARTESIAN_POINT('Ctrl Pts',(-41.8448994391838,45.4464542022802,-8.90626524469058));
#43460=CARTESIAN_POINT('Ctrl Pts',(-41.8418352055889,45.4518516438432,-8.90916037727808));
#43461=CARTESIAN_POINT('Ctrl Pts',(-41.8387233732327,45.4572239437181,-8.91202638213873));
#43462=CARTESIAN_POINT('Ctrl Pts',(-41.8379490304162,45.4585607772424,-8.91273955367935));
#43463=CARTESIAN_POINT('Ctrl Pts',(-41.8371715840211,45.4598963309502,-8.91345106303885));
#43464=CARTESIAN_POINT('Ctrl Pts',(-41.8363912062383,45.4612302114177,-8.91416070858338));
#43465=CARTESIAN_POINT('Ctrl Pts',(-41.8325053766855,45.4678721638856,-8.91769433254054));
#43466=CARTESIAN_POINT('Ctrl Pts',(-41.8285427447655,45.4744804257973,-8.92118599460502));
#43467=CARTESIAN_POINT('Ctrl Pts',(-41.8245000582813,45.4810503220176,-8.92463465959361));
#43468=CARTESIAN_POINT('Ctrl Pts',(-41.8235377795384,45.4826141512931,-8.92545554368212));
#43469=CARTESIAN_POINT('Ctrl Pts',(-41.8225709901412,45.4841758442149,-8.92627400994534));
#43470=CARTESIAN_POINT('Ctrl Pts',(-41.8215996339254,45.4857353191729,-8.92709003533626));
#43471=CARTESIAN_POINT('Ctrl Pts',(-41.8098562016529,45.5045889469695,-8.93695556021317));
#43472=CARTESIAN_POINT('Ctrl Pts',(-41.7974460451304,45.5231265694832,-8.9464672375347));
#43473=CARTESIAN_POINT('Ctrl Pts',(-41.7842200516186,45.5412462580514,-8.95560374436775));
#43474=CARTESIAN_POINT('Ctrl Pts',(-41.7805875545163,45.5462228003549,-8.95811307076099));
#43475=CARTESIAN_POINT('Ctrl Pts',(-41.7768935421867,45.5511671810966,-8.9605938588154));
#43476=CARTESIAN_POINT('Ctrl Pts',(-41.7731337798956,45.5560776923919,-8.96304587628849));
#43477=CARTESIAN_POINT('Ctrl Pts',(-41.7632041736153,45.5690464494629,-8.96952170274114));
#43478=CARTESIAN_POINT('Ctrl Pts',(-41.75281858549,45.5817832043924,-8.97579859997023));
#43479=CARTESIAN_POINT('Ctrl Pts',(-41.7418680590367,45.5942087950184,-8.98185051649874));
#43480=CARTESIAN_POINT('Ctrl Pts',(-41.7343196332262,45.6027740132655,-8.98602222852756));
#43481=CARTESIAN_POINT('Ctrl Pts',(-41.7265018645057,45.6111916179132,-8.99008727610328));
#43482=CARTESIAN_POINT('Ctrl Pts',(-41.7183666093141,45.6194329653189,-8.99403617303334));
#43483=CARTESIAN_POINT('Ctrl Pts',(-41.7172568243484,45.6205572230382,-8.99457486866619));
#43484=CARTESIAN_POINT('Ctrl Pts',(-41.7161408581521,45.6216784231438,-8.99511152314756));
#43485=CARTESIAN_POINT('Ctrl Pts',(-41.7150187648596,45.6227962934492,-8.99564601178507));
#43486=CARTESIAN_POINT('Ctrl Pts',(-41.7120281175915,45.6257756854456,-8.99707055196744));
#43487=CARTESIAN_POINT('Ctrl Pts',(-41.70900015992,45.6287243075931,-8.9984763094132));
#43488=CARTESIAN_POINT('Ctrl Pts',(-41.7059403448518,45.6316334313436,-8.99985935990986));
#43489=CARTESIAN_POINT('Ctrl Pts',(-41.703763557296,45.6337030153665,-9.0008432779059));
#43490=CARTESIAN_POINT('Ctrl Pts',(-41.7015691398645,45.6357540055558,-9.0018163966474));
#43491=CARTESIAN_POINT('Ctrl Pts',(-41.6993578766797,45.6377842033898,-9.0027777857267));
#43492=CARTESIAN_POINT('Ctrl Pts',(-41.6972946362417,45.6396784990562,-9.00367481907793));
#43493=CARTESIAN_POINT('Ctrl Pts',(-41.6952158521099,45.641555574399,-9.00456206138067));
#43494=CARTESIAN_POINT('Ctrl Pts',(-41.6931210371443,45.6434146521169,-9.00543924012301));
#43495=CARTESIAN_POINT('Ctrl Pts',(-41.6899079491655,45.6462661594648,-9.00678468233083));
#43496=CARTESIAN_POINT('Ctrl Pts',(-41.6866574181238,45.6490750873074,-9.00810634480957));
#43497=CARTESIAN_POINT('Ctrl Pts',(-41.683367132931,45.6518388544561,-9.00940337473763));
#43498=CARTESIAN_POINT('Ctrl Pts',(-41.6777690417215,45.6565411278684,-9.01161014145035));
#43499=CARTESIAN_POINT('Ctrl Pts',(-41.6720560193021,45.6611131196413,-9.01374581468396));
#43500=CARTESIAN_POINT('Ctrl Pts',(-41.6662154610016,45.665538373007,-9.01580446686645));
#43501=CARTESIAN_POINT('Ctrl Pts',(-41.6610327553656,45.669465186914,-9.01763124227383));
#43502=CARTESIAN_POINT('Ctrl Pts',(-41.6557496367553,45.6732762891216,-9.01939737122132));
#43503=CARTESIAN_POINT('Ctrl Pts',(-41.6503549411668,45.6769591907994,-9.02109833759718));
#43504=CARTESIAN_POINT('Ctrl Pts',(-41.6460969718104,45.6798660614893,-9.02244089021871));
#43505=CARTESIAN_POINT('Ctrl Pts',(-41.6417694968915,45.6826930774886,-9.02374285555159));
#43506=CARTESIAN_POINT('Ctrl Pts',(-41.6373663141285,45.6854319287458,-9.02500100931356));
#43507=CARTESIAN_POINT('Ctrl Pts',(-41.6304024527032,45.6897635637577,-9.0269908446036));
#43508=CARTESIAN_POINT('Ctrl Pts',(-41.6232495947523,45.693875048068,-9.02887130000535));
#43509=CARTESIAN_POINT('Ctrl Pts',(-41.6158751354701,45.6977294272706,-9.03062816298464));
#43510=CARTESIAN_POINT('Ctrl Pts',(-41.6126791934946,45.6993998375084,-9.03138955197952));
#43511=CARTESIAN_POINT('Ctrl Pts',(-41.6094415604145,45.7010217444016,-9.03212762696971));
#43512=CARTESIAN_POINT('Ctrl Pts',(-41.6061592594077,45.7025911406349,-9.03284077776707));
#43513=CARTESIAN_POINT('Ctrl Pts',(-41.6034837334275,45.703870414043,-9.03342209358249));
#43514=CARTESIAN_POINT('Ctrl Pts',(-41.6007783569267,45.7051148711038,-9.03398688253731));
#43515=CARTESIAN_POINT('Ctrl Pts',(-41.5980413638051,45.7063221317373,-9.03453418418577));
#43516=CARTESIAN_POINT('Ctrl Pts',(-41.5980019984786,45.706339495394,-9.0345420558563));
#43517=CARTESIAN_POINT('Ctrl Pts',(-41.5979626261383,45.7063568515059,-9.03454992397607));
#43518=CARTESIAN_POINT('Ctrl Pts',(-41.5979232468274,45.7063742000469,-9.03455778853368));
#43519=CARTESIAN_POINT('Ctrl Pts',(-41.5951459020883,45.707597758257,-9.03511246019182));
#43520=CARTESIAN_POINT('Ctrl Pts',(-41.5923316176566,45.7087845416927,-9.03564980619242));
#43521=CARTESIAN_POINT('Ctrl Pts',(-41.5895072796806,45.7099207110941,-9.03616371707989));
#43522=CARTESIAN_POINT('Ctrl Pts',(-41.5893316400524,45.7099913670754,-9.03619567611524));
#43523=CARTESIAN_POINT('Ctrl Pts',(-41.5891559504675,45.7100618323782,-9.03622754675872));
#43524=CARTESIAN_POINT('Ctrl Pts',(-41.5889802150548,45.7101321047206,-9.03625932801202));
#43525=CARTESIAN_POINT('Ctrl Pts',(-41.5859677707848,45.7113367083446,-9.03680412005438));
#43526=CARTESIAN_POINT('Ctrl Pts',(-41.5829376777973,45.7124865784167,-9.03732353620516));
#43527=CARTESIAN_POINT('Ctrl Pts',(-41.5798897584861,45.7135797785149,-9.03781686926509));
#43528=CARTESIAN_POINT('Ctrl Pts',(-41.5773971702446,45.7144737974938,-9.03822031701379));
#43529=CARTESIAN_POINT('Ctrl Pts',(-41.5748926681928,45.7153299965749,-9.03860642538735));
#43530=CARTESIAN_POINT('Ctrl Pts',(-41.5723761485838,45.7161472393841,-9.03897472984346));
#43531=CARTESIAN_POINT('Ctrl Pts',(-41.5637163275296,45.7189595268228,-9.04024213529982));
#43532=CARTESIAN_POINT('Ctrl Pts',(-41.5549125428017,45.7213117106978,-9.04129922850373));
#43533=CARTESIAN_POINT('Ctrl Pts',(-41.5459499111192,45.7231558414443,-9.04212652536896));
#43534=CARTESIAN_POINT('Ctrl Pts',(-41.5412041320697,45.7241323221668,-9.04256458511188));
#43535=CARTESIAN_POINT('Ctrl Pts',(-41.5364138582115,45.7249662131444,-9.04293815642914));
#43536=CARTESIAN_POINT('Ctrl Pts',(-41.5315766337177,45.7256494547312,-9.04324396659871));
#43537=CARTESIAN_POINT('Ctrl Pts',(-41.5284280862249,45.7260941764074,-9.04344301831605));
#43538=CARTESIAN_POINT('Ctrl Pts',(-41.5252569314378,45.726475340385,-9.04361348204527));
#43539=CARTESIAN_POINT('Ctrl Pts',(-41.5220695810843,45.7267898067094,-9.043754052548));
#43540=CARTESIAN_POINT('Ctrl Pts',(-41.5209058550529,45.7269046207735,-9.04380537591542));
#43541=CARTESIAN_POINT('Ctrl Pts',(-41.5197405027109,45.727010497462,-9.04385269377214));
#43542=CARTESIAN_POINT('Ctrl Pts',(-41.5185746234031,45.7271072918289,-9.04389594637392));
#43543=CARTESIAN_POINT('Ctrl Pts',(-41.5145270192726,45.727443334571,-9.04404610720827));
#43544=CARTESIAN_POINT('Ctrl Pts',(-41.5104730713073,45.7276699868093,-9.04414730118872));
#43545=CARTESIAN_POINT('Ctrl Pts',(-41.5064127138504,45.7277864292123,-9.04419938129327));
#43546=CARTESIAN_POINT('Ctrl Pts',(-41.5042769250897,45.7278476790845,-9.04422677595079));
#43547=CARTESIAN_POINT('Ctrl Pts',(-41.5021393585781,45.7278783937086,-9.04424052634312));
#43548=CARTESIAN_POINT('Ctrl Pts',(-41.5000000000005,45.7278784053971,-9.04424054928485));
#43549=CARTESIAN_POINT('',(-42.,34.999999994595,-8.54424050588343));
#43550=CARTESIAN_POINT('Ctrl Pts',(-42.,44.902988110908,-8.54424050588343));
#43551=CARTESIAN_POINT('Ctrl Pts',(-42.,45.3322472608192,-8.28784904304297));
#43552=CARTESIAN_POINT('Ctrl Pts',(-42.5,45.3322472608192,-8.28784904304297));
#43553=CARTESIAN_POINT('Ctrl Pts',(-42.,44.9286604045246,-8.56573120990982));
#43554=CARTESIAN_POINT('Ctrl Pts',(-42.0108999708817,45.3453293288621,-8.30975148851287));
#43555=CARTESIAN_POINT('Ctrl Pts',(-42.4999999895151,45.3549342921599,-8.32583242860273));
#43556=CARTESIAN_POINT('Ctrl Pts',(-41.9986214707204,44.9548030624169,-8.58676399861629));
#43557=CARTESIAN_POINT('Ctrl Pts',(-42.0202495830765,45.3594232689745,-8.33310036955195));
#43558=CARTESIAN_POINT('Ctrl Pts',(-42.497242938469,45.3780372174225,-8.36300684416903));
#43559=CARTESIAN_POINT('Ctrl Pts',(-41.9933750391373,45.0079907648268,-8.6279823069976));
#43560=CARTESIAN_POINT('Ctrl Pts',(-42.0351385937246,45.3894870614958,-8.38178650312646));
#43561=CARTESIAN_POINT('Ctrl Pts',(-42.4867500812463,45.4250403043614,-8.43585780778609));
#43562=CARTESIAN_POINT('Ctrl Pts',(-41.9895059097455,45.0350362147751,-8.64816784262251));
#43563=CARTESIAN_POINT('Ctrl Pts',(-42.0407565860507,45.4054076846729,-8.40706640877658));
#43564=CARTESIAN_POINT('Ctrl Pts',(-42.4790118184447,45.4489409335363,-8.47153456853107));
#43565=CARTESIAN_POINT('Ctrl Pts',(-41.979401772684,45.0899811643642,-8.68773568818862));
#43566=CARTESIAN_POINT('Ctrl Pts',(-42.04788943116,45.4390859958032,-8.45907111556724));
#43567=CARTESIAN_POINT('Ctrl Pts',(-42.4588035464137,45.4974969364344,-8.54146843493532));
#43568=CARTESIAN_POINT('Ctrl Pts',(-41.9731666254647,45.1178808703317,-8.70711789767085));
#43569=CARTESIAN_POINT('Ctrl Pts',(-42.0494921140164,45.4567992240739,-8.48575669704656));
#43570=CARTESIAN_POINT('Ctrl Pts',(-42.4463332516214,45.5221524896634,-8.57572536395869));
#43571=CARTESIAN_POINT('Ctrl Pts',(-41.9638964057752,45.1532484070924,-8.73085804517682));
#43572=CARTESIAN_POINT('Ctrl Pts',(-42.0487386127422,45.4802136676926,-8.51997409646917));
#43573=CARTESIAN_POINT('Ctrl Pts',(-42.4277928113774,45.5534075226671,-8.61768469375029));
#43574=CARTESIAN_POINT('Ctrl Pts',(-41.9619682484332,45.1603465096623,-8.7355816459985));
#43575=CARTESIAN_POINT('Ctrl Pts',(-42.0484549927054,45.4849117932795,-8.52679133797057));
#43576=CARTESIAN_POINT('Ctrl Pts',(-42.4239364971452,45.5596802642686,-8.62603338389302));
#43577=CARTESIAN_POINT('Ctrl Pts',(-41.9579625363262,45.1745906511032,-8.74498016260993));
#43578=CARTESIAN_POINT('Ctrl Pts',(-42.0476113931016,45.4944127529898,-8.54047636109722));
#43579=CARTESIAN_POINT('Ctrl Pts',(-42.4159250723737,45.5722681103951,-8.64264471521523));
#43580=CARTESIAN_POINT('Ctrl Pts',(-41.955882303473,45.1817455281307,-8.74966079550314));
#43581=CARTESIAN_POINT('Ctrl Pts',(-42.0470519527415,45.4992210657315,-8.54735241762345));
#43582=CARTESIAN_POINT('Ctrl Pts',(-42.411764606457,45.5785910245723,-8.65091746194013));
#43583=CARTESIAN_POINT('Ctrl Pts',(-41.9494346473223,45.2032149228718,-8.76358766865384));
#43584=CARTESIAN_POINT('Ctrl Pts',(-42.0449628041206,45.5137178535233,-8.56792941843968));
#43585=CARTESIAN_POINT('Ctrl Pts',(-42.3988692956227,45.5975639789771,-8.6755324004288));
#43586=CARTESIAN_POINT('Ctrl Pts',(-41.9448722632192,45.2174978104266,-8.77269577610381));
#43587=CARTESIAN_POINT('Ctrl Pts',(-42.0430249734493,45.5235278259453,-8.58165311177667));
#43588=CARTESIAN_POINT('Ctrl Pts',(-42.3897445259251,45.6101860644684,-8.69163045108915));
#43589=CARTESIAN_POINT('Ctrl Pts',(-41.9304066859268,45.2602328103821,-8.79951026319421));
#43590=CARTESIAN_POINT('Ctrl Pts',(-42.0356031360407,45.5531189722808,-8.62243545445269));
#43591=CARTESIAN_POINT('Ctrl Pts',(-42.3608133728757,45.6479518801124,-8.73902349739317));
#43592=CARTESIAN_POINT('Ctrl Pts',(-41.9197290595943,45.2885738141815,-8.81670858590767));
#43593=CARTESIAN_POINT('Ctrl Pts',(-42.0285011256322,45.573363377834,-8.64954189109913));
#43594=CARTESIAN_POINT('Ctrl Pts',(-42.3394581198824,45.6729974161304,-8.76942053466115));
#43595=CARTESIAN_POINT('Ctrl Pts',(-41.8962822187091,45.3447779229183,-8.84980840543283));
#43596=CARTESIAN_POINT('Ctrl Pts',(-42.0098501467087,45.6143697759043,-8.70284461529763));
#43597=CARTESIAN_POINT('Ctrl Pts',(-42.2925644367244,45.7226661655264,-8.8279225385782));
#43598=CARTESIAN_POINT('Ctrl Pts',(-41.8835140806194,45.3726424029527,-8.86571009100462));
#43599=CARTESIAN_POINT('Ctrl Pts',(-41.9983779043733,45.6351418297266,-8.72908283607111));
#43600=CARTESIAN_POINT('Ctrl Pts',(-42.2670281635762,45.7472905876327,-8.85602784747157));
#43601=CARTESIAN_POINT('Ctrl Pts',(-41.862670707963,45.4138740921654,-8.88858973796334));
#43602=CARTESIAN_POINT('Ctrl Pts',(-41.9776044328624,45.6665359773409,-8.76763025951353));
#43603=CARTESIAN_POINT('Ctrl Pts',(-42.2253414147564,45.7837278959388,-8.8964662890298));
#43604=CARTESIAN_POINT('Ctrl Pts',(-41.8554398788958,45.427522950843,-8.89605366242561));
#43605=CARTESIAN_POINT('Ctrl Pts',(-41.9701420076706,45.6769743994332,-8.78026942647067));
#43606=CARTESIAN_POINT('Ctrl Pts',(-42.2108797593804,45.795789676984,-8.90965834491112));
#43607=CARTESIAN_POINT('Ctrl Pts',(-41.8441404753721,45.4478172893659,-8.90700052899381));
#43608=CARTESIAN_POINT('Ctrl Pts',(-41.958022565088,45.6926462815954,-8.79898741435063));
#43609=CARTESIAN_POINT('Ctrl Pts',(-42.1882809499499,45.8137242094849,-8.92900629222498));
#43610=CARTESIAN_POINT('Ctrl Pts',(-41.8402940153966,45.4545592291316,-8.91061164426722));
#43611=CARTESIAN_POINT('Ctrl Pts',(-41.9538372921188,45.6978624661921,-8.80517489813451));
#43612=CARTESIAN_POINT('Ctrl Pts',(-42.1805880309734,45.8196822021074,-8.93538873003764));
#43613=CARTESIAN_POINT('Ctrl Pts',(-41.8324883720422,45.4679011401808,-8.91770979566791));
#43614=CARTESIAN_POINT('Ctrl Pts',(-41.9452093359132,45.7082222863744,-8.81738175445068));
#43615=CARTESIAN_POINT('Ctrl Pts',(-42.1649767439042,45.8314727289465,-8.9479342988573));
#43616=CARTESIAN_POINT('Ctrl Pts',(-41.8285250186428,45.4745089647429,-8.92120111745386));
#43617=CARTESIAN_POINT('Ctrl Pts',(-41.940763007093,45.7133726477466,-8.82340956419523));
#43618=CARTESIAN_POINT('Ctrl Pts',(-42.1570500375643,45.8373122010236,-8.95410500834317));
#43619=CARTESIAN_POINT('Ctrl Pts',(-41.8083998462294,45.5072149631162,-8.93836914430218));
#43620=CARTESIAN_POINT('Ctrl Pts',(-41.9179983851406,45.7388018091337,-8.85297773751299));
#43621=CARTESIAN_POINT('Ctrl Pts',(-42.1167996913393,45.8662151783001,-8.98444849433146));
#43622=CARTESIAN_POINT('Ctrl Pts',(-41.7913199828142,45.5323245258358,-8.95118532573511));
#43623=CARTESIAN_POINT('Ctrl Pts',(-41.8975757846378,45.7587513033878,-8.87555470746898));
#43624=CARTESIAN_POINT('Ctrl Pts',(-42.0826399682652,45.8884050213045,-9.00710035766719));
#43625=CARTESIAN_POINT('Ctrl Pts',(-41.7549472623746,45.5798301722945,-8.97490663201676));
#43626=CARTESIAN_POINT('Ctrl Pts',(-41.8522755408233,45.7968273270403,-8.91768065668701));
#43627=CARTESIAN_POINT('Ctrl Pts',(-42.0098945221124,45.9303867584722,-9.04902637713643));
#43628=CARTESIAN_POINT('Ctrl Pts',(-41.7356587556976,45.6022335718975,-8.98581453285689));
#43629=CARTESIAN_POINT('Ctrl Pts',(-41.827418348961,45.8150217309514,-8.9373171564491));
#43630=CARTESIAN_POINT('Ctrl Pts',(-41.9713175153897,45.9501851085395,-9.06830547181726));
#43631=CARTESIAN_POINT('Ctrl Pts',(-41.7098586873126,45.6279367771953,-8.99810391954615));
#43632=CARTESIAN_POINT('Ctrl Pts',(-41.7930929437521,45.8361032447929,-8.95964586975483));
#43633=CARTESIAN_POINT('Ctrl Pts',(-41.9197173736266,45.9728995709431,-9.09002623703225));
#43634=CARTESIAN_POINT('Ctrl Pts',(-41.704632773787,45.6329411844467,-9.00048442311758));
#43635=CARTESIAN_POINT('Ctrl Pts',(-41.7861251546753,45.8401999741684,-8.9639626962812));
#43636=CARTESIAN_POINT('Ctrl Pts',(-41.9092655478991,45.9773220695307,-9.09423364209421));
#43637=CARTESIAN_POINT('Ctrl Pts',(-41.6940829685631,45.6426271938172,-9.00507115312237));
#43638=CARTESIAN_POINT('Ctrl Pts',(-41.7719775499116,45.8481422955614,-8.97229352456195));
#43639=CARTESIAN_POINT('Ctrl Pts',(-41.8881659368007,45.9858817996664,-9.10234041840881));
#43640=CARTESIAN_POINT('Ctrl Pts',(-41.6887533114059,45.6473145875886,-9.00728014401976));
#43641=CARTESIAN_POINT('Ctrl Pts',(-41.76478941984,45.8519939510722,-8.97631403485392));
#43642=CARTESIAN_POINT('Ctrl Pts',(-41.877506623199,45.9900241467431,-9.10624468388211));
#43643=CARTESIAN_POINT('Ctrl Pts',(-41.6725947699906,45.6608873717108,-9.01364983853488));
#43644=CARTESIAN_POINT('Ctrl Pts',(-41.7429102615715,45.8631498532122,-8.98790974948757));
#43645=CARTESIAN_POINT('Ctrl Pts',(-41.8451895392067,46.0020187014886,-9.11750274457941));
#43646=CARTESIAN_POINT('Ctrl Pts',(-41.6615966611876,45.6692843712125,-9.01755378461365));
#43647=CARTESIAN_POINT('Ctrl Pts',(-41.7278472754948,45.8700901815488,-8.9950561303503));
#43648=CARTESIAN_POINT('Ctrl Pts',(-41.8231933233325,46.0094393040033,-9.12440274854059));
#43649=CARTESIAN_POINT('Ctrl Pts',(-41.639113172241,45.6846338528735,-9.02464290600063));
#43650=CARTESIAN_POINT('Ctrl Pts',(-41.6968062378558,45.8827994607731,-9.0080542913267));
#43651=CARTESIAN_POINT('Ctrl Pts',(-41.7782263435246,46.0230039638273,-9.13693235132219));
#43652=CARTESIAN_POINT('Ctrl Pts',(-41.6276278973201,45.691586658138,-9.02782822994433));
#43653=CARTESIAN_POINT('Ctrl Pts',(-41.6808195592107,45.8885783031742,-9.01391663064739));
#43654=CARTESIAN_POINT('Ctrl Pts',(-41.7552557956688,46.0291483018663,-9.14256223432903));
#43655=CARTESIAN_POINT('Ctrl Pts',(-41.6099987545451,45.7008008118369,-9.03202812950479));
#43656=CARTESIAN_POINT('Ctrl Pts',(-41.6561159186992,45.8962508251284,-9.02165960285725));
#43657=CARTESIAN_POINT('Ctrl Pts',(-41.7199975085757,46.037291043381,-9.14998530576052));
#43658=CARTESIAN_POINT('Ctrl Pts',(-41.6040554010528,45.7036694039868,-9.03333158983249));
#43659=CARTESIAN_POINT('Ctrl Pts',(-41.6477683894613,45.8986408027904,-9.02406393261697));
#43660=CARTESIAN_POINT('Ctrl Pts',(-41.7081108026102,46.0398260776494,-9.15228910096591));
#43661=CARTESIAN_POINT('Ctrl Pts',(-41.5950343440379,45.707648490221,-9.03513548159103));
#43662=CARTESIAN_POINT('Ctrl Pts',(-41.6350621829909,45.9019591498723,-9.0273943698628));
#43663=CARTESIAN_POINT('Ctrl Pts',(-41.6900686878235,46.0433424799017,-9.15547737091504));
#43664=CARTESIAN_POINT('Ctrl Pts',(-41.5920068986027,45.7089217810477,-9.03571196085561));
#43665=CARTESIAN_POINT('Ctrl Pts',(-41.6307939033919,45.9030212106372,-9.02845888268938));
#43666=CARTESIAN_POINT('Ctrl Pts',(-41.6840137971755,46.0444677133423,-9.1564962658135));
#43667=CARTESIAN_POINT('Ctrl Pts',(-41.5859535254763,45.7113423972445,-9.03680669625905));
#43668=CARTESIAN_POINT('Ctrl Pts',(-41.6222498275285,45.9050409290163,-9.0304810243379));
#43669=CARTESIAN_POINT('Ctrl Pts',(-41.6719070509825,46.0466068628566,-9.15843114693368));
#43670=CARTESIAN_POINT('Ctrl Pts',(-41.5829233752423,45.7124917049892,-9.03732585120345));
#43671=CARTESIAN_POINT('Ctrl Pts',(-41.6179678487693,45.9060003613735,-9.03144043622865));
#43672=CARTESIAN_POINT('Ctrl Pts',(-41.6658467504665,46.047622529863,-9.15934872320473));
#43673=CARTESIAN_POINT('Ctrl Pts',(-41.5556208222111,45.7222843539839,-9.04174501411847));
#43674=CARTESIAN_POINT('Ctrl Pts',(-41.5794217634366,45.9141617518149,-9.03959362376309));
#43675=CARTESIAN_POINT('Ctrl Pts',(-41.6112416445666,46.0562765000394,-9.16715933617831));
#43676=CARTESIAN_POINT('Ctrl Pts',(-41.5311308076983,45.7270775602764,-9.04388233509682));
#43677=CARTESIAN_POINT('Ctrl Pts',(-41.5444292326109,45.9181968905741,-9.04357633437154));
#43678=CARTESIAN_POINT('Ctrl Pts',(-41.5622616154321,46.0605123555124,-9.17093692978999));
#43679=CARTESIAN_POINT('Ctrl Pts',(-41.4940536667479,45.7281408512266,-9.04435790439379));
#43680=CARTESIAN_POINT('Ctrl Pts',(-41.4915166863813,45.9190876289001,-9.04445814124235));
#43681=CARTESIAN_POINT('Ctrl Pts',(-41.488107333478,46.0614520081263,-9.17177746703914));
#43682=CARTESIAN_POINT('Ctrl Pts',(-41.4816374541537,45.7274728039395,-9.04405951499495));
#43683=CARTESIAN_POINT('Ctrl Pts',(-41.4737840688501,45.9185271854623,-9.04390407525488));
#43684=CARTESIAN_POINT('Ctrl Pts',(-41.4632749081632,46.0608616409463,-9.17125008419945));
#43685=CARTESIAN_POINT('Ctrl Pts',(-41.4629246490349,45.7248907522696,-9.0429031920658));
#43686=CARTESIAN_POINT('Ctrl Pts',(-41.4471201591405,45.9163657707925,-9.04176155338066));
#43687=CARTESIAN_POINT('Ctrl Pts',(-41.425849298142,46.0585798274846,-9.16920634795539));
#43688=CARTESIAN_POINT('Ctrl Pts',(-41.4566624705733,45.7237626947943,-9.04239772264832));
#43689=CARTESIAN_POINT('Ctrl Pts',(-41.4382011712065,45.9154212255412,-9.04082471749996));
#43690=CARTESIAN_POINT('Ctrl Pts',(-41.4133249413372,46.0575829397824,-9.16831295915316));
#43691=CARTESIAN_POINT('Ctrl Pts',(-41.4442731608293,45.7210143399589,-9.04116431640955));
#43692=CARTESIAN_POINT('Ctrl Pts',(-41.4205799986544,45.9131217963581,-9.03854049004602));
#43693=CARTESIAN_POINT('Ctrl Pts',(-41.388546321468,46.0551541607308,-9.16613298912151));
#43694=CARTESIAN_POINT('Ctrl Pts',(-41.4381262046785,45.7193922594189,-9.0404355851954));
#43695=CARTESIAN_POINT('Ctrl Pts',(-41.4118473895139,45.911764846025,-9.03719104617774));
#43696=CARTESIAN_POINT('Ctrl Pts',(-41.3762524095784,46.053720694625,-9.16484499548513));
#43697=CARTESIAN_POINT('Ctrl Pts',(-41.407621134817,45.7100931492939,-9.0362495685661));
#43698=CARTESIAN_POINT('Ctrl Pts',(-41.3685291843857,45.9039820475746,-9.02943568588035));
#43699=CARTESIAN_POINT('Ctrl Pts',(-41.3152422687481,46.0455028751849,-9.15744646291901));
#43700=CARTESIAN_POINT('Ctrl Pts',(-41.3839484100396,45.6988653534475,-9.03117626479338));
#43701=CARTESIAN_POINT('Ctrl Pts',(-41.3351481982956,45.8945772852277,-9.02002671647569));
#43702=CARTESIAN_POINT('Ctrl Pts',(-41.2678968207294,46.0355806396204,-9.14847968289344));
#43703=CARTESIAN_POINT('Ctrl Pts',(-41.3551721676721,45.6807380719283,-9.02284347211491));
#43704=CARTESIAN_POINT('Ctrl Pts',(-41.2953272780234,45.8795837361382,-9.00476516996006));
#43705=CARTESIAN_POINT('Ctrl Pts',(-41.2103443351816,46.0195611794421,-9.13375196105432));
#43706=CARTESIAN_POINT('Ctrl Pts',(-41.3494454368654,45.6768975505525,-9.02107227041025));
#43707=CARTESIAN_POINT('Ctrl Pts',(-41.287409656368,45.8764014737269,-9.00151523627819));
#43708=CARTESIAN_POINT('Ctrl Pts',(-41.1988908745363,46.0161672311216,-9.13062146148794));
#43709=CARTESIAN_POINT('Ctrl Pts',(-41.3381720289335,45.6688915109853,-9.01736513631701));
#43710=CARTESIAN_POINT('Ctrl Pts',(-41.2718899027242,45.8697790039318,-8.99472450291166));
#43711=CARTESIAN_POINT('Ctrl Pts',(-41.1763440570616,46.0090921256199,-9.12406932266754));
#43712=CARTESIAN_POINT('Ctrl Pts',(-41.3326168231151,45.6647216906387,-9.01542726254812));
#43713=CARTESIAN_POINT('Ctrl Pts',(-41.2642748270683,45.8663339932396,-8.99117880533118));
#43714=CARTESIAN_POINT('Ctrl Pts',(-41.1652336469978,46.0054071688866,-9.12064423860081));
#43715=CARTESIAN_POINT('Ctrl Pts',(-41.3161815155429,45.6517477750581,-9.00937179381302));
#43716=CARTESIAN_POINT('Ctrl Pts',(-41.241826326959,45.8556226394696,-8.98010650018481));
#43717=CARTESIAN_POINT('Ctrl Pts',(-41.1323630295511,45.9939418469458,-9.10994155647637));
#43718=CARTESIAN_POINT('Ctrl Pts',(-41.3055311846566,45.6424803476347,-9.00501290349459));
#43719=CARTESIAN_POINT('Ctrl Pts',(-41.2274362460732,45.8479980985234,-8.97216285930692));
#43720=CARTESIAN_POINT('Ctrl Pts',(-41.1110623706261,45.985752028998,-9.10223746326134));
#43721=CARTESIAN_POINT('Ctrl Pts',(-41.2744096325773,45.6130614999026,-8.99103607019868));
#43722=CARTESIAN_POINT('Ctrl Pts',(-41.1857604875355,45.8238434014517,-8.9467425861811));
#43723=CARTESIAN_POINT('Ctrl Pts',(-41.0488192625286,45.9597539749973,-9.07753423341684));
#43724=CARTESIAN_POINT('Ctrl Pts',(-41.2547598251768,45.5913023257157,-8.98052231633313));
#43725=CARTESIAN_POINT('Ctrl Pts',(-41.1601629016934,45.8061099177734,-8.92775042784227));
#43726=CARTESIAN_POINT('Ctrl Pts',(-41.0095243303217,45.9405275308553,-9.05895435738375));
#43727=CARTESIAN_POINT('Ctrl Pts',(-41.2360638672433,45.567851127476,-8.96890239236004));
#43728=CARTESIAN_POINT('Ctrl Pts',(-41.1367508806195,45.7873702696317,-8.90717732011608));
#43729=CARTESIAN_POINT('Ctrl Pts',(-40.9721277344869,45.9198006242979,-9.03841423774551));
#43730=CARTESIAN_POINT('Origin',(-39.,48.5946168001447,-6.3392739254555));
#43731=CARTESIAN_POINT('',(-46.,52.2061427793358,-5.15737710185882));
#43732=CARTESIAN_POINT('Origin',(-46.,48.5946168001447,-6.3392739254555));
#43733=CARTESIAN_POINT('Ctrl Pts',(-46.,52.2061427793358,-5.15737710185883));
#43734=CARTESIAN_POINT('Ctrl Pts',(-46.,52.1813102167619,-5.08149615939848));
#43735=CARTESIAN_POINT('Ctrl Pts',(-45.9868485706877,52.1541549603842,-5.00673960430385));
#43736=CARTESIAN_POINT('Ctrl Pts',(-45.9274064730372,52.0781955342347,-4.81574086290611));
#43737=CARTESIAN_POINT('Ctrl Pts',(-45.8652318634837,52.0272394525228,-4.70527038001436));
#43738=CARTESIAN_POINT('Ctrl Pts',(-45.7071137304848,51.9128490522269,-4.48235789714551));
#43739=CARTESIAN_POINT('Ctrl Pts',(-45.6026237298735,51.8461984168199,-4.36873234959023));
#43740=CARTESIAN_POINT('Ctrl Pts',(-45.5017843995202,51.7768809810558,-4.26245040303759));
#43741=CARTESIAN_POINT('Ctrl Pts',(-45.5008921986149,51.7762672711454,-4.26151033429702));
#43742=CARTESIAN_POINT('Ctrl Pts',(-45.5,51.7756531463268,-4.26057054010477));
#43743=CARTESIAN_POINT('Origin',(-45.,48.5946168001447,-6.3392739254555));
#43744=CARTESIAN_POINT('Origin',(-45.5,52.6127679742695,-3.71354333343353));
#43745=CARTESIAN_POINT('Origin',(-46.,52.6127679742695,-3.71354333343353));
#43746=CARTESIAN_POINT('Origin',(-46.,52.6127679742695,-3.71354333343353));
#43747=CARTESIAN_POINT('Origin',(-45.,20.1123922190465,-8.20726109677752));
#43748=CARTESIAN_POINT('Origin',(-45.,19.0050007760892,0.400000000655));
#43749=CARTESIAN_POINT('Origin',(-45.,20.1123922190465,-8.20726109677752));
#43750=CARTESIAN_POINT('',(-45.,47.8027400910494,-6.80733765974042));
#43751=CARTESIAN_POINT('Origin',(-46.,34.999999994595,6.54998265276524E-10));
#43752=CARTESIAN_POINT('',(-46.,39.9275186688271,-2.44326824394971));
#43753=CARTESIAN_POINT('',(-46.,34.9369175583481,-0.136474846523149));
#43754=CARTESIAN_POINT('',(-46.,29.500909160648,-0.099999999345));
#43755=CARTESIAN_POINT('Origin',(-46.,34.999999994595,6.55E-10));
#43756=CARTESIAN_POINT('',(-46.,34.999999994595,-0.099999999345));
#43757=CARTESIAN_POINT('',(-46.,24.0004545494414,0.100000000654999));
#43758=CARTESIAN_POINT('',(-46.,29.0008333858067,0.100000000655));
#43759=CARTESIAN_POINT('',(-46.,34.999999994595,0.100000000655));
#43760=CARTESIAN_POINT('',(-46.,29.4923003031304,2.38017732779692));
#43761=CARTESIAN_POINT('Origin',(-46.,34.999999994595,6.55E-10));
#43762=CARTESIAN_POINT('',(-46.,24.952916660542,4.47840557391373));
#43763=CARTESIAN_POINT('',(-46.,34.9369175583481,-0.13647484652315));
#43764=CARTESIAN_POINT('Origin',(-46.,34.999999994595,6.55E-10));
#43765=CARTESIAN_POINT('Origin',(-46.,34.999999994595,6.55E-10));
#43766=CARTESIAN_POINT('Origin',(-29.,48.5946168001447,-3.5392739254555));
#43767=CARTESIAN_POINT('Origin',(-39.,56.5946168001448,-3.5392739254555));
#43768=CARTESIAN_POINT('Origin',(-33.5,53.0946168001448,-3.5392739254555));
#43769=CARTESIAN_POINT('',(-39.,48.5946168001447,-3.5392739254555));
#43770=CARTESIAN_POINT('Ctrl Pts',(-41.,51.6274934940962,-3.5392739254555));
#43771=CARTESIAN_POINT('Ctrl Pts',(-40.8774289857881,51.6274934940962,-3.5392739254555));
#43772=CARTESIAN_POINT('Ctrl Pts',(-40.7332628863176,51.6566516291422,-3.5392739254555));
#43773=CARTESIAN_POINT('Ctrl Pts',(-40.505929311989,51.7520470879015,-3.5392739254555));
#43774=CARTESIAN_POINT('Ctrl Pts',(-40.3828782109269,51.8356412158619,-3.5392739254555));
#43775=CARTESIAN_POINT('Ctrl Pts',(-40.2076014610043,52.0132462040385,-3.5392739254555));
#43776=CARTESIAN_POINT('Ctrl Pts',(-40.1248075750373,52.1391374121605,-3.5392739254555));
#43777=CARTESIAN_POINT('Ctrl Pts',(-40.0292644975066,52.3726433492684,-3.5392739254555));
#43778=CARTESIAN_POINT('Ctrl Pts',(-40.,52.5218803109357,-3.5392739254555));
#43779=CARTESIAN_POINT('Ctrl Pts',(-40.,52.6486129734088,-3.5392739254555));
#43780=CARTESIAN_POINT('Origin',(-42.,34.999999994595,6.55E-10));
#43781=CARTESIAN_POINT('Origin',(-42.,34.999999994595,6.55E-10));
#43782=CARTESIAN_POINT('Origin',(-42.5,34.999999994595,6.55E-10));
#43783=CARTESIAN_POINT('Origin',(-42.,34.999999994595,6.55E-10));
#43784=CARTESIAN_POINT('',(-42.5,24.5171568688013,0.600000000655));
#43785=CARTESIAN_POINT('Origin',(-42.5,34.999999994595,6.55E-10));
#43786=CARTESIAN_POINT('',(-45.5,24.5171568688013,0.600000000655));
#43787=CARTESIAN_POINT('',(-46.,24.5171568688013,0.600000000655));
#43788=CARTESIAN_POINT('Origin',(-45.5,34.999999994595,6.55E-10));
#43789=CARTESIAN_POINT('Origin',(-42.,34.999999994595,6.55E-10));
#43790=CARTESIAN_POINT('',(-42.,47.8027400910494,-6.80733765974042));
#43791=CARTESIAN_POINT('',(-42.,20.5417843370527,-1.099999999345));
#43792=CARTESIAN_POINT('Origin',(-42.,34.999999994595,6.55E-10));
#43793=CARTESIAN_POINT('',(-42.,28.5937530433762,-1.099999999345));
#43794=CARTESIAN_POINT('',(-42.,29.0300753719553,-1.099999999345));
#43795=CARTESIAN_POINT('Origin',(-42.,34.999999994595,6.55E-10));
#43796=CARTESIAN_POINT('Origin',(-42.,34.999999994595,6.55E-10));
#43797=CARTESIAN_POINT('',(-42.,38.1717829354129,9.48365926152771));
#43798=CARTESIAN_POINT('',(-42.,36.6893998635448,6.27661756768842));
#43799=CARTESIAN_POINT('',(-42.,36.5063304560983,5.88055852351209));
#43800=CARTESIAN_POINT('',(-42.,29.6176568283776,3.64422585000525));
#43801=CARTESIAN_POINT('Origin',(-42.,34.999999994595,6.55E-10));
#43802=CARTESIAN_POINT('',(-42.,26.4133371006572,5.12535075410315));
#43803=CARTESIAN_POINT('',(-42.,25.9224009791377,5.35227496195084));
#43804=CARTESIAN_POINT('Origin',(-42.,34.999999994595,6.55E-10));
#43805=CARTESIAN_POINT('Origin',(-42.,34.999999994595,6.55E-10));
#43806=CARTESIAN_POINT('',(-42.,25.0606841227656,1.100000000655));
#43807=CARTESIAN_POINT('',(-42.,25.0180162238208,1.100000000655));
#43808=CARTESIAN_POINT('',(-42.,25.5003909094963,3.12368808212367));
#43809=CARTESIAN_POINT('Origin',(-42.,34.999999994595,6.55E-10));
#43810=CARTESIAN_POINT('',(-42.,29.1031045477543,1.45841453098734));
#43811=CARTESIAN_POINT('Origin',(-46.,24.5171568688013,0.600000000655));
#43812=CARTESIAN_POINT('',(-42.5,29.0300753719553,0.600000000655));
#43813=CARTESIAN_POINT('',(-45.5,29.0300753719553,0.600000000655));
#43814=CARTESIAN_POINT('',(-42.,29.0300753719553,0.600000000655));
#43815=CARTESIAN_POINT('',(-45.5,24.5171568688013,0.600000000655));
#43816=CARTESIAN_POINT('Origin',(-42.,34.999999994595,6.55E-10));
#43817=CARTESIAN_POINT('Origin',(-42.5,34.999999994595,6.55E-10));
#43818=CARTESIAN_POINT('Origin',(-45.5,34.999999994595,6.55E-10));
#43819=CARTESIAN_POINT('Origin',(-42.,34.999999994595,6.55E-10));
#43820=CARTESIAN_POINT('Origin',(-42.,34.999999994595,6.55E-10));
#43821=CARTESIAN_POINT('Origin',(-42.5,34.999999994595,6.55E-10));
#43822=CARTESIAN_POINT('Origin',(-45.5,34.999999994595,6.55E-10));
#43823=CARTESIAN_POINT('Origin',(-42.,34.999999994595,6.55E-10));
#43824=CARTESIAN_POINT('Ctrl Pts',(-45.5,29.3128914363174,1.91227514988591));
#43825=CARTESIAN_POINT('Ctrl Pts',(-45.5628391134956,29.3128914363174,1.91227514988591));
#43826=CARTESIAN_POINT('Ctrl Pts',(-45.6298331441263,29.3168834840241,1.92427779549175));
#43827=CARTESIAN_POINT('Ctrl Pts',(-45.7530108833858,29.3335483580741,1.97281123155531));
#43828=CARTESIAN_POINT('Ctrl Pts',(-45.8091981254106,29.3462726308219,2.00931537180972));
#43829=CARTESIAN_POINT('Ctrl Pts',(-45.8979247274123,29.3767120398422,2.09299196879008));
#43830=CARTESIAN_POINT('Ctrl Pts',(-45.9363923973194,29.3964723731256,2.14575933493431));
#43831=CARTESIAN_POINT('Ctrl Pts',(-45.9874312621461,29.4417718124439,2.26050976623123));
#43832=CARTESIAN_POINT('Ctrl Pts',(-46.,29.4673632318665,2.32247326594399));
#43833=CARTESIAN_POINT('Ctrl Pts',(-46.,29.4923003031304,2.38017732779691));
#43834=CARTESIAN_POINT('Ctrl Pts',(-46.,29.0008333858068,0.100000000654999));
#43835=CARTESIAN_POINT('Ctrl Pts',(-46.,29.0018807488039,0.162833051853196));
#43836=CARTESIAN_POINT('Ctrl Pts',(-45.987434136778,29.0040858280371,0.229815422305264));
#43837=CARTESIAN_POINT('Ctrl Pts',(-45.9363958048209,29.0100749953873,0.352987712488953));
#43838=CARTESIAN_POINT('Ctrl Pts',(-45.897925533031,29.0138032964881,0.409181248810524));
#43839=CARTESIAN_POINT('Ctrl Pts',(-45.8091901150632,29.0205302518391,0.49791666677831));
#43840=CARTESIAN_POINT('Ctrl Pts',(-45.7529965530102,29.0239694137344,0.536391275967779));
#43841=CARTESIAN_POINT('Ctrl Pts',(-45.6298176902908,29.0287707804367,0.587434063339562));
#43842=CARTESIAN_POINT('Ctrl Pts',(-45.5628292221247,29.0300753719553,0.600000000654999));
#43843=CARTESIAN_POINT('Ctrl Pts',(-45.5,29.0300753719553,0.600000000654999));
#43844=CARTESIAN_POINT('Origin',(-45.5,34.999999994595,6.55E-10));
#43845=CARTESIAN_POINT('Origin',(-45.5,34.999999994595,6.55E-10));
#43846=CARTESIAN_POINT('Ctrl Pts',(-46.,24.952916660542,4.47840557391373));
#43847=CARTESIAN_POINT('Ctrl Pts',(-46.,24.9534438587617,4.47700178764069));
#43848=CARTESIAN_POINT('Ctrl Pts',(-45.9999966732694,24.9539711604922,4.47559803619075));
#43849=CARTESIAN_POINT('Ctrl Pts',(-45.9994155814552,25.000042193889,4.35297758352556));
#43850=CARTESIAN_POINT('Ctrl Pts',(-45.9740798347619,25.0455855649062,4.23423066579828));
#43851=CARTESIAN_POINT('Ctrl Pts',(-45.8905117508397,25.1174860867329,4.04969045435885));
#43852=CARTESIAN_POINT('Ctrl Pts',(-45.8415534230064,25.1451044879621,3.97986335572903));
#43853=CARTESIAN_POINT('Ctrl Pts',(-45.7413191892353,25.1822011485462,3.8867107561863));
#43854=CARTESIAN_POINT('Ctrl Pts',(-45.6923971848574,25.195297523774,3.85407797624252));
#43855=CARTESIAN_POINT('Ctrl Pts',(-45.5936828209341,25.21066817034,3.81586538743094));
#43856=CARTESIAN_POINT('Ctrl Pts',(-45.5474486391928,25.2143573355172,3.80673058592582));
#43857=CARTESIAN_POINT('Ctrl Pts',(-45.5,25.2143573355172,3.80673058592582));
#43858=CARTESIAN_POINT('Ctrl Pts',(-46.,24.0004545494414,0.100000000655013));
#43859=CARTESIAN_POINT('Ctrl Pts',(-46.,24.0015172240447,0.101053058095808));
#43860=CARTESIAN_POINT('Ctrl Pts',(-45.9999966732101,24.0025799776156,0.102106041183611));
#43861=CARTESIAN_POINT('Ctrl Pts',(-45.9996481828921,24.0582582442755,0.157264429326908));
#43862=CARTESIAN_POINT('Ctrl Pts',(-45.9905229793199,24.113427651011,0.211504412924178));
#43863=CARTESIAN_POINT('Ctrl Pts',(-45.9552065634892,24.2178946933341,0.313459887982052));
#43864=CARTESIAN_POINT('Ctrl Pts',(-45.9295269357133,24.2681331179157,0.362125603591196));
#43865=CARTESIAN_POINT('Ctrl Pts',(-45.8607273465329,24.3600964972318,0.450654394481858));
#43866=CARTESIAN_POINT('Ctrl Pts',(-45.8173190858306,24.4027631032684,0.491431360067023));
#43867=CARTESIAN_POINT('Ctrl Pts',(-45.7252137953263,24.4630158614508,0.54876653070038));
#43868=CARTESIAN_POINT('Ctrl Pts',(-45.6810126507288,24.484178630487,0.568815347785938));
#43869=CARTESIAN_POINT('Ctrl Pts',(-45.5900334171141,24.5105597708073,0.593774499405668));
#43870=CARTESIAN_POINT('Ctrl Pts',(-45.5456486747149,24.5171385264558,0.599982678137806));
#43871=CARTESIAN_POINT('Ctrl Pts',(-45.5001267533779,24.5171568560425,0.599999988604697));
#43872=CARTESIAN_POINT('Ctrl Pts',(-45.5000633756126,24.5171568688013,0.600000000654999));
#43873=CARTESIAN_POINT('Ctrl Pts',(-45.5,24.5171568688013,0.600000000654999));
#43874=CARTESIAN_POINT('Origin',(-45.5,34.9369175583481,-0.136474846523149));
#43875=CARTESIAN_POINT('Origin',(-45.5,34.9369175583481,-0.136474846523149));
#43876=CARTESIAN_POINT('Ctrl Pts',(-45.5,40.1413699032525,-3.09294608072936));
#43877=CARTESIAN_POINT('Ctrl Pts',(-45.5491501916832,40.1413699032525,-3.09294608072936));
#43878=CARTESIAN_POINT('Ctrl Pts',(-45.5972692604454,40.138519820516,-3.08364786424418));
#43879=CARTESIAN_POINT('Ctrl Pts',(-45.6941793711978,40.1270402998169,-3.04649616739224));
#43880=CARTESIAN_POINT('Ctrl Pts',(-45.7405959310225,40.1179528663737,-3.01720069323527));
#43881=CARTESIAN_POINT('Ctrl Pts',(-45.8337415969986,40.0922525585882,-2.93547744772848));
#43882=CARTESIAN_POINT('Ctrl Pts',(-45.8761467093307,40.0744137826655,-2.87945196974603));
#43883=CARTESIAN_POINT('Ctrl Pts',(-45.9391011359062,40.0366703300967,-2.76344022534597));
#43884=CARTESIAN_POINT('Ctrl Pts',(-45.961318424291,40.0169300538135,-2.70376918947611));
#43885=CARTESIAN_POINT('Ctrl Pts',(-45.9919234108107,39.9747588404363,-2.57887452839208));
#43886=CARTESIAN_POINT('Ctrl Pts',(-45.9996764174093,39.9520381992281,-2.51291999016442));
#43887=CARTESIAN_POINT('Ctrl Pts',(-45.9999966934192,39.9284920364042,-2.44603148477463));
#43888=CARTESIAN_POINT('Ctrl Pts',(-46.,39.9280054482978,-2.44464982890693));
#43889=CARTESIAN_POINT('Ctrl Pts',(-46.,39.9275186688271,-2.44326824394971));
#43890=CARTESIAN_POINT('Origin',(-45.5,34.999999994595,0.100000000655));
#43891=CARTESIAN_POINT('Origin',(-45.5,34.999999994595,6.55E-10));
#43892=CARTESIAN_POINT('Ctrl Pts',(-45.5,29.0300753719553,-0.599999999345));
#43893=CARTESIAN_POINT('Ctrl Pts',(-45.548970157778,29.0300753719553,-0.599999999345));
#43894=CARTESIAN_POINT('Ctrl Pts',(-45.5969081567834,29.0365711967785,-0.592808580903382));
#43895=CARTESIAN_POINT('Ctrl Pts',(-45.6935221969332,29.0626157928012,-0.564105664860167));
#43896=CARTESIAN_POINT('Ctrl Pts',(-45.7398209612911,29.0831997568478,-0.54147109065902));
#43897=CARTESIAN_POINT('Ctrl Pts',(-45.8328892935188,29.1409993072008,-0.478410110413383));
#43898=CARTESIAN_POINT('Ctrl Pts',(-45.8753161788561,29.1808820841999,-0.435208680228837));
#43899=CARTESIAN_POINT('Ctrl Pts',(-45.9385897729846,29.2644717707674,-0.345802317210053));
#43900=CARTESIAN_POINT('Ctrl Pts',(-45.9609910872763,29.3079608495334,-0.299750899422561));
#43901=CARTESIAN_POINT('Ctrl Pts',(-45.9918589780637,29.3998033012657,-0.203702083584708));
#43902=CARTESIAN_POINT('Ctrl Pts',(-45.9996751413528,29.448752394715,-0.153142830446623));
#43903=CARTESIAN_POINT('Ctrl Pts',(-45.9999966939211,29.498847589825,-0.102099695500558));
#43904=CARTESIAN_POINT('Ctrl Pts',(-46.,29.4998783026423,-0.101049773754294));
#43905=CARTESIAN_POINT('Ctrl Pts',(-46.,29.500909160648,-0.0999999993449992));
#43906=CARTESIAN_POINT('Origin',(-45.5,34.999999994595,-0.099999999345));
#43907=CARTESIAN_POINT('Ctrl Pts',(-45.9555887800306,18.2967958718846,-0.306006949495302));
#43908=CARTESIAN_POINT('Ctrl Pts',(-45.9286742504228,18.3561332001619,-0.365529007853841));
#43909=CARTESIAN_POINT('Ctrl Pts',(-45.8916577250397,18.4215697732152,-0.415449055491825));
#43910=CARTESIAN_POINT('Ctrl Pts',(-45.7584535062404,18.6397957575259,-0.548653274291119));
#43911=CARTESIAN_POINT('Ctrl Pts',(-45.6188300321941,18.8369497329432,-0.599999999344998));
#43912=CARTESIAN_POINT('Ctrl Pts',(-45.5,19.0050007760892,-0.599999999344998));
#43913=CARTESIAN_POINT('Origin',(-39.,20.2255401693197,4.45249206217833));
#43914=CARTESIAN_POINT('',(-39.,20.2255401693197,4.45249206217833));
#43915=CARTESIAN_POINT('Origin',(-46.,19.0050007760892,0.400000000655));
#43916=CARTESIAN_POINT('Origin',(-30.,39.9592920728172,13.6255430020507));
#43917=CARTESIAN_POINT('Origin',(-39.,56.5946168001448,6.5496670161002E-10));
#43918=CARTESIAN_POINT('',(-39.7071067811866,57.3017235813313,0.915815935106727));
#43919=CARTESIAN_POINT('Ctrl Pts',(-40.,56.5946168001448,0.460726074544506));
#43920=CARTESIAN_POINT('Ctrl Pts',(-40.,56.6851510498546,0.524743456443905));
#43921=CARTESIAN_POINT('Ctrl Pts',(-39.9870743510596,56.783707730714,0.594529537273628));
#43922=CARTESIAN_POINT('Ctrl Pts',(-39.9298163989785,56.9760781041861,0.726060874194729));
#43923=CARTESIAN_POINT('Ctrl Pts',(-39.8854254499147,57.0699455247195,0.787701988575014));
#43924=CARTESIAN_POINT('Ctrl Pts',(-39.7965927093604,57.2020671761929,0.865686530039721));
#43925=CARTESIAN_POINT('Ctrl Pts',(-39.7551464473864,57.2536839151314,0.893953570114362));
#43926=CARTESIAN_POINT('Ctrl Pts',(-39.7071067811866,57.3017235813313,0.915815935106716));
#43927=CARTESIAN_POINT('Ctrl Pts',(-39.7071067811866,57.3017235813313,0.915815935106747));
#43928=CARTESIAN_POINT('Ctrl Pts',(-39.6590671149867,57.3497632475312,0.893953570114389));
#43929=CARTESIAN_POINT('Ctrl Pts',(-39.6074503760481,57.3912095095051,0.865686530039736));
#43930=CARTESIAN_POINT('Ctrl Pts',(-39.4753287245747,57.4800422500596,0.787701988575014));
#43931=CARTESIAN_POINT('Ctrl Pts',(-39.3814613040413,57.5244331991233,0.726060874194723));
#43932=CARTESIAN_POINT('Ctrl Pts',(-39.1890909305692,57.5816911512044,0.594529537273623));
#43933=CARTESIAN_POINT('Ctrl Pts',(-39.0905342497097,57.5946168001448,0.524743456443903));
#43934=CARTESIAN_POINT('Ctrl Pts',(-39.,57.5946168001448,0.460726074544505));
#43935=CARTESIAN_POINT('Origin',(-29.,49.0946168001447,0.460726074544506));
#43936=CARTESIAN_POINT('',(-29.,49.0946168001447,0.960726074544506));
#43937=CARTESIAN_POINT('Origin',(-36.7071067811866,49.0946168001449,0.460726074544334));
#43938=CARTESIAN_POINT('Origin',(-41.,34.999999994595,6.54998265276524E-10));
#43939=CARTESIAN_POINT('Ctrl Pts',(-40.9999916854225,51.9933714024979,0.474687470722451));
#43940=CARTESIAN_POINT('Ctrl Pts',(-40.9669669960565,51.9933716766225,0.474687466548977));
#43941=CARTESIAN_POINT('Ctrl Pts',(-40.9012775948277,51.9966387486667,0.4746377262469));
#43942=CARTESIAN_POINT('Ctrl Pts',(-40.8363006666026,52.0063215827071,0.474490566145437));
#43943=CARTESIAN_POINT('Ctrl Pts',(-40.7878360936142,52.01601685831,0.474343539939905));
#43944=CARTESIAN_POINT('Ctrl Pts',(-40.7717013944448,52.0196627095898,0.474288294394399));
#43945=CARTESIAN_POINT('Ctrl Pts',(-40.7398056090422,52.0277029666335,0.474166606459729));
#43946=CARTESIAN_POINT('Ctrl Pts',(-40.6924300624422,52.040902120181,0.473967040272293));
#43947=CARTESIAN_POINT('Ctrl Pts',(-40.6157642654392,52.0684797155497,0.473551566584779));
#43948=CARTESIAN_POINT('Ctrl Pts',(-40.5568449560762,52.0964124422323,0.473133577527132));
#43949=CARTESIAN_POINT('Ctrl Pts',(-40.5135744864942,52.1195975832219,0.472788208703002));
#43950=CARTESIAN_POINT('Ctrl Pts',(-40.4993044370294,52.1276992237301,0.472667764625631));
#43951=CARTESIAN_POINT('Ctrl Pts',(-40.4781338636937,52.1404221344366,0.472479067172326));
#43952=CARTESIAN_POINT('Ctrl Pts',(-40.4711065130498,52.1447644052945,0.472414737515416));
#43953=CARTESIAN_POINT('Ctrl Pts',(-40.4571840957994,52.1536074404532,0.472283888769367));
#43954=CARTESIAN_POINT('Ctrl Pts',(-40.4227223611727,52.1761016382909,0.471951435217613));
#43955=CARTESIAN_POINT('Ctrl Pts',(-40.363742898356,52.220017783896,0.471306160137212));
#43956=CARTESIAN_POINT('Ctrl Pts',(-40.2914457842733,52.2856940685341,0.470351766833669));
#43957=CARTESIAN_POINT('Ctrl Pts',(-40.247486690588,52.3342381117076,0.469654917353387));
#43958=CARTESIAN_POINT('Ctrl Pts',(-40.2213795506908,52.3661134507234,0.469200546860636));
#43959=CARTESIAN_POINT('Ctrl Pts',(-40.216222153751,52.3725716342351,0.469108641273594));
#43960=CARTESIAN_POINT('Ctrl Pts',(-40.2060999842062,52.3855731513054,0.468923937574523));
#43961=CARTESIAN_POINT('Ctrl Pts',(-40.1911870321444,52.4052251480644,0.468645228815098));
#43962=CARTESIAN_POINT('Ctrl Pts',(-40.1582619483118,52.4521166070354,0.467983631257275));
#43963=CARTESIAN_POINT('Ctrl Pts',(-40.1164784540024,52.5220137105018,0.467007786904805));
#43964=CARTESIAN_POINT('Ctrl Pts',(-40.0885974238781,52.5810032526374,0.466196427926919));
#43965=CARTESIAN_POINT('Ctrl Pts',(-40.069805896849,52.6264192897992,0.46557672633137));
#43966=CARTESIAN_POINT('Ctrl Pts',(-40.0638958909063,52.6417539639008,0.465368290852179));
#43967=CARTESIAN_POINT('Ctrl Pts',(-40.0555726258997,52.6650560555401,0.465052833465107));
#43968=CARTESIAN_POINT('Ctrl Pts',(-40.0528914574447,52.6728662080822,0.464947312131413));
#43969=CARTESIAN_POINT('Ctrl Pts',(-40.0477386832659,52.688501047461,0.464736497152779));
#43970=CARTESIAN_POINT('Ctrl Pts',(-40.0353635450435,52.7276744199,0.464209352250129));
#43971=CARTESIAN_POINT('Ctrl Pts',(-40.0175847433647,52.7989519400502,0.463259743685644));
#43972=CARTESIAN_POINT('Ctrl Pts',(-40.0032590220346,52.8955853337854,0.461993031367599));
#43973=CARTESIAN_POINT('Ctrl Pts',(-40.,52.961078630892,0.461148437744956));
#43974=CARTESIAN_POINT('Ctrl Pts',(-40.,52.9941026808875,0.460726074544506));
#43975=CARTESIAN_POINT('Origin',(-29.,48.5946168001447,0.960726074544506));
#43976=CARTESIAN_POINT('',(-39.5,57.0946168001448,0.960726074544506));
#43977=CARTESIAN_POINT('',(-29.,57.0946168001448,0.960726074544506));
#43978=CARTESIAN_POINT('',(-39.5,52.9941026808875,0.960726074544506));
#43979=CARTESIAN_POINT('',(-39.5,52.9743429703744,0.960726074544506));
#43980=CARTESIAN_POINT('Origin',(-41.0008349053211,52.9940758729588,0.960726074536255));
#43981=CARTESIAN_POINT('Origin',(-39.5,34.999999994595,0.460726074544506));
#43982=CARTESIAN_POINT('Origin',(-39.4999999999966,57.0946168001405,0.460726074522097));
#43983=CARTESIAN_POINT('Origin',(-39.5,52.9941026808875,0.460726074544506));
#43984=CARTESIAN_POINT('Origin',(-29.,57.0946168001448,0.460726074544506));
#43985=CARTESIAN_POINT('Ctrl Pts',(-40.0001655039079,53.0123407644378,0.460493170805832));
#43986=CARTESIAN_POINT('Ctrl Pts',(-40.0003984920697,53.012336506285,0.960745122447957));
#43987=CARTESIAN_POINT('Ctrl Pts',(-39.5002292175527,53.0214512149348,0.960726074182035));
#43988=CARTESIAN_POINT('Ctrl Pts',(-39.9994498624972,52.9728908588742,0.460996190252693));
#43989=CARTESIAN_POINT('Ctrl Pts',(-39.9991801743049,52.9729248253368,0.960745093722174));
#43990=CARTESIAN_POINT('Ctrl Pts',(-39.499155759087,52.9622948946583,0.9607260741824));
#43991=CARTESIAN_POINT('Ctrl Pts',(-40.0010599694177,52.9338359806619,0.461499117712378));
#43992=CARTESIAN_POINT('Ctrl Pts',(-40.0002848056282,52.9338282680843,0.960745065037616));
#43993=CARTESIAN_POINT('Ctrl Pts',(-39.5015709557979,52.903731217001,0.960726074182764));
#43994=CARTESIAN_POINT('Ctrl Pts',(-40.0081477928623,52.8624555520283,0.462427261950409));
#43995=CARTESIAN_POINT('Ctrl Pts',(-40.0064631934232,52.8622602496085,0.960745012189611));
#43996=CARTESIAN_POINT('Ctrl Pts',(-39.512202841528,52.7966951634192,0.960726074183437));
#43997=CARTESIAN_POINT('Ctrl Pts',(-40.0129905514434,52.8300215069154,0.462852495681728));
#43998=CARTESIAN_POINT('Ctrl Pts',(-40.0108949524489,52.8297015577819,0.960744988014785));
#43999=CARTESIAN_POINT('Ctrl Pts',(-39.5194670799186,52.7480600167976,0.960726074183745));
#44000=CARTESIAN_POINT('Ctrl Pts',(-40.0258472542811,52.7656933673554,0.463702766417071));
#44001=CARTESIAN_POINT('Ctrl Pts',(-40.0229589514936,52.7650452541844,0.960744939747848));
#44002=CARTESIAN_POINT('Ctrl Pts',(-39.5387523946349,52.6515997894431,0.960726074184361));
#44003=CARTESIAN_POINT('Ctrl Pts',(-40.0338610657608,52.7337992504474,0.464127804316484));
#44004=CARTESIAN_POINT('Ctrl Pts',(-40.0305883230144,52.7329471688104,0.960744915655539));
#44005=CARTESIAN_POINT('Ctrl Pts',(-39.5507732701283,52.6037746745126,0.960726074184669));
#44006=CARTESIAN_POINT('Ctrl Pts',(-40.0459065884668,52.6942769582217,0.464658757667562));
#44007=CARTESIAN_POINT('Ctrl Pts',(-40.0421830649057,52.6931098486124,0.960744885594489));
#44008=CARTESIAN_POINT('Ctrl Pts',(-39.5688417936154,52.5445113921488,0.960726074185053));
#44009=CARTESIAN_POINT('Ctrl Pts',(-40.0484173432833,52.686389808028,0.464764930564257));
#44010=CARTESIAN_POINT('Ctrl Pts',(-40.0446041297497,52.6851598207343,0.9607448795874));
#44011=CARTESIAN_POINT('Ctrl Pts',(-39.5726079746068,52.5326847014799,0.96072607418513));
#44012=CARTESIAN_POINT('Ctrl Pts',(-40.0536442942955,52.6706504884901,0.464977232783128));
#44013=CARTESIAN_POINT('Ctrl Pts',(-40.0496543933496,52.6692900276159,0.960744867580106));
#44014=CARTESIAN_POINT('Ctrl Pts',(-39.5804485047973,52.5090837996536,0.960726074185284));
#44015=CARTESIAN_POINT('Ctrl Pts',(-40.0563645657016,52.6627872826563,0.465083511790395));
#44016=CARTESIAN_POINT('Ctrl Pts',(-40.0522875048945,52.6613591123839,0.960744861571438));
#44017=CARTESIAN_POINT('Ctrl Pts',(-39.5845289653705,52.4972930389892,0.960726074185361));
#44018=CARTESIAN_POINT('Ctrl Pts',(-40.0648010481868,52.6393500297714,0.465400924687527));
#44019=CARTESIAN_POINT('Ctrl Pts',(-40.0604670716587,52.6377151220421,0.960744843634412));
#44020=CARTESIAN_POINT('Ctrl Pts',(-39.5971838533673,52.4621492626542,0.960726074185592));
#44021=CARTESIAN_POINT('Ctrl Pts',(-40.0707911880509,52.623927967324,0.465610636191831));
#44022=CARTESIAN_POINT('Ctrl Pts',(-40.0662935062176,52.6221453256381,0.960744831791026));
#44023=CARTESIAN_POINT('Ctrl Pts',(-39.6061691817211,52.4390241844292,0.960726074185743));
#44024=CARTESIAN_POINT('Ctrl Pts',(-40.0898370304849,52.5782578888926,0.466234080194723));
#44025=CARTESIAN_POINT('Ctrl Pts',(-40.084867712451,52.5760195290014,0.960744796614806));
#44026=CARTESIAN_POINT('Ctrl Pts',(-39.6347383153858,52.3705429448364,0.960726074186195));
#44027=CARTESIAN_POINT('Ctrl Pts',(-40.1039655757069,52.5486045524486,0.466642140861632));
#44028=CARTESIAN_POINT('Ctrl Pts',(-40.0987139813306,52.5460250690031,0.960744773619268));
#44029=CARTESIAN_POINT('Ctrl Pts',(-39.6559314088288,52.3260786404838,0.96072607418649));
#44030=CARTESIAN_POINT('Ctrl Pts',(-40.1350337723299,52.4908561093173,0.467442665085129));
#44031=CARTESIAN_POINT('Ctrl Pts',(-40.1292885679029,52.487546836494,0.960744728569577));
#44032=CARTESIAN_POINT('Ctrl Pts',(-39.702534304357,52.2394869022988,0.960726074187071));
#44033=CARTESIAN_POINT('Ctrl Pts',(-40.1519734728763,52.4627610299867,0.467835129764516));
#44034=CARTESIAN_POINT('Ctrl Pts',(-40.1460151229703,52.4590609364356,0.960744706513894));
#44035=CARTESIAN_POINT('Ctrl Pts',(-39.727944181063,52.19735950989,0.960726074187355));
#44036=CARTESIAN_POINT('Ctrl Pts',(-40.1795147094014,52.421800055698,0.468411323187832));
#44037=CARTESIAN_POINT('Ctrl Pts',(-40.1733008051782,52.4174778892912,0.960744674169833));
#44038=CARTESIAN_POINT('Ctrl Pts',(-39.7692565659718,52.1359404926989,0.960726074187773));
#44039=CARTESIAN_POINT('Ctrl Pts',(-40.1890510386164,52.4083436912061,0.468601298890646));
#44040=CARTESIAN_POINT('Ctrl Pts',(-40.1827597525983,52.4038117349707,0.960744663514773));
#44041=CARTESIAN_POINT('Ctrl Pts',(-39.7835612418075,52.1157633598134,0.96072607418791));
#44042=CARTESIAN_POINT('Ctrl Pts',(-40.203898320647,52.3884600286176,0.468882980831395));
#44043=CARTESIAN_POINT('Ctrl Pts',(-40.1975076720815,52.3836053509173,0.96074464772499));
#44044=CARTESIAN_POINT('Ctrl Pts',(-39.8058324502274,52.0859488816049,0.960726074188115));
#44045=CARTESIAN_POINT('Ctrl Pts',(-40.2089379225118,52.3818823125493,0.468976327560764));
#44046=CARTESIAN_POINT('Ctrl Pts',(-40.2025162200678,52.3769196053701,0.960744642494575));
#44047=CARTESIAN_POINT('Ctrl Pts',(-39.8133919488952,52.076085960794,0.960726074188182));
#44048=CARTESIAN_POINT('Ctrl Pts',(-40.2192001688965,52.3688283470369,0.469161897284951));
#44049=CARTESIAN_POINT('Ctrl Pts',(-40.2127215810503,52.3636476684092,0.960744632100017));
#44050=CARTESIAN_POINT('Ctrl Pts',(-39.8287855156091,52.0565122835928,0.960726074188316));
#44051=CARTESIAN_POINT('Ctrl Pts',(-40.2244232075698,52.3623522299886,0.469254119011349));
#44052=CARTESIAN_POINT('Ctrl Pts',(-40.2179187794572,52.3570615644569,0.960744626935923));
#44053=CARTESIAN_POINT('Ctrl Pts',(-39.8366201735086,52.0468017246971,0.960726074188384));
#44054=CARTESIAN_POINT('Ctrl Pts',(-40.2508489212739,52.3304076335106,0.469709778885052));
#44055=CARTESIAN_POINT('Ctrl Pts',(-40.2442221313025,52.3245746168839,0.960744601435455));
#44056=CARTESIAN_POINT('Ctrl Pts',(-39.8762592480715,51.9989027144972,0.960726074188714));
#44057=CARTESIAN_POINT('Ctrl Pts',(-40.273095635695,52.3060951210873,0.470059023733022));
#44058=CARTESIAN_POINT('Ctrl Pts',(-40.2664202498769,52.2998131605779,0.960744581909348));
#44059=CARTESIAN_POINT('Ctrl Pts',(-39.9096297458151,51.9624477101716,0.960726074188967));
#44060=CARTESIAN_POINT('Ctrl Pts',(-40.3197348873262,52.2598817711329,0.47072674893928));
#44061=CARTESIAN_POINT('Ctrl Pts',(-40.3130496584301,52.2527055307459,0.960744544620133));
#44062=CARTESIAN_POINT('Ctrl Pts',(-39.9795895104191,51.8931540832812,0.96072607418945));
#44063=CARTESIAN_POINT('Ctrl Pts',(-40.3441275914038,52.2379811214821,0.471045228543483));
#44064=CARTESIAN_POINT('Ctrl Pts',(-40.3374810791704,52.2303564867772,0.960744526854748));
#44065=CARTESIAN_POINT('Ctrl Pts',(-40.0161790302021,51.8603157450578,0.960726074189681));
#44066=CARTESIAN_POINT('Ctrl Pts',(-40.3950567662191,52.1965892330283,0.471650299906407));
#44067=CARTESIAN_POINT('Ctrl Pts',(-40.3885742287628,52.1880843837587,0.96074449313787));
#44068=CARTESIAN_POINT('Ctrl Pts',(-40.0925737593492,51.7982519901567,0.960726074190119));
#44069=CARTESIAN_POINT('Ctrl Pts',(-40.4215930942303,52.1770978340976,0.471936895541539));
#44070=CARTESIAN_POINT('Ctrl Pts',(-40.4152361106502,52.168158359676,0.960744477184023));
#44071=CARTESIAN_POINT('Ctrl Pts',(-40.1323787528732,51.7690263311577,0.960726074190327));
#44072=CARTESIAN_POINT('Ctrl Pts',(-40.4630511915683,52.1497192822008,0.472341311397696));
#44073=CARTESIAN_POINT('Ctrl Pts',(-40.4569521385459,52.1401467612328,0.960744454689427));
#44074=CARTESIAN_POINT('Ctrl Pts',(-40.1945666842034,51.7279746912277,0.96072607419062));
#44075=CARTESIAN_POINT('Ctrl Pts',(-40.4771781181886,52.1408868781905,0.472472109426542));
#44076=CARTESIAN_POINT('Ctrl Pts',(-40.4711742927655,52.1311074238323,0.960744447418406));
#44077=CARTESIAN_POINT('Ctrl Pts',(-40.2157573411748,51.7147313274549,0.960726074190715));
#44078=CARTESIAN_POINT('Ctrl Pts',(-40.5056906476565,52.1240325721919,0.47272224767737));
#44079=CARTESIAN_POINT('Ctrl Pts',(-40.4998960757661,52.113852479979,0.960744433519271));
#44080=CARTESIAN_POINT('Ctrl Pts',(-40.2585266732872,51.689459904419,0.960726074190896));
#44081=CARTESIAN_POINT('Ctrl Pts',(-40.5201047475496,52.1159897576834,0.472841895424202));
#44082=CARTESIAN_POINT('Ctrl Pts',(-40.514424530058,52.1056151429109,0.960744426873757));
#44083=CARTESIAN_POINT('Ctrl Pts',(-40.2801480959472,51.6774004912111,0.960726074190983));
#44084=CARTESIAN_POINT('Ctrl Pts',(-40.5638122296279,52.0929940680948,0.473184660310897));
#44085=CARTESIAN_POINT('Ctrl Pts',(-40.5584969221185,52.0820589039531,0.96074440784537));
#44086=CARTESIAN_POINT('Ctrl Pts',(-40.345710143499,51.6429207424569,0.960726074191231));
#44087=CARTESIAN_POINT('Ctrl Pts',(-40.5935696830967,52.0791712433114,0.473391632961349));
#44088=CARTESIAN_POINT('Ctrl Pts',(-40.588538086652,52.0678858991667,0.960744396362926));
#44089=CARTESIAN_POINT('Ctrl Pts',(-40.3903468851132,51.6221948521615,0.960726074191381));
#44090=CARTESIAN_POINT('Ctrl Pts',(-40.6543065460004,52.0545011905415,0.4737621108513));
#44091=CARTESIAN_POINT('Ctrl Pts',(-40.6499035064575,52.0425809534879,0.960744375822678));
#44092=CARTESIAN_POINT('Ctrl Pts',(-40.4814533235621,51.5852047365437,0.96072607419165));
#44093=CARTESIAN_POINT('Ctrl Pts',(-40.6852859475085,52.043653943586,0.47392561750322));
#44094=CARTESIAN_POINT('Ctrl Pts',(-40.6812299251525,52.0314467950658,0.960744366763052));
#44095=CARTESIAN_POINT('Ctrl Pts',(-40.5279230084688,51.5689404826149,0.960726074191768));
#44096=CARTESIAN_POINT('Ctrl Pts',(-40.7326861808497,52.0296505042667,0.474137149769106));
#44097=CARTESIAN_POINT('Ctrl Pts',(-40.7291925714429,52.0170682302869,0.960744355047342));
#44098=CARTESIAN_POINT('Ctrl Pts',(-40.5990242502966,51.5479438967512,0.960726074191921));
#44099=CARTESIAN_POINT('Ctrl Pts',(-40.7486417259643,52.0253612757894,0.474202030566825));
#44100=CARTESIAN_POINT('Ctrl Pts',(-40.7453413637245,52.0126633195588,0.960744351455017));
#44101=CARTESIAN_POINT('Ctrl Pts',(-40.6229578676032,51.5415126836689,0.960726074191969));
#44102=CARTESIAN_POINT('Ctrl Pts',(-40.772812741707,52.0195062621464,0.474290680866358));
#44103=CARTESIAN_POINT('Ctrl Pts',(-40.7698118586169,52.0066494175163,0.960744346547479));
#44104=CARTESIAN_POINT('Ctrl Pts',(-40.6592148458315,51.5327337612339,0.960726074192033));
#44105=CARTESIAN_POINT('Ctrl Pts',(-40.7809209123333,52.0176487217575,0.474318821429952));
#44106=CARTESIAN_POINT('Ctrl Pts',(-40.778021312729,52.0047413385575,0.960744344989861));
#44107=CARTESIAN_POINT('Ctrl Pts',(-40.6713772541575,51.5299485927647,0.960726074192054));
#44108=CARTESIAN_POINT('Ctrl Pts',(-40.7971478395831,52.0141437354624,0.474371943666935));
#44109=CARTESIAN_POINT('Ctrl Pts',(-40.7944527664113,52.0011407470928,0.960744342049743));
#44110=CARTESIAN_POINT('Ctrl Pts',(-40.6957179497932,51.5246932689571,0.960726074192092));
#44111=CARTESIAN_POINT('Ctrl Pts',(-40.8052667802835,52.0124958472928,0.474396931937503));
#44112=CARTESIAN_POINT('Ctrl Pts',(-40.8026749958654,51.9994477605747,0.960744340666859));
#44113=CARTESIAN_POINT('Ctrl Pts',(-40.7078965135666,51.5222224521958,0.96072607419211));
#44114=CARTESIAN_POINT('Ctrl Pts',(-40.8458885680889,52.0047736588639,0.474514075775359));
#44115=CARTESIAN_POINT('Ctrl Pts',(-40.843814734944,51.9915143162406,0.960744334184926));
#44116=CARTESIAN_POINT('Ctrl Pts',(-40.768829958314,51.5106439255071,0.960726074192195));
#44117=CARTESIAN_POINT('Ctrl Pts',(-40.878472462022,52.0002472210685,0.474582886620358));
#44118=CARTESIAN_POINT('Ctrl Pts',(-40.8768310261112,51.986861668354,0.960744330378307));
#44119=CARTESIAN_POINT('Ctrl Pts',(-40.8177064113942,51.5038570687547,0.960726074192245));
#44120=CARTESIAN_POINT('Ctrl Pts',(-40.9438088155039,51.9944136675709,0.47467159909151));
#44121=CARTESIAN_POINT('Ctrl Pts',(-40.9430436333268,51.9808656960017,0.960744325471528));
#44122=CARTESIAN_POINT('Ctrl Pts',(-40.9157121683823,51.4951103457,0.960726074192309));
#44123=CARTESIAN_POINT('Ctrl Pts',(-40.9765613745278,51.9931067249951,0.474691498565247));
#44124=CARTESIAN_POINT('Ctrl Pts',(-40.9762432211227,51.9795219679182,0.960744324371349));
#44125=CARTESIAN_POINT('Ctrl Pts',(-40.9648416217445,51.4931507434584,0.960726074192323));
#44126=CARTESIAN_POINT('Ctrl Pts',(-41.0093983575033,51.9934156040182,0.474686798057427));
#44127=CARTESIAN_POINT('Ctrl Pts',(-41.0095260061652,51.9798394813421,0.960744324630973));
#44128=CARTESIAN_POINT('Ctrl Pts',(-41.0140977126992,51.4936138694024,0.96072607419232));
#44129=CARTESIAN_POINT('Ctrl Pts',(-39.0000040107747,39.1144560173486,15.9767070126905));
#44130=CARTESIAN_POINT('Ctrl Pts',(-38.997993285275,39.2396510906292,16.4628478279265));
#44131=CARTESIAN_POINT('Ctrl Pts',(-39.5,39.2396510906291,16.4628478279265));
#44132=CARTESIAN_POINT('Ctrl Pts',(-38.9999710932286,39.1281993640875,15.9816539819137));
#44133=CARTESIAN_POINT('Ctrl Pts',(-39.0061770165812,39.2517434266058,16.4597337088979));
#44134=CARTESIAN_POINT('Ctrl Pts',(-39.4999999961727,39.2572581017962,16.4583135222598));
#44135=CARTESIAN_POINT('Ctrl Pts',(-38.9999389637471,39.1421528140174,15.9865420342591));
#44136=CARTESIAN_POINT('Ctrl Pts',(-39.014035614548,39.2643832154332,16.4564671712221));
#44137=CARTESIAN_POINT('Ctrl Pts',(-39.499705301717,39.2748828882628,16.4537445183042));
#44138=CARTESIAN_POINT('Ctrl Pts',(-38.9998764799205,39.1704877658621,15.9961825392357));
#44139=CARTESIAN_POINT('Ctrl Pts',(-39.0289560950027,39.2904676116262,16.449694614346));
#44140=CARTESIAN_POINT('Ctrl Pts',(-39.4985567623278,39.3101653714108,16.4445372951836));
#44141=CARTESIAN_POINT('Ctrl Pts',(-38.9998460867676,39.1848893574197,16.0009413430847));
#44142=CARTESIAN_POINT('Ctrl Pts',(-39.0360421116469,39.3039238546721,16.4461859930947));
#44143=CARTESIAN_POINT('Ctrl Pts',(-39.4977012327184,39.3278472445554,16.4398926700023));
#44144=CARTESIAN_POINT('Ctrl Pts',(-38.9997581301385,39.2285967746172,16.0149383729164));
#44145=CARTESIAN_POINT('Ctrl Pts',(-39.0559248124238,39.344910686845,16.4354437398195));
#44146=CARTESIAN_POINT('Ctrl Pts',(-39.4943483441076,39.3807573812163,16.425903199997));
#44147=CARTESIAN_POINT('Ctrl Pts',(-38.9997039330361,39.2583318414788,16.0238756193564));
#44148=CARTESIAN_POINT('Ctrl Pts',(-39.0677029509203,39.3735823596466,16.4278595602795));
#44149=CARTESIAN_POINT('Ctrl Pts',(-39.4910758730554,39.4157676793138,16.4165250387018));
#44150=CARTESIAN_POINT('Ctrl Pts',(-38.999604938088,39.3190178033854,16.0408596441778));
#44151=CARTESIAN_POINT('Ctrl Pts',(-39.0882518025141,39.4325885301134,16.412067946938));
#44152=CARTESIAN_POINT('Ctrl Pts',(-39.4827310120233,39.4853254063385,16.3976569833155));
#44153=CARTESIAN_POINT('Ctrl Pts',(-38.9995601408619,39.3499685976509,16.0489061580615));
#44154=CARTESIAN_POINT('Ctrl Pts',(-39.0971196495093,39.4629323923524,16.4038627674137));
#44155=CARTESIAN_POINT('Ctrl Pts',(-39.477657772467,39.5198726423859,16.3881671255767));
#44156=CARTESIAN_POINT('Ctrl Pts',(-38.9994801961035,39.4130852578651,16.0639945121934));
#44157=CARTESIAN_POINT('Ctrl Pts',(-39.1121948841364,39.5248397888183,16.3869197775902));
#44158=CARTESIAN_POINT('Ctrl Pts',(-39.4659272469331,39.5885541732129,16.3690696448498));
#44159=CARTESIAN_POINT('Ctrl Pts',(-38.9994450516092,39.4452510448586,16.0710360960569));
#44160=CARTESIAN_POINT('Ctrl Pts',(-39.1184775000691,39.5564256521688,16.378180606244));
#44161=CARTESIAN_POINT('Ctrl Pts',(-39.459269437904,39.6226883492881,16.3594620443941));
#44162=CARTESIAN_POINT('Ctrl Pts',(-38.9993541639804,39.5435429335581,16.0904717711952));
#44163=CARTESIAN_POINT('Ctrl Pts',(-39.1336266951939,39.6515152942701,16.3515497917151));
#44164=CARTESIAN_POINT('Ctrl Pts',(-39.4371887494363,39.7245336577965,16.3304551567704));
#44165=CARTESIAN_POINT('Ctrl Pts',(-38.9993130686179,39.61146453535,16.1011742849298));
#44166=CARTESIAN_POINT('Ctrl Pts',(-39.1394434604447,39.7175866597975,16.3326419457149));
#44167=CARTESIAN_POINT('Ctrl Pts',(-39.4196659843394,39.7916893166733,16.3108717173562));
#44168=CARTESIAN_POINT('Ctrl Pts',(-38.9992682955953,39.7516550808854,16.117053677644));
#44169=CARTESIAN_POINT('Ctrl Pts',(-39.1435098339892,39.8515050401373,16.2933507973697));
#44170=CARTESIAN_POINT('Ctrl Pts',(-39.3801865982225,39.9247885133103,16.2711794528008));
#44171=CARTESIAN_POINT('Ctrl Pts',(-38.9992646285835,39.8239232615503,16.1222252243025));
#44172=CARTESIAN_POINT('Ctrl Pts',(-39.1420289111712,39.9196949489101,16.272899676181));
#44173=CARTESIAN_POINT('Ctrl Pts',(-39.3582250294553,39.9907309434165,16.2510708476132));
#44174=CARTESIAN_POINT('Ctrl Pts',(-38.9992908400457,39.9719736471985,16.1260514269948));
#44175=CARTESIAN_POINT('Ctrl Pts',(-39.1333004854831,40.0568779685301,16.2307569206561));
#44176=CARTESIAN_POINT('Ctrl Pts',(-39.3108390135054,40.1216262610997,16.2102943675883));
#44177=CARTESIAN_POINT('Ctrl Pts',(-38.9993206376677,40.0473915068889,16.1246923030909));
#44178=CARTESIAN_POINT('Ctrl Pts',(-39.1262064141833,40.1259439037555,16.2090697109808));
#44179=CARTESIAN_POINT('Ctrl Pts',(-39.2855296954197,40.1862633392644,16.1897252160385));
#44180=CARTESIAN_POINT('Ctrl Pts',(-38.9994069311823,40.1999218820111,16.1148017033617));
#44181=CARTESIAN_POINT('Ctrl Pts',(-39.1079941481566,40.2637234010117,16.1648101024219));
#44182=CARTESIAN_POINT('Ctrl Pts',(-39.2325813022676,40.3142937443227,16.1481519683413));
#44183=CARTESIAN_POINT('Ctrl Pts',(-38.9994634274222,40.2770321041362,16.1062664623901));
#44184=CARTESIAN_POINT('Ctrl Pts',(-39.0968995045256,40.3328826748058,16.142114510182));
#44185=CARTESIAN_POINT('Ctrl Pts',(-39.2049393098256,40.3776888833517,16.1271472128044));
#44186=CARTESIAN_POINT('Ctrl Pts',(-38.9995951129803,40.4316194825974,16.081643859639));
#44187=CARTESIAN_POINT('Ctrl Pts',(-39.072159950563,40.4706330784677,16.095916469794));
#44188=CARTESIAN_POINT('Ctrl Pts',(-39.1481308710056,40.5035902044287,16.0846171794634));
#44189=CARTESIAN_POINT('Ctrl Pts',(-38.999670291757,40.5090898760604,16.0655543496676));
#44190=CARTESIAN_POINT('Ctrl Pts',(-39.0584715863085,40.5396732906564,16.072276576533));
#44191=CARTESIAN_POINT('Ctrl Pts',(-39.1189633371598,40.5660959131574,16.0630920071615));
#44192=CARTESIAN_POINT('Ctrl Pts',(-38.9997902995226,40.6244575672009,16.0357256794342));
#44193=CARTESIAN_POINT('Ctrl Pts',(-39.0370060054887,40.6428892089116,16.0361908002652));
#44194=CARTESIAN_POINT('Ctrl Pts',(-39.0746438817091,40.6594331070692,16.0303432281553));
#44195=CARTESIAN_POINT('Ctrl Pts',(-38.9998315025215,40.6627730639081,16.024836482104));
#44196=CARTESIAN_POINT('Ctrl Pts',(-39.0296982884772,40.6772372709639,16.0240596836177));
#44197=CARTESIAN_POINT('Ctrl Pts',(-39.0597758040782,40.6904751380211,16.0193500439252));
#44198=CARTESIAN_POINT('Ctrl Pts',(-38.9998942165126,40.7198948523673,16.0071060901951));
#44199=CARTESIAN_POINT('Ctrl Pts',(-39.0186217778953,40.7286878641882,16.0057033726188));
#44200=CARTESIAN_POINT('Ctrl Pts',(-39.0374020341813,40.7369624565466,16.002735157554));
#44201=CARTESIAN_POINT('Ctrl Pts',(-38.9999152726188,40.7388768849487,16.0009633713224));
#44202=CARTESIAN_POINT('Ctrl Pts',(-39.014910542557,40.7458261614915,15.9995581052332));
#44203=CARTESIAN_POINT('Ctrl Pts',(-39.0299321594339,40.7524456017426,15.9971760044345));
#44204=CARTESIAN_POINT('Ctrl Pts',(-38.9999575371806,40.7767006320785,15.9882187582803));
#44205=CARTESIAN_POINT('Ctrl Pts',(-39.0074696557041,40.7800779010963,15.9872148913379));
#44206=CARTESIAN_POINT('Ctrl Pts',(-39.0149802525177,40.7833915593417,15.986014280891));
#44207=CARTESIAN_POINT('Ctrl Pts',(-38.9999787159053,40.7955159485185,15.9816268333025));
#44208=CARTESIAN_POINT('Ctrl Pts',(-39.0037437085471,40.7971742516858,15.9810232603102));
#44209=CARTESIAN_POINT('Ctrl Pts',(-39.0075087112142,40.798832545426,15.9804196907491));
#44210=CARTESIAN_POINT('Ctrl Pts',(-39.,40.8143424311314,15.9747745540155));
#44211=CARTESIAN_POINT('Ctrl Pts',(-39.,40.8143424311314,15.9747745540155));
#44212=CARTESIAN_POINT('Ctrl Pts',(-39.,40.8143424311314,15.9747745540155));
#44213=CARTESIAN_POINT('Origin',(-33.5,53.0946168001448,6.54972098527501E-10));
#44214=CARTESIAN_POINT('Origin',(-39.,34.999999994595,6.54998265276524E-10));
#44215=CARTESIAN_POINT('',(-39.,34.999999994595,-5.04750793782168));
#44216=CARTESIAN_POINT('',(-39.,35.0898188972248,14.8657974082861));
#44217=CARTESIAN_POINT('Origin',(-35.3179607461319,20.7255401693197,-5.04750793782167));
#44218=CARTESIAN_POINT('Origin',(-42.5,34.8957733482214,1.2045349051092));
#44219=CARTESIAN_POINT('Ctrl Pts',(-42.5,25.7126140905746,4.89841434305228));
#44220=CARTESIAN_POINT('Ctrl Pts',(-42.4544360876625,25.7126140905746,4.89841434305228));
#44221=CARTESIAN_POINT('Ctrl Pts',(-42.4099205589807,25.7211751731272,4.90131450985059));
#44222=CARTESIAN_POINT('Ctrl Pts',(-42.3189430447185,25.7556046238125,4.91292843604643));
#44223=CARTESIAN_POINT('Ctrl Pts',(-42.2748783192192,25.7831784389946,4.92220957382935));
#44224=CARTESIAN_POINT('Ctrl Pts',(-42.1833702395799,25.8618864121522,4.94850465259141));
#44225=CARTESIAN_POINT('Ctrl Pts',(-42.1405089721587,25.9175895123965,4.96697887534569));
#44226=CARTESIAN_POINT('Ctrl Pts',(-42.0712695189332,26.0405218463918,5.00723555150006));
#44227=CARTESIAN_POINT('Ctrl Pts',(-42.0453333388046,26.1092745195586,5.0294917844871));
#44228=CARTESIAN_POINT('Ctrl Pts',(-42.009448637647,26.2541174515733,5.07570493574361));
#44229=CARTESIAN_POINT('Ctrl Pts',(-42.0003510591406,26.3317096755902,5.10009922095507));
#44230=CARTESIAN_POINT('Ctrl Pts',(-42.0000033224979,26.4103312392474,5.12442130473777));
#44231=CARTESIAN_POINT('Ctrl Pts',(-42.,26.4118341518126,5.12488609601442));
#44232=CARTESIAN_POINT('Ctrl Pts',(-42.,26.4133371006572,5.12535075410316));
#44233=CARTESIAN_POINT('Ctrl Pts',(-42.5,29.807193045783,3.00578708432712));
#44234=CARTESIAN_POINT('Ctrl Pts',(-42.4826491826238,29.807193045783,3.00578708432712));
#44235=CARTESIAN_POINT('Ctrl Pts',(-42.4652566053828,29.8068240402059,3.00695243590386));
#44236=CARTESIAN_POINT('Ctrl Pts',(-42.3984104029602,29.8039651162076,3.01599095899508));
#44237=CARTESIAN_POINT('Ctrl Pts',(-42.3512786216694,29.7989069718977,3.03197933804397));
#44238=CARTESIAN_POINT('Ctrl Pts',(-42.2553373204745,29.7827689996808,3.08348287759294));
#44239=CARTESIAN_POINT('Ctrl Pts',(-42.2093703460395,29.7709244144044,3.12153688374801));
#44240=CARTESIAN_POINT('Ctrl Pts',(-42.1185333929893,29.7396094754438,3.2237433121557));
#44241=CARTESIAN_POINT('Ctrl Pts',(-42.0788703599454,29.7189044820864,3.29243451923833));
#44242=CARTESIAN_POINT('Ctrl Pts',(-42.0174426176904,29.6718912445443,3.45220337209255));
#44243=CARTESIAN_POINT('Ctrl Pts',(-42.0004779950666,29.6448701695635,3.5464777915612));
#44244=CARTESIAN_POINT('Ctrl Pts',(-42.0000033202246,29.6183969280026,3.64156592368197));
#44245=CARTESIAN_POINT('Ctrl Pts',(-42.,29.6180268093032,3.64289586884436));
#44246=CARTESIAN_POINT('Ctrl Pts',(-42.,29.6176568283776,3.64422585000526));
#44247=CARTESIAN_POINT('Origin',(-42.5,34.2321258407597,0.960461174773771));
#44248=CARTESIAN_POINT('Ctrl Pts',(-42.,38.1717829354129,9.48365926152771));
#44249=CARTESIAN_POINT('Ctrl Pts',(-42.,38.1732312920561,9.48428452066275));
#44250=CARTESIAN_POINT('Ctrl Pts',(-42.0000033223958,38.1746797081854,9.48490965401909));
#44251=CARTESIAN_POINT('Ctrl Pts',(-42.0003519017721,38.2506410915851,9.51768648885896));
#44252=CARTESIAN_POINT('Ctrl Pts',(-42.0094939504563,38.3258766921555,9.54973837417019));
#44253=CARTESIAN_POINT('Ctrl Pts',(-42.0455618257965,38.466697942878,9.60902145670787));
#44254=CARTESIAN_POINT('Ctrl Pts',(-42.0716251146577,38.5337398417288,9.63690992139051));
#44255=CARTESIAN_POINT('Ctrl Pts',(-42.1410737799586,38.6535794559786,9.68628167508754));
#44256=CARTESIAN_POINT('Ctrl Pts',(-42.1839363914962,38.7079106249327,9.70842519372085));
#44257=CARTESIAN_POINT('Ctrl Pts',(-42.2753727862073,38.7847364479714,9.73954067383277));
#44258=CARTESIAN_POINT('Ctrl Pts',(-42.3193584730603,38.8116785080646,9.75038190390326));
#44259=CARTESIAN_POINT('Ctrl Pts',(-42.4101445564636,38.8453212413905,9.76389368020581));
#44260=CARTESIAN_POINT('Ctrl Pts',(-42.4545481243919,38.8536933372283,9.7672436047095));
#44261=CARTESIAN_POINT('Ctrl Pts',(-42.5,38.8536933372283,9.7672436047095));
#44262=CARTESIAN_POINT('Ctrl Pts',(-42.,36.6893998635448,6.27661756768842));
#44263=CARTESIAN_POINT('Ctrl Pts',(-42.,36.6899827586311,6.27537117437134));
#44264=CARTESIAN_POINT('Ctrl Pts',(-42.0000033204919,36.6905655271129,6.27412471941368));
#44265=CARTESIAN_POINT('Ctrl Pts',(-42.0004662363704,36.731188818525,6.18721435730615));
#44266=CARTESIAN_POINT('Ctrl Pts',(-42.0165992209749,36.7708781213347,6.10065128632007));
#44267=CARTESIAN_POINT('Ctrl Pts',(-42.0758441660175,36.8385492890082,5.95035856080122));
#44268=CARTESIAN_POINT('Ctrl Pts',(-42.1151456113166,36.8678277552101,5.88417276489002));
#44269=CARTESIAN_POINT('Ctrl Pts',(-42.2056695167071,36.911145913672,5.78502383058571));
#44270=CARTESIAN_POINT('Ctrl Pts',(-42.2516602512676,36.9271867915193,5.74785640724485));
#44271=CARTESIAN_POINT('Ctrl Pts',(-42.3477951889101,36.948899442058,5.69727843691421));
#44272=CARTESIAN_POINT('Ctrl Pts',(-42.3950686181708,36.9556558410848,5.68141836584189));
#44273=CARTESIAN_POINT('Ctrl Pts',(-42.4631644468274,36.959654908806,5.67203138674556));
#44274=CARTESIAN_POINT('Ctrl Pts',(-42.4816022135789,36.9601910749969,5.67077163494895));
#44275=CARTESIAN_POINT('Ctrl Pts',(-42.5,36.9601910749969,5.67077163494895));
#44276=CARTESIAN_POINT('Ctrl Pts',(-39.5,42.3343534352396,15.3364682905744));
#44277=CARTESIAN_POINT('Ctrl Pts',(-38.9979932851518,42.3343534352396,15.3364682905744));
#44278=CARTESIAN_POINT('Ctrl Pts',(-39.0000040107752,42.1177731327825,14.8835889784804));
#44279=CARTESIAN_POINT('Ctrl Pts',(-39.4999999961727,42.3179510866741,15.3443123795369));
#44280=CARTESIAN_POINT('Ctrl Pts',(-39.006177016461,42.323088451335,15.3418555407348));
#44281=CARTESIAN_POINT('Ctrl Pts',(-38.9999710932271,42.110424968906,14.8962126297643));
#44282=CARTESIAN_POINT('Ctrl Pts',(-39.499705301717,42.3015128178088,15.3521413138102));
#44283=CARTESIAN_POINT('Ctrl Pts',(-39.0140356144307,42.3113061213981,15.3474779273468));
#44284=CARTESIAN_POINT('Ctrl Pts',(-38.9999389637436,42.1028779856087,14.9089261998295));
#44285=CARTESIAN_POINT('Ctrl Pts',(-39.4985567623277,42.2685665787124,15.3677673147087));
#44286=CARTESIAN_POINT('Ctrl Pts',(-39.0289560948911,42.2869709989985,15.3590565744642));
#44287=CARTESIAN_POINT('Ctrl Pts',(-38.9998764799132,42.0873689503535,14.9345246110643));
#44288=CARTESIAN_POINT('Ctrl Pts',(-39.4977012327184,42.252035970528,15.3755750143715));
#44289=CARTESIAN_POINT('Ctrl Pts',(-39.036042111538,42.2744076205215,15.365018320954));
#44290=CARTESIAN_POINT('Ctrl Pts',(-38.9998460867584,42.0793955913205,14.9474272309225));
#44291=CARTESIAN_POINT('Ctrl Pts',(-39.4943483441076,42.2025121963684,15.3988684388844));
#44292=CARTESIAN_POINT('Ctrl Pts',(-39.0559248123225,42.2361048981911,15.3831351054061));
#44293=CARTESIAN_POINT('Ctrl Pts',(-38.9997581301239,42.054910884604,14.9862441640743));
#44294=CARTESIAN_POINT('Ctrl Pts',(-39.4910758730554,42.1696645861769,15.4141885363659));
#44295=CARTESIAN_POINT('Ctrl Pts',(-39.0677029508239,42.2092661059301,15.3957550828391));
#44296=CARTESIAN_POINT('Ctrl Pts',(-38.9997039330181,42.0378772531472,15.0122038246002));
#44297=CARTESIAN_POINT('Ctrl Pts',(-39.4827310120233,42.1042521236924,15.4444456124742));
#44298=CARTESIAN_POINT('Ctrl Pts',(-39.0882518024267,42.1539141035433,15.4215864404609));
#44299=CARTESIAN_POINT('Ctrl Pts',(-38.9996049380639,42.0023062299753,15.0642225268363));
#44300=CARTESIAN_POINT('Ctrl Pts',(-39.4776577724669,42.071687442521,15.4593824949676));
#44301=CARTESIAN_POINT('Ctrl Pts',(-39.097119649426,42.1253951687597,15.4348055669586));
#44302=CARTESIAN_POINT('Ctrl Pts',(-38.9995601408351,41.9837687454459,15.0902813011494));
#44303=CARTESIAN_POINT('Ctrl Pts',(-39.4659272469331,42.0067987134986,15.4889006130091));
#44304=CARTESIAN_POINT('Ctrl Pts',(-39.1121948840609,42.0670806077806,15.4616197911504));
#44305=CARTESIAN_POINT('Ctrl Pts',(-38.9994801960717,41.9451171857117,15.1424102581432));
#44306=CARTESIAN_POINT('Ctrl Pts',(-39.4592694379039,41.9744747710641,15.5034817895162));
#44307=CARTESIAN_POINT('Ctrl Pts',(-39.1184774999971,42.0372670016198,15.4752281991058));
#44308=CARTESIAN_POINT('Ctrl Pts',(-38.9994450515753,41.9250030061892,15.1684801936704));
#44309=CARTESIAN_POINT('Ctrl Pts',(-39.4371887494363,41.8778114704634,15.5467261268538));
#44310=CARTESIAN_POINT('Ctrl Pts',(-39.1336266951318,41.947306152076,15.5159502553722));
#44311=CARTESIAN_POINT('Ctrl Pts',(-38.9993541639409,41.862200062219,15.2465495928052));
#44312=CARTESIAN_POINT('Ctrl Pts',(-39.4196659843393,41.8137792589468,15.5748911673596));
#44313=CARTESIAN_POINT('Ctrl Pts',(-39.1394434603886,41.8845388205298,15.5439358601282));
#44314=CARTESIAN_POINT('Ctrl Pts',(-38.9993130685758,41.8170485398245,15.2984073580465));
#44315=CARTESIAN_POINT('Ctrl Pts',(-39.3801865982225,41.6863056631219,15.63003964312));
#44316=CARTESIAN_POINT('Ctrl Pts',(-39.1435098339433,41.7566955261113,15.5999181698673));
#44317=CARTESIAN_POINT('Ctrl Pts',(-38.9992682955504,41.7198634283339,15.4006844242726));
#44318=CARTESIAN_POINT('Ctrl Pts',(-39.3582250294554,41.6228652687111,15.6570225348818));
#44319=CARTESIAN_POINT('Ctrl Pts',(-39.1420289111301,41.6913132981144,15.6280833305903));
#44320=CARTESIAN_POINT('Ctrl Pts',(-38.9992646285384,41.6678269962403,15.4510991499646));
#44321=CARTESIAN_POINT('Ctrl Pts',(-39.3108390135053,41.496383021843,15.7099238273215));
#44322=CARTESIAN_POINT('Ctrl Pts',(-39.1333004854501,41.5591361671536,15.6839796521741));
#44323=CARTESIAN_POINT('Ctrl Pts',(-38.9992908400022,41.5568732567025,15.5491951447912));
#44324=CARTESIAN_POINT('Ctrl Pts',(-39.2855296954198,41.4336465515375,15.7357148560477));
#44325=CARTESIAN_POINT('Ctrl Pts',(-39.1262064141541,41.4922883215965,15.7117610131304));
#44326=CARTESIAN_POINT('Ctrl Pts',(-38.999320637626,41.4982261963719,15.5966316612412));
#44327=CARTESIAN_POINT('Ctrl Pts',(-39.2325813022674,41.3088468026781,15.7861642587015));
#44328=CARTESIAN_POINT('Ctrl Pts',(-39.1079941481342,41.3582935753545,15.7664191396453));
#44329=CARTESIAN_POINT('Ctrl Pts',(-38.9994069311459,41.3750235951481,15.6870996575201));
#44330=CARTESIAN_POINT('Ctrl Pts',(-39.2049393098254,41.2467817121011,15.8108232923254));
#44331=CARTESIAN_POINT('Ctrl Pts',(-39.0968995045062,41.2907260524874,15.7934880316164));
#44332=CARTESIAN_POINT('Ctrl Pts',(-38.9994634273892,41.3104673908405,15.7301267789704));
#44333=CARTESIAN_POINT('Ctrl Pts',(-39.1481308710058,41.1229979262366,15.8591712058507));
#44334=CARTESIAN_POINT('Ctrl Pts',(-39.0721599505498,41.1555075932688,15.846642532199));
#44335=CARTESIAN_POINT('Ctrl Pts',(-38.9995951129554,41.1762194846274,15.8106316224558));
#44336=CARTESIAN_POINT('Ctrl Pts',(-39.1189633371598,41.0612796613498,15.8828598623271));
#44337=CARTESIAN_POINT('Ctrl Pts',(-39.058471586298,41.0874242918864,15.872911516296));
#44338=CARTESIAN_POINT('Ctrl Pts',(-38.9996702917367,41.1065315825528,15.848103351789));
#44339=CARTESIAN_POINT('Ctrl Pts',(-39.0746438817091,40.9687287132405,15.9177688339196));
#44340=CARTESIAN_POINT('Ctrl Pts',(-39.0370060054821,40.9851608213935,15.9116141212873));
#44341=CARTESIAN_POINT('Ctrl Pts',(-38.9997902995097,40.9989813041981,15.8994101871385));
#44342=CARTESIAN_POINT('Ctrl Pts',(-39.0597758040783,40.9378828553123,15.9293009991034));
#44343=CARTESIAN_POINT('Ctrl Pts',(-39.0296982884719,40.9510509478529,15.924399655495));
#44344=CARTESIAN_POINT('Ctrl Pts',(-38.9998315025111,40.9626304897362,15.9156973045773));
#44345=CARTESIAN_POINT('Ctrl Pts',(-39.0374020341813,40.8915916601846,15.9464547300814));
#44346=CARTESIAN_POINT('Ctrl Pts',(-39.018621777892,40.8998382975478,15.9434097092941));
#44347=CARTESIAN_POINT('Ctrl Pts',(-38.9998942165061,40.9074757848707,15.9388322142473));
#44348=CARTESIAN_POINT('Ctrl Pts',(-39.0299321594335,40.8761575280997,15.9521485456168));
#44349=CARTESIAN_POINT('Ctrl Pts',(-39.0149105425542,40.8827594984001,15.9497184465192));
#44350=CARTESIAN_POINT('Ctrl Pts',(-38.9999152726136,40.8889862407112,15.9463280339396));
#44351=CARTESIAN_POINT('Ctrl Pts',(-39.014980252518,40.8452769316474,15.9634898474352));
#44352=CARTESIAN_POINT('Ctrl Pts',(-39.0074696557029,40.8485870786527,15.9622795899339));
#44353=CARTESIAN_POINT('Ctrl Pts',(-38.999957537178,40.8518194900493,15.9608777299468));
#44354=CARTESIAN_POINT('Ctrl Pts',(-39.0075087112135,40.829852316837,15.9691294172817));
#44355=CARTESIAN_POINT('Ctrl Pts',(-39.0037437085461,40.8315106105773,15.9685258477206));
#44356=CARTESIAN_POINT('Ctrl Pts',(-38.999978715904,40.8331689137449,15.9679222747282));
#44357=CARTESIAN_POINT('Ctrl Pts',(-39.,40.8143424311314,15.9747745540155));
#44358=CARTESIAN_POINT('Ctrl Pts',(-39.,40.8143424311314,15.9747745540155));
#44359=CARTESIAN_POINT('Ctrl Pts',(-39.,40.8143424311314,15.9747745540155));
#44360=CARTESIAN_POINT('Origin',(-42.5,34.999999994595,6.55E-10));
#44361=CARTESIAN_POINT('Origin',(-42.5,34.999999994595,6.55E-10));
#44362=CARTESIAN_POINT('Origin',(-42.5,34.999999994595,6.55E-10));
#44363=CARTESIAN_POINT('Ctrl Pts',(-42.,25.0606841227656,1.100000000655));
#44364=CARTESIAN_POINT('Ctrl Pts',(-42.,25.0595088693021,1.09894763890697));
#44365=CARTESIAN_POINT('Ctrl Pts',(-42.0000033223958,25.058333705052,1.09789517038892));
#44366=CARTESIAN_POINT('Ctrl Pts',(-42.0003519017721,24.99671007141,1.04269570981911));
#44367=CARTESIAN_POINT('Ctrl Pts',(-42.0094939504564,24.9360490092969,0.987850887928174));
#44368=CARTESIAN_POINT('Ctrl Pts',(-42.0455618257965,24.8231515921703,0.884898074774389));
#44369=CARTESIAN_POINT('Ctrl Pts',(-42.0716251146577,24.7697076177618,0.835743987830459));
#44370=CARTESIAN_POINT('Ctrl Pts',(-42.1410737799586,24.6746102687835,0.747678118028473));
#44371=CARTESIAN_POINT('Ctrl Pts',(-42.1839363914962,24.6317141928668,0.707651401846346));
#44372=CARTESIAN_POINT('Ctrl Pts',(-42.2753727862072,24.5712359099918,0.650970210180581));
#44373=CARTESIAN_POINT('Ctrl Pts',(-42.3193584730602,24.550090913296,0.631063025893261));
#44374=CARTESIAN_POINT('Ctrl Pts',(-42.4101445564636,24.5237103782914,0.606193989374706));
#44375=CARTESIAN_POINT('Ctrl Pts',(-42.4545481243919,24.5171568688013,0.60000000065501));
#44376=CARTESIAN_POINT('Ctrl Pts',(-42.5,24.5171568688013,0.60000000065501));
#44377=CARTESIAN_POINT('Ctrl Pts',(-42.5,25.2143573355172,3.80673058592581));
#44378=CARTESIAN_POINT('Ctrl Pts',(-42.4546604723592,25.2143573355172,3.80673058592581));
#44379=CARTESIAN_POINT('Ctrl Pts',(-42.410369154297,25.2177192828128,3.79838660971661));
#44380=CARTESIAN_POINT('Ctrl Pts',(-42.3197752645317,25.2312813982443,3.76485163764536));
#44381=CARTESIAN_POINT('Ctrl Pts',(-42.2758690263218,25.2421675242903,3.73798453911452));
#44382=CARTESIAN_POINT('Ctrl Pts',(-42.184505343157,25.2734307410951,3.66132378610309));
#44383=CARTESIAN_POINT('Ctrl Pts',(-42.141641846796,25.2956984958726,3.60706178152292));
#44384=CARTESIAN_POINT('Ctrl Pts',(-42.0719829628829,25.345457581468,3.48710459800191));
#44385=CARTESIAN_POINT('Ctrl Pts',(-42.0457917884805,25.3736439183274,3.41980920565272));
#44386=CARTESIAN_POINT('Ctrl Pts',(-42.0095395323332,25.4335707666125,3.27843423840761));
#44387=CARTESIAN_POINT('Ctrl Pts',(-42.0003527473331,25.4659862397681,3.20286907923119));
#44388=CARTESIAN_POINT('Ctrl Pts',(-42.0000033222927,25.4991296293867,3.126589852694));
#44389=CARTESIAN_POINT('Ctrl Pts',(-42.,25.4997602061239,3.12513893728405));
#44390=CARTESIAN_POINT('Ctrl Pts',(-42.,25.5003909094963,3.12368808212368));
#44391=CARTESIAN_POINT('Origin',(-42.5,31.9421285471778,0.146139381756428));
#44392=CARTESIAN_POINT('Origin',(-42.5,24.5171568688013,1.100000000655));
#44393=CARTESIAN_POINT('Origin',(-42.5,34.999999994595,6.55E-10));
#44394=CARTESIAN_POINT('Ctrl Pts',(-42.,28.5937530433762,-1.099999999345));
#44395=CARTESIAN_POINT('Ctrl Pts',(-42.,28.5946398535677,-1.09894793914394));
#44396=CARTESIAN_POINT('Ctrl Pts',(-42.0000033204919,28.5955267728317,-1.09789596800162));
#44397=CARTESIAN_POINT('Ctrl Pts',(-42.0004662363704,28.6573726864841,-1.02455603473682));
#44398=CARTESIAN_POINT('Ctrl Pts',(-42.0165992209748,28.7192952337358,-0.952209617009781));
#44399=CARTESIAN_POINT('Ctrl Pts',(-42.0758441660175,28.8273260851525,-0.827724174405475));
#44400=CARTESIAN_POINT('Ctrl Pts',(-42.1151456113167,28.8751198610887,-0.773377664441317));
#44401=CARTESIAN_POINT('Ctrl Pts',(-42.2056695167071,28.9469442910977,-0.692456559159142));
#44402=CARTESIAN_POINT('Ctrl Pts',(-42.2516602512676,28.9739516189116,-0.662301437467018));
#44403=CARTESIAN_POINT('Ctrl Pts',(-42.3477951889101,29.0107522579474,-0.621371213393126));
#44404=CARTESIAN_POINT('Ctrl Pts',(-42.3950686181708,29.0223139734333,-0.608583816580183));
#44405=CARTESIAN_POINT('Ctrl Pts',(-42.4631644468274,29.029156829769,-0.601015247603024));
#44406=CARTESIAN_POINT('Ctrl Pts',(-42.4816022135789,29.0300753719553,-0.599999999345001));
#44407=CARTESIAN_POINT('Ctrl Pts',(-42.5,29.0300753719553,-0.599999999345001));
#44408=CARTESIAN_POINT('Origin',(-42.5,24.5171568688013,-1.099999999345));
#44409=CARTESIAN_POINT('Ctrl Pts',(-42.4999999999992,21.3792341097314,-0.599999999345));
#44410=CARTESIAN_POINT('Ctrl Pts',(-42.4490140835651,21.3497688309388,-0.599999999345));
#44411=CARTESIAN_POINT('Ctrl Pts',(-42.4007729318771,21.3161690037742,-0.607751395428307));
#44412=CARTESIAN_POINT('Ctrl Pts',(-42.285433335349,21.2206234281771,-0.642356903987189));
#44413=CARTESIAN_POINT('Ctrl Pts',(-42.2250431349784,21.154461459802,-0.677422925574331));
#44414=CARTESIAN_POINT('Ctrl Pts',(-42.1177385329819,21.0028381404881,-0.76878542539937));
#44415=CARTESIAN_POINT('Ctrl Pts',(-42.0745545865654,20.9152860451152,-0.828340175668635));
#44416=CARTESIAN_POINT('Ctrl Pts',(-42.0155723848691,20.7344912244631,-0.956764117541972));
#44417=CARTESIAN_POINT('Ctrl Pts',(-42.0004519323175,20.6399172853836,-1.02689744515237));
#44418=CARTESIAN_POINT('Ctrl Pts',(-42.0000033273437,20.5446114752944,-1.09789375193343));
#44419=CARTESIAN_POINT('Ctrl Pts',(-42.,20.5431978887484,-1.09894685426265));
#44420=CARTESIAN_POINT('Ctrl Pts',(-42.,20.5417843370527,-1.099999999345));
#44421=CARTESIAN_POINT('Origin',(-35.8316689588642,34.999999994595,6.55E-10));
#44422=CARTESIAN_POINT('Origin',(-43.,34.999999994595,6.55E-10));
#44423=CARTESIAN_POINT('Origin',(-43.,34.999999994595,6.55E-10));
#44424=CARTESIAN_POINT('Origin',(-44.,47.8027400910494,-6.80733765974042));
#44425=CARTESIAN_POINT('Origin',(-42.5,39.7882820011544,13.1556966916577));
#44426=CARTESIAN_POINT('',(-34.,37.4390504491896,14.0107470499719));
#44427=CARTESIAN_POINT('',(-34.,37.4390504491896,14.0107470499719));
#44428=CARTESIAN_POINT('',(-39.,35.0898188972248,14.8657974082861));
#44429=CARTESIAN_POINT('Origin',(-34.,38.5965482096145,9.88143500940095));
#44430=CARTESIAN_POINT('',(-34.,37.7810705925152,14.9504396707578));
#44431=CARTESIAN_POINT('Origin',(-39.,35.4318390405505,15.805490029072));
#44432=CARTESIAN_POINT('Origin',(-30.8535533905933,49.0946168001447,-5.39282731604877));
#44433=CARTESIAN_POINT('Origin',(-46.,34.999999994595,6.54998265276524E-10));
#44434=CARTESIAN_POINT('Origin',(-46.,34.999999994595,6.54998265276524E-10));
#44435=CARTESIAN_POINT('Origin',(-31.,34.999999994595,6.54998265276524E-10));
#62952=UNCERTAINTY_MEASURE_WITH_UNIT(LENGTH_MEASURE(0.01),#62975,
'DISTANCE_ACCURACY_VALUE',
'Maximum model space distance between geometric entities at asserted c
onnectivities');
#62960=UNCERTAINTY_MEASURE_WITH_UNIT(LENGTH_MEASURE(0.01),#62975,
'DISTANCE_ACCURACY_VALUE',
'Maximum model space distance between geometric entities at asserted c
onnectivities');
#62966=(
GEOMETRIC_REPRESENTATION_CONTEXT(3)
GLOBAL_UNCERTAINTY_ASSIGNED_CONTEXT((#62952))
GLOBAL_UNIT_ASSIGNED_CONTEXT((#62975,#62977,#62978))
REPRESENTATION_CONTEXT('','3D')
);
#62974=(
GEOMETRIC_REPRESENTATION_CONTEXT(3)
GLOBAL_UNCERTAINTY_ASSIGNED_CONTEXT((#62960))
GLOBAL_UNIT_ASSIGNED_CONTEXT((#62975,#62977,#62978))
REPRESENTATION_CONTEXT('','3D')
);
#62975=(
LENGTH_UNIT()
NAMED_UNIT(*)
SI_UNIT(.MILLI.,.METRE.)
);
#62977=(
NAMED_UNIT(*)
PLANE_ANGLE_UNIT()
SI_UNIT($,.RADIAN.)
);
#62978=(
NAMED_UNIT(*)
SI_UNIT($,.STERADIAN.)
SOLID_ANGLE_UNIT()
);
#62984=SHAPE_DEFINITION_REPRESENTATION(#62997,#63025);
#62997=PRODUCT_DEFINITION_SHAPE('',$,#63039);
#63025=SHAPE_REPRESENTATION('',(#15858),#62966);
#63033=PRODUCT_DEFINITION_CONTEXT('part definition',#63074,'design');
#63039=PRODUCT_DEFINITION('Throttle Actuation Mechanism Spring',
'Throttle Actuation Mechanism Spring',#63052,#63033);
#63052=PRODUCT_DEFINITION_FORMATION('',$,#63081);
#63074=APPLICATION_CONTEXT(
'Core Data for Automotive Mechanical Design Process');
#63075=PRODUCT_CONTEXT('part definition',#63074,'mechanical');
#63081=PRODUCT('Throttle Actuation Mechanism Spring',
'Throttle Actuation Mechanism Spring',$,(#63075));
#63090=PRESENTATION_STYLE_ASSIGNMENT((#63092));
#63092=SURFACE_STYLE_USAGE(.BOTH.,#63094);
#63094=SURFACE_SIDE_STYLE('',(#63096));
#63096=SURFACE_STYLE_FILL_AREA(#63098);
#63098=FILL_AREA_STYLE('Opaque(202,209,238)',(#63100));
#63100=FILL_AREA_STYLE_COLOUR('Opaque(202,209,238)',#63102);
#63102=COLOUR_RGB('Opaque(202,209,238)', 0.66274510, 0.83137255, 0.94901961);
ENDSEC;
END-ISO-10303-21;
